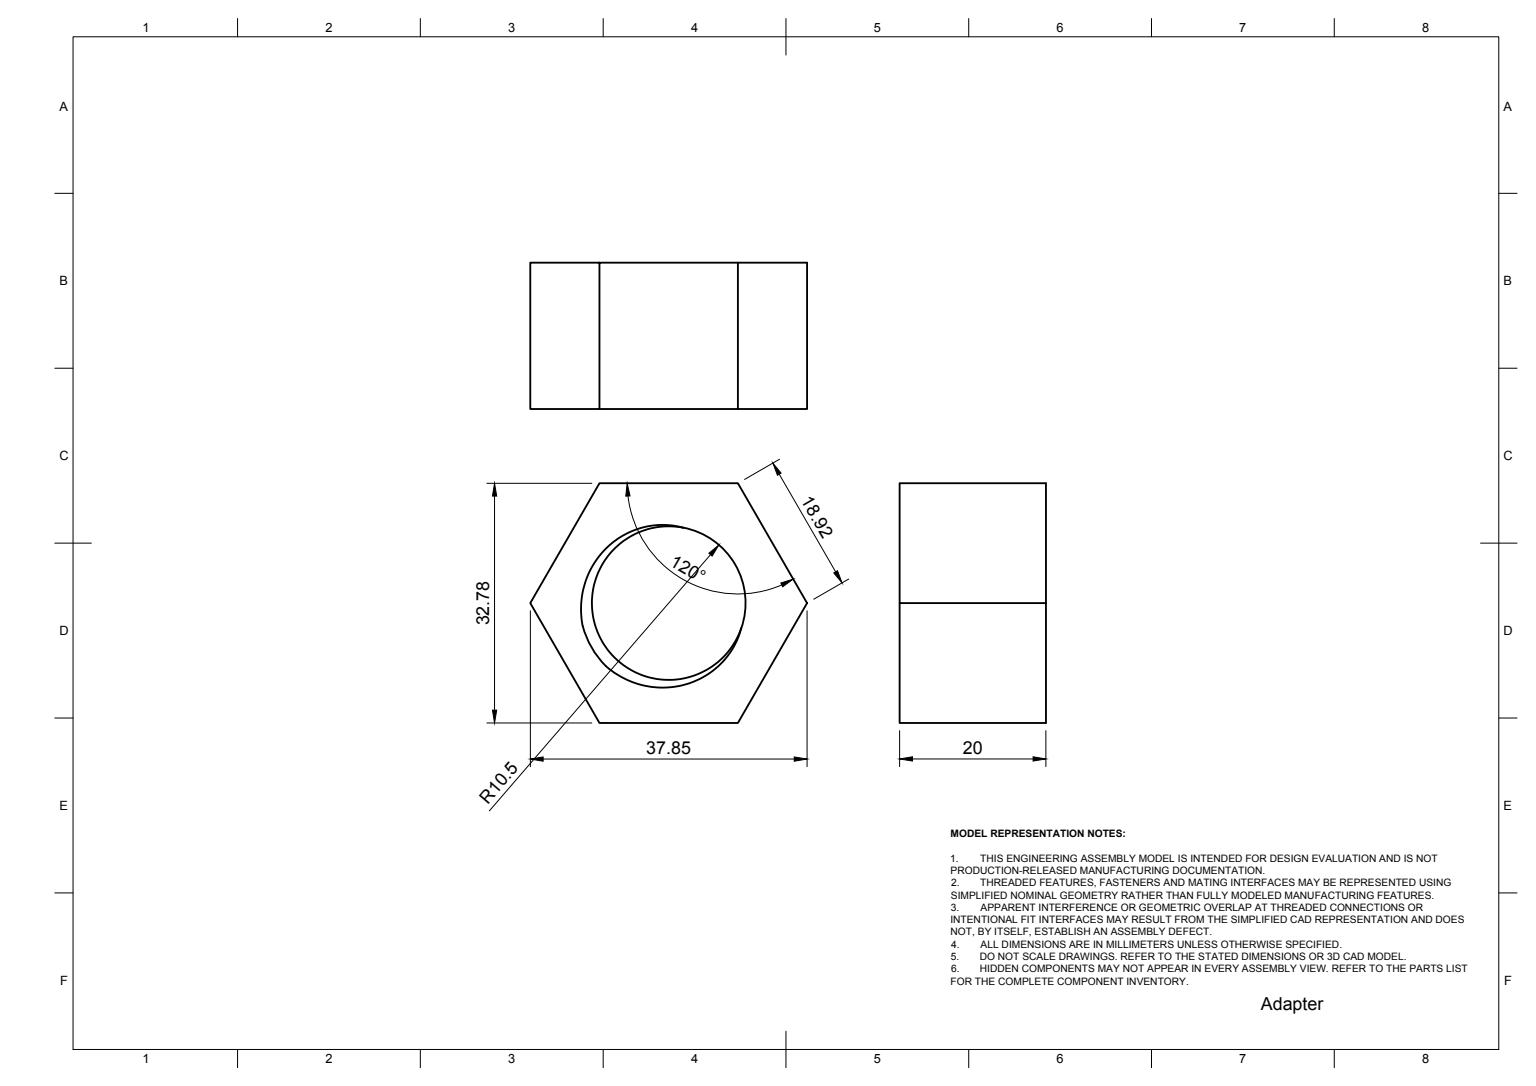
ISO-10303-21;
HEADER;
/* Generated by software containing ST-Developer
 * from STEP Tools, Inc. (www.steptools.com) 
 */

FILE_DESCRIPTION(
/* description */ (''),
/* implementation_level */ '2;1');

FILE_NAME(
/* name */ 'Adapter.step',
/* time_stamp */ '2026-10-06T12:47:13-07:00',
/* author */ (''),
/* organization */ (''),
/* preprocessor_version */ 'ST-DEVELOPER v20.2',
/* originating_system */ 'Autodesk Translation Framework v15.15.0.0',
/* authorisation */ '');

FILE_SCHEMA (('AUTOMOTIVE_DESIGN { 1 0 10303 214 3 1 1 }'));
ENDSEC;

DATA;
#10=MECHANICAL_DESIGN_GEOMETRIC_PRESENTATION_REPRESENTATION('',(#70),#42667);
#52=SHAPE_REPRESENTATION_RELATIONSHIP('SRR','None',#42705,#61);
#61=ADVANCED_BREP_SHAPE_REPRESENTATION('',(#79),#42661);
#70=STYLED_ITEM('',(#42756),#79);
#79=MANIFOLD_SOLID_BREP('Body1',#4035);
#86=B_SPLINE_SURFACE_WITH_KNOTS('',3,3,((#10429,#10430,#10431,#10432,#10433,
#10434,#10435,#10436,#10437,#10438,#10439,#10440,#10441,#10442,#10443,#10444,
#10445,#10446,#10447,#10448,#10449,#10450,#10451,#10452,#10453,#10454,#10455,
#10456,#10457,#10458,#10459,#10460,#10461,#10462,#10463,#10464,#10465,#10466,
#10467,#10468,#10469,#10470,#10471,#10472,#10473,#10474,#10475,#10476,#10477,
#10478,#10479,#10480,#10481,#10482,#10483,#10484,#10485,#10486,#10487,#10488,
#10489,#10490,#10491,#10492,#10493,#10494,#10495,#10496,#10497,#10498,#10499,
#10500,#10501,#10502,#10503,#10504,#10505,#10506,#10507,#10508,#10509,#10510,
#10511,#10512,#10513,#10514,#10515,#10516,#10517,#10518,#10519),(#10520,
#10521,#10522,#10523,#10524,#10525,#10526,#10527,#10528,#10529,#10530,#10531,
#10532,#10533,#10534,#10535,#10536,#10537,#10538,#10539,#10540,#10541,#10542,
#10543,#10544,#10545,#10546,#10547,#10548,#10549,#10550,#10551,#10552,#10553,
#10554,#10555,#10556,#10557,#10558,#10559,#10560,#10561,#10562,#10563,#10564,
#10565,#10566,#10567,#10568,#10569,#10570,#10571,#10572,#10573,#10574,#10575,
#10576,#10577,#10578,#10579,#10580,#10581,#10582,#10583,#10584,#10585,#10586,
#10587,#10588,#10589,#10590,#10591,#10592,#10593,#10594,#10595,#10596,#10597,
#10598,#10599,#10600,#10601,#10602,#10603,#10604,#10605,#10606,#10607,#10608,
#10609,#10610),(#10611,#10612,#10613,#10614,#10615,#10616,#10617,#10618,
#10619,#10620,#10621,#10622,#10623,#10624,#10625,#10626,#10627,#10628,#10629,
#10630,#10631,#10632,#10633,#10634,#10635,#10636,#10637,#10638,#10639,#10640,
#10641,#10642,#10643,#10644,#10645,#10646,#10647,#10648,#10649,#10650,#10651,
#10652,#10653,#10654,#10655,#10656,#10657,#10658,#10659,#10660,#10661,#10662,
#10663,#10664,#10665,#10666,#10667,#10668,#10669,#10670,#10671,#10672,#10673,
#10674,#10675,#10676,#10677,#10678,#10679,#10680,#10681,#10682,#10683,#10684,
#10685,#10686,#10687,#10688,#10689,#10690,#10691,#10692,#10693,#10694,#10695,
#10696,#10697,#10698,#10699,#10700,#10701),(#10702,#10703,#10704,#10705,
#10706,#10707,#10708,#10709,#10710,#10711,#10712,#10713,#10714,#10715,#10716,
#10717,#10718,#10719,#10720,#10721,#10722,#10723,#10724,#10725,#10726,#10727,
#10728,#10729,#10730,#10731,#10732,#10733,#10734,#10735,#10736,#10737,#10738,
#10739,#10740,#10741,#10742,#10743,#10744,#10745,#10746,#10747,#10748,#10749,
#10750,#10751,#10752,#10753,#10754,#10755,#10756,#10757,#10758,#10759,#10760,
#10761,#10762,#10763,#10764,#10765,#10766,#10767,#10768,#10769,#10770,#10771,
#10772,#10773,#10774,#10775,#10776,#10777,#10778,#10779,#10780,#10781,#10782,
#10783,#10784,#10785,#10786,#10787,#10788,#10789,#10790,#10791,#10792)),
 .UNSPECIFIED.,.F.,.F.,.F.,(4,4),(4,1,1,1,1,1,1,1,1,1,1,1,1,1,1,1,1,1,1,
1,1,1,1,1,1,1,1,1,1,1,1,1,1,1,1,1,1,1,1,1,1,1,1,1,1,1,1,1,1,1,1,1,1,1,1,
1,1,1,1,1,1,1,1,1,1,1,1,1,1,1,1,1,1,1,1,1,1,1,1,1,1,1,1,1,1,1,1,1,4),(-0.000129081019394602,
0.193330292353948),(11.8519068837255,12.3510302549558,12.8500245451668,
13.3490188353777,13.8480131255886,14.3470074157995,14.8460017060104,15.3449959962214,
15.8439902864323,16.3429845766432,16.8419788668541,17.3409731570651,17.839967447276,
18.3389617374869,18.8379560276978,19.3369503179088,19.8359446081197,20.3349388983306,
20.8339331885415,21.3329274787524,21.8319217689634,22.3309160591743,22.8299103493852,
23.3289046395961,23.8278989298071,24.326893220018,24.8258875102289,25.3248818004398,
25.8238760906508,26.3228703808617,26.8218646710726,27.3208589612835,27.8198532514944,
28.3188475417054,28.8178418319163,29.3168361221272,29.8158304123381,30.3148247025491,
30.81381899276,31.3128132829709,31.8118075731818,32.3108018633928,32.8097961536037,
33.3087904438146,33.8077847340255,34.3067790242364,34.8057733144474,35.3047676046583,
35.8037618948692,36.3027561850801,36.8017504752911,37.300744765502,37.7997390557129,
38.2987333459238,38.7977276361348,39.2967219263457,39.7957162165566,40.2947105067675,
40.7937047969784,41.2926990871894,41.7916933774003,42.2906876676112,42.7896819578221,
43.2886762480331,43.787670538244,44.2866648284549,44.7856591186658,45.2846534088767,
45.7836476990877,46.2826419892986,46.7816362795095,47.2806305697204,47.7796248599314,
48.2786191501423,48.7776134403532,49.2766077305641,49.7756020207751,50.274596310986,
50.7735906011969,51.2725848914078,51.7715791816187,52.2705734718297,52.7695677620406,
53.2685620522515,53.7675563424624,54.2665506326734,54.7655449228843,55.2645392130952,
55.7635335033061),.UNSPECIFIED.);
#87=B_SPLINE_SURFACE_WITH_KNOTS('',3,3,((#11034,#11035,#11036,#11037,#11038,
#11039,#11040,#11041,#11042,#11043,#11044,#11045,#11046,#11047,#11048,#11049,
#11050,#11051,#11052,#11053,#11054,#11055,#11056,#11057,#11058,#11059,#11060,
#11061,#11062,#11063,#11064,#11065,#11066,#11067,#11068,#11069,#11070,#11071,
#11072,#11073,#11074,#11075,#11076,#11077,#11078,#11079,#11080,#11081,#11082,
#11083,#11084,#11085,#11086,#11087,#11088,#11089,#11090,#11091,#11092,#11093,
#11094,#11095,#11096,#11097,#11098,#11099,#11100,#11101,#11102,#11103,#11104,
#11105,#11106,#11107,#11108,#11109,#11110,#11111,#11112,#11113,#11114,#11115,
#11116,#11117,#11118,#11119,#11120,#11121,#11122,#11123,#11124),(#11125,
#11126,#11127,#11128,#11129,#11130,#11131,#11132,#11133,#11134,#11135,#11136,
#11137,#11138,#11139,#11140,#11141,#11142,#11143,#11144,#11145,#11146,#11147,
#11148,#11149,#11150,#11151,#11152,#11153,#11154,#11155,#11156,#11157,#11158,
#11159,#11160,#11161,#11162,#11163,#11164,#11165,#11166,#11167,#11168,#11169,
#11170,#11171,#11172,#11173,#11174,#11175,#11176,#11177,#11178,#11179,#11180,
#11181,#11182,#11183,#11184,#11185,#11186,#11187,#11188,#11189,#11190,#11191,
#11192,#11193,#11194,#11195,#11196,#11197,#11198,#11199,#11200,#11201,#11202,
#11203,#11204,#11205,#11206,#11207,#11208,#11209,#11210,#11211,#11212,#11213,
#11214,#11215),(#11216,#11217,#11218,#11219,#11220,#11221,#11222,#11223,
#11224,#11225,#11226,#11227,#11228,#11229,#11230,#11231,#11232,#11233,#11234,
#11235,#11236,#11237,#11238,#11239,#11240,#11241,#11242,#11243,#11244,#11245,
#11246,#11247,#11248,#11249,#11250,#11251,#11252,#11253,#11254,#11255,#11256,
#11257,#11258,#11259,#11260,#11261,#11262,#11263,#11264,#11265,#11266,#11267,
#11268,#11269,#11270,#11271,#11272,#11273,#11274,#11275,#11276,#11277,#11278,
#11279,#11280,#11281,#11282,#11283,#11284,#11285,#11286,#11287,#11288,#11289,
#11290,#11291,#11292,#11293,#11294,#11295,#11296,#11297,#11298,#11299,#11300,
#11301,#11302,#11303,#11304,#11305,#11306),(#11307,#11308,#11309,#11310,
#11311,#11312,#11313,#11314,#11315,#11316,#11317,#11318,#11319,#11320,#11321,
#11322,#11323,#11324,#11325,#11326,#11327,#11328,#11329,#11330,#11331,#11332,
#11333,#11334,#11335,#11336,#11337,#11338,#11339,#11340,#11341,#11342,#11343,
#11344,#11345,#11346,#11347,#11348,#11349,#11350,#11351,#11352,#11353,#11354,
#11355,#11356,#11357,#11358,#11359,#11360,#11361,#11362,#11363,#11364,#11365,
#11366,#11367,#11368,#11369,#11370,#11371,#11372,#11373,#11374,#11375,#11376,
#11377,#11378,#11379,#11380,#11381,#11382,#11383,#11384,#11385,#11386,#11387,
#11388,#11389,#11390,#11391,#11392,#11393,#11394,#11395,#11396,#11397)),
 .UNSPECIFIED.,.F.,.F.,.F.,(4,4),(4,1,1,1,1,1,1,1,1,1,1,1,1,1,1,1,1,1,1,
1,1,1,1,1,1,1,1,1,1,1,1,1,1,1,1,1,1,1,1,1,1,1,1,1,1,1,1,1,1,1,1,1,1,1,1,
1,1,1,1,1,1,1,1,1,1,1,1,1,1,1,1,1,1,1,1,1,1,1,1,1,1,1,1,1,1,1,1,1,4),(-9.09719654654513E-5,
0.1933682374602),(14.3987024268659,14.8976967170768,15.3966910072877,15.8956852974986,
16.3946795877096,16.8936738779205,17.3926681681314,17.8916624583423,18.3906567485533,
18.8896510387642,19.3886453289751,19.887639619186,20.386633909397,20.8856281996079,
21.3846224898188,21.8836167800297,22.3826110702406,22.8816053604516,23.3805996506625,
23.8795939408734,24.3785882310843,24.8775825212953,25.3765768115062,25.8755711017171,
26.374565391928,26.8735596821389,27.3725539723499,27.8715482625608,28.3705425527717,
28.8695368429826,29.3685311331936,29.8675254234045,30.3665197136154,30.8655140038263,
31.3645082940373,31.8635025842482,32.3624968744591,32.86149116467,33.3604854548809,
33.8594797450919,34.3584740353028,34.8574683255137,35.3564626157246,35.8554569059356,
36.3544511961465,36.8534454863574,37.3524397765683,37.8514340667792,38.3504283569902,
38.8494226472011,39.348416937412,39.8474112276229,40.3464055178339,40.8453998080448,
41.3443940982557,41.8433883884666,42.3423826786776,42.8413769688885,43.3403712590994,
43.8393655493103,44.3383598395212,44.8373541297322,45.3363484199431,45.835342710154,
46.3343370003649,46.8333312905759,47.3323255807868,47.8313198709977,48.3303141612086,
48.8293084514195,49.3283027416305,49.8272970318414,50.3262913220523,50.8252856122632,
51.3242799024742,51.8232741926851,52.322268482896,52.8212627731069,53.3202570633179,
53.8192513535288,54.3182456437397,54.8172399339506,55.3162342241615,55.8152285143725,
56.3142228045834,56.8132170947943,57.3122113850052,57.8112056752162,58.3103290677895),
 .UNSPECIFIED.);
#100=B_SPLINE_CURVE_WITH_KNOTS('',3,(#5957,#5958,#5959,#5960,#5961,#5962,
#5963),.UNSPECIFIED.,.F.,.F.,(4,3,4),(13.8756314554422,13.9455249758043,
14.0061469241355),.UNSPECIFIED.);
#101=B_SPLINE_CURVE_WITH_KNOTS('',3,(#5970,#5971,#5972,#5973,#5974,#5975,
#5976,#5977,#5978,#5979,#5980,#5981,#5982,#5983,#5984,#5985,#5986,#5987,
#5988,#5989,#5990,#5991,#5992,#5993,#5994,#5995,#5996,#5997,#5998,#5999,
#6000,#6001,#6002,#6003,#6004,#6005,#6006,#6007,#6008,#6009,#6010,#6011,
#6012,#6013,#6014,#6015,#6016,#6017,#6018,#6019,#6020,#6021,#6022,#6023,
#6024,#6025,#6026,#6027,#6028,#6029,#6030,#6031,#6032,#6033,#6034,#6035,
#6036,#6037,#6038,#6039,#6040,#6041,#6042,#6043,#6044,#6045,#6046,#6047,
#6048,#6049,#6050,#6051,#6052,#6053,#6054,#6055,#6056,#6057,#6058,#6059,
#6060,#6061,#6062,#6063,#6064,#6065,#6066,#6067,#6068,#6069,#6070,#6071,
#6072,#6073,#6074,#6075,#6076,#6077,#6078,#6079,#6080,#6081,#6082,#6083,
#6084,#6085,#6086,#6087,#6088,#6089,#6090,#6091,#6092,#6093,#6094,#6095,
#6096,#6097,#6098,#6099,#6100,#6101,#6102,#6103,#6104,#6105,#6106,#6107,
#6108,#6109,#6110,#6111,#6112,#6113,#6114,#6115,#6116,#6117,#6118,#6119,
#6120,#6121,#6122,#6123,#6124,#6125,#6126,#6127,#6128,#6129,#6130,#6131,
#6132,#6133,#6134,#6135,#6136,#6137,#6138,#6139,#6140,#6141,#6142,#6143,
#6144,#6145,#6146,#6147,#6148,#6149,#6150,#6151,#6152,#6153,#6154,#6155,
#6156,#6157,#6158,#6159,#6160,#6161,#6162,#6163,#6164,#6165),
 .UNSPECIFIED.,.F.,.F.,(4,3,3,3,3,3,3,3,3,3,3,3,3,3,3,3,3,3,3,3,3,3,3,3,
3,3,3,3,3,3,3,3,3,3,3,3,3,3,3,3,3,3,3,3,3,3,3,3,3,3,3,3,3,3,3,3,3,3,3,3,
3,3,3,3,3,4),(15.7079632680278,15.781258546969,15.8439902864323,15.9140293859905,
15.9840565719878,16.0540759705774,16.1263031220939,16.1963262492752,16.2696554129592,
16.3429845766432,16.4130258394328,16.4830552130784,16.5530768178735,16.6253023301186,
16.6953276818739,16.768653274364,16.8419788668541,16.9120192399517,16.9820477145933,
17.0520684134795,17.1242945993759,17.1943190394544,17.2676460982597,17.3409731570651,
17.4110137716016,17.4810424897669,17.5510634336108,17.6232894370271,17.6933141225493,
17.7666407849127,17.839967447276,17.9100080714022,17.9800367996442,18.0500577540238,
18.1222837498896,18.192308446954,18.2656350922205,18.3389617374869,18.4090022932936,
18.4790309522726,18.5490518366316,18.6212778843981,18.6913025104407,18.7646292690693,
18.8379560276978,18.9079966408986,18.9780253579764,19.048046300983,19.1202723052145,
19.1902969905308,19.2636236542198,19.3369503179088,19.406990897852,19.47701958129,
19.5470404903645,19.6192665198033,19.6892911708882,19.762617889504,19.8359446081197,
19.9059847976786,19.9760129588395,20.0460332138481,20.1160559860082,20.1860772609487,
20.2561091917616,20.289300242169),.UNSPECIFIED.);
#102=B_SPLINE_CURVE_WITH_KNOTS('',3,(#6166,#6167,#6168,#6169,#6170,#6171,
#6172,#6173,#6174,#6175,#6176,#6177,#6178,#6179,#6180,#6181,#6182,#6183,
#6184,#6185,#6186,#6187,#6188,#6189,#6190,#6191,#6192,#6193,#6194,#6195,
#6196,#6197,#6198,#6199,#6200,#6201,#6202,#6203,#6204,#6205,#6206,#6207,
#6208,#6209,#6210,#6211,#6212,#6213,#6214,#6215,#6216,#6217,#6218,#6219,
#6220,#6221,#6222,#6223,#6224,#6225,#6226,#6227,#6228,#6229,#6230,#6231,
#6232,#6233,#6234,#6235,#6236,#6237,#6238,#6239,#6240,#6241),
 .UNSPECIFIED.,.F.,.F.,(4,3,3,3,3,3,3,3,3,3,3,3,3,3,3,3,3,3,3,3,3,3,3,3,
3,4),(14.0061469241355,14.076021357976,14.1459007978716,14.2157791918409,
14.2856739697488,14.3470074157995,14.4170482343003,14.4870771759581,14.5570983621866,
14.6293241981425,14.6993491698427,14.7726754379265,14.8460017060104,14.9160393182244,
14.9860649926552,15.0560828595175,15.1283111436935,15.198332708346,15.2716643522837,
15.3449959962214,15.4148686130277,15.488142276758,15.5579967616873,15.6278466788921,
15.697700868083,15.7079632679489),.UNSPECIFIED.);
#103=B_SPLINE_CURVE_WITH_KNOTS('',3,(#6245,#6246,#6247,#6248,#6249,#6250),
 .UNSPECIFIED.,.F.,.F.,(4,1,1,4),(14.3987024268659,14.8976967170768,15.3966910072877,
15.7079632679489),.UNSPECIFIED.);
#104=B_SPLINE_CURVE_WITH_KNOTS('',3,(#6251,#6252,#6253,#6254,#6255,#6256,
#6257,#6258,#6259,#6260,#6261,#6262,#6263),.UNSPECIFIED.,.F.,.F.,(4,1,1,
1,1,1,1,1,1,1,4),(15.7079632679489,15.8956852974986,16.3946795877096,16.8936738779205,
17.3926681681314,17.8916624583423,18.3906567485533,18.8896510387642,19.3886453289751,
19.887639619186,20.2892872762916),.UNSPECIFIED.);
#105=B_SPLINE_CURVE_WITH_KNOTS('',3,(#6269,#6270,#6271,#6272,#6273,#6274,
#6275,#6276,#6277,#6278,#6279,#6280,#6281,#6282,#6283,#6284,#6285,#6286,
#6287,#6288,#6289,#6290,#6291,#6292,#6293,#6294,#6295,#6296,#6297,#6298,
#6299,#6300,#6301,#6302,#6303,#6304,#6305,#6306,#6307,#6308,#6309,#6310,
#6311,#6312,#6313,#6314,#6315,#6316,#6317,#6318,#6319,#6320,#6321,#6322,
#6323,#6324,#6325,#6326,#6327,#6328,#6329,#6330,#6331,#6332,#6333,#6334,
#6335,#6336,#6337,#6338,#6339,#6340,#6341,#6342,#6343,#6344,#6345,#6346,
#6347,#6348,#6349,#6350,#6351,#6352,#6353,#6354,#6355,#6356,#6357,#6358,
#6359,#6360,#6361,#6362,#6363,#6364,#6365,#6366,#6367,#6368,#6369,#6370,
#6371,#6372,#6373,#6374,#6375,#6376,#6377,#6378,#6379,#6380,#6381,#6382,
#6383,#6384,#6385,#6386,#6387,#6388,#6389,#6390,#6391,#6392,#6393,#6394,
#6395,#6396,#6397,#6398,#6399,#6400,#6401,#6402,#6403,#6404,#6405,#6406,
#6407,#6408,#6409,#6410,#6411,#6412,#6413,#6414,#6415,#6416,#6417,#6418,
#6419,#6420,#6421,#6422,#6423,#6424,#6425,#6426,#6427,#6428,#6429,#6430,
#6431,#6432,#6433,#6434,#6435,#6436,#6437,#6438,#6439,#6440,#6441,#6442,
#6443,#6444,#6445,#6446,#6447,#6448,#6449,#6450,#6451,#6452,#6453,#6454,
#6455,#6456,#6457,#6458,#6459,#6460,#6461,#6462,#6463,#6464),
 .UNSPECIFIED.,.F.,.F.,(4,3,3,3,3,3,3,3,3,3,3,3,3,3,3,3,3,3,3,3,3,3,3,3,
3,3,3,3,3,3,3,3,3,3,3,3,3,3,3,3,3,3,3,3,3,3,3,3,3,3,3,3,3,3,3,3,3,3,3,3,
3,3,3,3,3,4),(21.9911485751285,22.0611187640108,22.1310953555668,22.2010715824223,
22.2710644969389,22.3309160591743,22.4009566501728,22.4709853447878,22.541006265131,
22.6132322861946,22.683256948635,22.7565836490101,22.8299103493852,22.8999509401425,
22.9699796345137,23.0400005546109,23.1122265758572,23.18225123805,23.2555779388231,
23.3289046395961,23.3989452304404,23.4689739248995,23.5389948450855,23.6112208662659,
23.6812455285474,23.7545722291773,23.8278989298071,23.8979395206352,23.9679682150779,
24.037989135248,24.1102151564405,24.1802398187058,24.2535665193619,24.326893220018,
24.3969338108387,24.4669625052738,24.5369834254368,24.6092094466348,24.6792341088923,
24.7525608095606,24.8258875102289,24.8959281010602,24.9659567955063,25.0359777156793,
25.1082037368695,25.1782283991379,25.2515550997889,25.3248818004398,25.3949223912636,
25.4649510857019,25.5349720058675,25.6071980270633,25.6772226893242,25.7505493899875,
25.8238760906508,25.8939166814786,25.9639453759211,26.0339662960901,26.106192317283,
26.1762169795476,26.2495436802046,26.3228703808617,26.392910974502,26.4629389186468,
26.5329614212261,26.5724975465912),.UNSPECIFIED.);
#106=B_SPLINE_CURVE_WITH_KNOTS('',3,(#6465,#6466,#6467,#6468,#6469,#6470,
#6471,#6472,#6473,#6474,#6475,#6476,#6477,#6478,#6479,#6480,#6481,#6482,
#6483,#6484,#6485,#6486,#6487,#6488,#6489,#6490,#6491,#6492,#6493,#6494,
#6495,#6496,#6497,#6498,#6499,#6500,#6501,#6502,#6503,#6504,#6505,#6506,
#6507,#6508,#6509,#6510,#6511,#6512,#6513,#6514,#6515,#6516,#6517,#6518,
#6519,#6520,#6521,#6522,#6523,#6524,#6525,#6526,#6527,#6528,#6529,#6530,
#6531,#6532,#6533,#6534,#6535,#6536,#6537,#6538,#6539,#6540),
 .UNSPECIFIED.,.F.,.F.,(4,3,3,3,3,3,3,3,3,3,3,3,3,3,3,3,3,3,3,3,3,3,3,3,
3,4),(20.289300242169,20.3349388983306,20.4049794883864,20.4750081820518,
20.5450291014412,20.6172551232163,20.6872797847037,20.7606064866226,20.8339331885415,
20.9039737790573,20.9740024731822,21.0440233930295,21.1162494144602,21.1862740763956,
21.259600777574,21.3329274787524,21.4029680700421,21.4729967649525,21.5430176855947,
21.6152437064369,21.6852683691804,21.7585950690719,21.8319217689634,21.9045986695098,
21.9772545252523,21.9911485750577),.UNSPECIFIED.);
#107=B_SPLINE_CURVE_WITH_KNOTS('',3,(#6542,#6543,#6544,#6545,#6546,#6547,
#6548,#6549),.UNSPECIFIED.,.F.,.F.,(4,1,1,1,1,4),(20.2892872762916,20.386633909397,
20.8856281996079,21.3846224898188,21.8836167800297,21.9911485751285),
 .UNSPECIFIED.);
#108=B_SPLINE_CURVE_WITH_KNOTS('',3,(#6550,#6551,#6552,#6553,#6554,#6555,
#6556,#6557,#6558,#6559,#6560,#6561,#6562,#6563,#6564,#6565,#6566,#6567,
#6568,#6569,#6570,#6571,#6572,#6573,#6574,#6575,#6576,#6577,#6578,#6579,
#6580,#6581,#6582,#6583,#6584,#6585,#6586,#6587,#6588,#6589,#6590,#6591,
#6592,#6593,#6594,#6595,#6596,#6597,#6598,#6599,#6600,#6601,#6602,#6603,
#6604,#6605,#6606,#6607,#6608,#6609,#6610,#6611,#6612,#6613,#6614,#6615,
#6616,#6617,#6618,#6619,#6620,#6621,#6622,#6623,#6624,#6625,#6626,#6627,
#6628,#6629,#6630,#6631,#6632,#6633,#6634,#6635,#6636,#6637,#6638,#6639,
#6640,#6641,#6642,#6643,#6644,#6645,#6646,#6647,#6648,#6649,#6650,#6651,
#6652,#6653,#6654,#6655,#6656,#6657,#6658,#6659,#6660,#6661,#6662,#6663,
#6664,#6665,#6666,#6667,#6668,#6669,#6670,#6671,#6672,#6673,#6674,#6675,
#6676,#6677,#6678,#6679,#6680,#6681,#6682,#6683,#6684,#6685,#6686,#6687,
#6688,#6689,#6690,#6691,#6692,#6693,#6694,#6695,#6696,#6697,#6698,#6699,
#6700,#6701,#6702,#6703,#6704,#6705,#6706,#6707,#6708,#6709,#6710,#6711,
#6712,#6713,#6714,#6715,#6716,#6717,#6718,#6719,#6720,#6721,#6722,#6723,
#6724,#6725,#6726,#6727,#6728,#6729,#6730,#6731,#6732,#6733,#6734,#6735,
#6736,#6737,#6738,#6739,#6740,#6741,#6742,#6743,#6744,#6745),
 .UNSPECIFIED.,.F.,.F.,(4,3,3,3,3,3,3,3,3,3,3,3,3,3,3,3,3,3,3,3,3,3,3,3,
3,3,3,3,3,3,3,3,3,3,3,3,3,3,3,3,3,3,3,3,3,3,3,3,3,3,3,3,3,3,3,3,3,3,3,3,
3,3,3,3,3,4),(21.9911485751285,22.0609174698852,22.1306788205048,22.2004452722809,
22.2702117236623,22.339993679049,22.3826110702406,22.4526516650052,22.522680363424,
22.5927012875987,22.6649273058119,22.7349519721031,22.8082786662773,22.8816053604516,
22.9516459505158,23.0216746441895,23.0916955635876,23.1639215853563,23.2339462468523,
23.3072729487574,23.3805996506625,23.4506402411789,23.5206689353043,23.5906898551522,
23.6629158765825,23.7329405385188,23.8062672396961,23.8795939408734,23.9496345321602,
24.0196632270677,24.0896841477066,24.1619101685511,24.2319348312914,24.3052615311878,
24.3785882310843,24.4486288215852,24.5186575156965,24.5886784355325,24.6609044569732,
24.7309291189009,24.8042558200981,24.8775825212953,24.9476231122925,25.0176518069063,
25.0876727272481,25.1598987483126,25.2299234107518,25.303250111129,25.3765768115062,
25.4466174022641,25.5166460966359,25.5866670167347,25.6588930379803,25.7289177001737,
25.8022444009454,25.8755711017171,25.9456116925611,26.0156403870198,26.0856613072057,
26.1578873283863,26.2279119906681,26.301238691298,26.374565391928,26.4446053180435,
26.5146354344288,26.5725063250621),.UNSPECIFIED.);
#109=B_SPLINE_CURVE_WITH_KNOTS('',3,(#6751,#6752,#6753,#6754,#6755,#6756,
#6757,#6758,#6759,#6760,#6761,#6762,#6763,#6764,#6765,#6766,#6767,#6768,
#6769,#6770,#6771,#6772,#6773,#6774,#6775,#6776,#6777,#6778,#6779,#6780,
#6781,#6782,#6783,#6784,#6785,#6786,#6787,#6788,#6789,#6790,#6791,#6792,
#6793,#6794,#6795,#6796,#6797,#6798,#6799,#6800,#6801,#6802,#6803,#6804,
#6805,#6806,#6807,#6808,#6809,#6810,#6811,#6812,#6813,#6814,#6815,#6816,
#6817,#6818,#6819,#6820,#6821,#6822,#6823,#6824,#6825,#6826,#6827,#6828,
#6829,#6830,#6831,#6832,#6833,#6834,#6835,#6836,#6837,#6838,#6839,#6840,
#6841,#6842,#6843,#6844,#6845,#6846,#6847,#6848,#6849,#6850,#6851,#6852,
#6853,#6854,#6855,#6856,#6857,#6858,#6859,#6860,#6861,#6862,#6863,#6864,
#6865,#6866,#6867,#6868,#6869,#6870,#6871,#6872,#6873,#6874,#6875,#6876,
#6877,#6878,#6879,#6880,#6881,#6882,#6883,#6884,#6885,#6886,#6887,#6888,
#6889,#6890,#6891,#6892,#6893,#6894,#6895,#6896,#6897,#6898,#6899,#6900,
#6901,#6902,#6903,#6904,#6905,#6906,#6907,#6908,#6909,#6910,#6911,#6912,
#6913,#6914,#6915,#6916,#6917,#6918,#6919,#6920,#6921,#6922,#6923,#6924,
#6925,#6926,#6927,#6928,#6929,#6930,#6931,#6932,#6933,#6934,#6935,#6936,
#6937,#6938,#6939,#6940,#6941,#6942,#6943,#6944,#6945,#6946),
 .UNSPECIFIED.,.F.,.F.,(4,3,3,3,3,3,3,3,3,3,3,3,3,3,3,3,3,3,3,3,3,3,3,3,
3,3,3,3,3,3,3,3,3,3,3,3,3,3,3,3,3,3,3,3,3,3,3,3,3,3,3,3,3,3,3,3,3,3,3,3,
3,3,3,3,3,4),(28.2743338823081,28.3188475417054,28.3888881325318,28.4589168269729,
28.5289377471412,28.601163768335,28.6711884305987,28.7445151312575,28.8178418319163,
28.8878824227428,28.9579111171838,29.0279320373515,29.1001580585454,29.170182720809,
29.2435094214681,29.3168361221272,29.3868767129537,29.4569054073949,29.526926327563,
29.5991523487568,29.6691770110205,29.7425037116793,29.8158304123381,29.8858710031646,
29.9558996976058,30.025920617774,30.0981466389678,30.1681713012315,30.2414980018903,
30.3148247025491,30.3848652933756,30.4548939878167,30.5249149079848,30.5971409291786,
30.6671655914423,30.7404922921012,30.81381899276,30.8838595835864,30.9538882780275,
31.0239091981955,31.0961352193893,31.166159881653,31.2394865823119,31.3128132829709,
31.3828538737974,31.4528825682385,31.5229034884066,31.5951295096004,31.6651541718641,
31.7384808725229,31.8118075731818,31.8818481640083,31.9518768584493,32.0218977786175,
32.0941237998113,32.164148462075,32.2374751627339,32.3108018633928,32.3808424542193,
32.4508711486604,32.5208920688285,32.5931180900223,32.6631427522859,32.7364694529448,
32.8097961536037,32.8556949433396),.UNSPECIFIED.);
#110=B_SPLINE_CURVE_WITH_KNOTS('',3,(#6947,#6948,#6949,#6950,#6951,#6952,
#6953,#6954,#6955,#6956,#6957,#6958,#6959,#6960,#6961,#6962,#6963,#6964,
#6965,#6966,#6967,#6968,#6969,#6970,#6971,#6972,#6973,#6974,#6975,#6976,
#6977,#6978,#6979,#6980,#6981,#6982,#6983,#6984,#6985,#6986,#6987,#6988,
#6989,#6990,#6991,#6992,#6993,#6994,#6995,#6996,#6997,#6998,#6999,#7000,
#7001,#7002,#7003,#7004,#7005,#7006,#7007,#7008,#7009,#7010,#7011,#7012,
#7013,#7014,#7015,#7016,#7017,#7018,#7019,#7020,#7021,#7022),
 .UNSPECIFIED.,.F.,.F.,(4,3,3,3,3,3,3,3,3,3,3,3,3,3,3,3,3,3,3,3,3,3,3,3,
3,4),(26.5724975465912,26.6425224627946,26.7125479358874,26.7825880206627,
26.8218646710726,26.8919052618991,26.9619339563403,27.0319548765084,27.1041808977022,
27.1742055599662,27.2475322606249,27.3208589612835,27.3908995521103,27.4609282465518,
27.5309491667197,27.6031751879134,27.6731998501771,27.7465265508357,27.8198532514944,
27.8896727070108,27.9594796023928,28.0292786272708,28.0990816217299,28.1688842155913,
28.238700456284,28.2743338822293),.UNSPECIFIED.);
#111=B_SPLINE_CURVE_WITH_KNOTS('',3,(#7024,#7025,#7026,#7027,#7028,#7029,
#7030,#7031,#7032,#7033,#7034,#7035,#7036,#7037,#7038,#7039,#7040,#7041,
#7042,#7043,#7044,#7045,#7046,#7047,#7048,#7049,#7050,#7051,#7052,#7053,
#7054,#7055,#7056,#7057,#7058,#7059,#7060,#7061,#7062,#7063,#7064,#7065,
#7066,#7067,#7068,#7069,#7070,#7071,#7072,#7073,#7074,#7075,#7076,#7077,
#7078,#7079,#7080,#7081,#7082,#7083,#7084,#7085,#7086,#7087,#7088,#7089,
#7090,#7091,#7092,#7093,#7094,#7095,#7096,#7097,#7098,#7099),
 .UNSPECIFIED.,.F.,.F.,(4,3,3,3,3,3,3,3,3,3,3,3,3,3,3,3,3,3,3,3,3,3,3,3,
3,4),(26.5725063250621,26.6425239289077,26.7125485918865,26.7825748927809,
26.8526147955675,26.8735596821389,26.9436002729595,27.0136289673943,27.0836498875562,
27.1558759087546,27.2259005710118,27.2992272716809,27.3725539723499,27.4425945631809,
27.5126232576271,27.5826441778001,27.6548701989903,27.7248948612584,27.7982215619096,
27.8715482625608,27.9413131725913,28.0110652143382,28.0808150034561,28.1505602216933,
28.2203156472821,28.2743338822406),.UNSPECIFIED.);
#112=B_SPLINE_CURVE_WITH_KNOTS('',3,(#7100,#7101,#7102,#7103,#7104,#7105,
#7106,#7107,#7108,#7109,#7110,#7111,#7112,#7113,#7114,#7115,#7116,#7117,
#7118,#7119,#7120,#7121,#7122,#7123,#7124,#7125,#7126,#7127,#7128,#7129,
#7130,#7131,#7132,#7133,#7134,#7135,#7136,#7137,#7138,#7139,#7140,#7141,
#7142,#7143,#7144,#7145,#7146,#7147,#7148,#7149,#7150,#7151,#7152,#7153,
#7154,#7155,#7156,#7157,#7158,#7159,#7160,#7161,#7162,#7163,#7164,#7165,
#7166,#7167,#7168,#7169,#7170,#7171,#7172,#7173,#7174,#7175,#7176,#7177,
#7178,#7179,#7180,#7181,#7182,#7183,#7184,#7185,#7186,#7187,#7188,#7189,
#7190,#7191,#7192,#7193,#7194,#7195,#7196,#7197,#7198,#7199,#7200,#7201,
#7202,#7203,#7204,#7205,#7206,#7207,#7208,#7209,#7210,#7211,#7212,#7213,
#7214,#7215,#7216,#7217,#7218,#7219,#7220,#7221,#7222,#7223,#7224,#7225,
#7226,#7227,#7228,#7229,#7230,#7231,#7232,#7233,#7234,#7235,#7236,#7237,
#7238,#7239,#7240,#7241,#7242,#7243,#7244,#7245,#7246,#7247,#7248,#7249,
#7250,#7251,#7252,#7253,#7254,#7255,#7256,#7257,#7258,#7259,#7260,#7261,
#7262,#7263,#7264,#7265,#7266,#7267,#7268,#7269,#7270,#7271,#7272,#7273,
#7274,#7275,#7276,#7277,#7278,#7279,#7280,#7281,#7282,#7283,#7284,#7285,
#7286,#7287,#7288,#7289,#7290,#7291,#7292,#7293,#7294,#7295),
 .UNSPECIFIED.,.F.,.F.,(4,3,3,3,3,3,3,3,3,3,3,3,3,3,3,3,3,3,3,3,3,3,3,3,
3,3,3,3,3,3,3,3,3,3,3,3,3,3,3,3,3,3,3,3,3,3,3,3,3,3,3,3,3,3,3,3,3,3,3,3,
3,3,3,3,3,4),(28.2743338823081,28.3488858316158,28.3705425527717,28.4405831435994,
28.5106118380417,28.5806327582111,28.652858779404,28.7228834416689,28.7962101423258,
28.8695368429826,28.9395774338088,29.0096061282494,29.0796270484171,29.1518530696112,
29.2218777318745,29.295204432534,29.3685311331936,29.4385717240202,29.5086004184613,
29.5786213386295,29.6508473598232,29.7208720220869,29.7941987227457,29.8675254234045,
29.937566014231,30.0075947086721,30.0776156288402,30.149841650034,30.2198663122976,
30.2931930129565,30.3665197136154,30.4365603044418,30.5065889988829,30.576609919051,
30.6488359402448,30.7188606025084,30.7921873031673,30.8655140038263,30.9355545946528,
31.005583289094,31.0756042092621,31.1478302304559,31.2178548927196,31.2911815933785,
31.3645082940373,31.4345488848638,31.5045775793049,31.574598499473,31.6468245206668,
31.7168491829305,31.7901758835893,31.8635025842482,31.9335431750747,32.0035718695158,
32.0735927896838,32.1458188108776,32.2158434731413,32.2891701738002,32.3624968744591,
32.4325374038997,32.5025660201463,32.5725868453283,32.643360355704,32.7133845410207,
32.7845327139258,32.8556808868309),.UNSPECIFIED.);
#113=B_SPLINE_CURVE_WITH_KNOTS('',3,(#7301,#7302,#7303,#7304,#7305,#7306,
#7307,#7308,#7309,#7310,#7311,#7312,#7313),.UNSPECIFIED.,.F.,.F.,(4,1,1,
1,1,1,1,1,1,1,4),(34.5575191894877,34.8057733144474,35.3047676046583,35.8037618948692,
36.3027561850801,36.8017504752911,37.300744765502,37.7997390557129,38.2987333459238,
38.7977276361348,39.138844988577),.UNSPECIFIED.);
#114=B_SPLINE_CURVE_WITH_KNOTS('',3,(#7314,#7315,#7316,#7317,#7318,#7319,
#7320,#7321,#7322,#7323,#7324,#7325,#7326,#7327,#7328,#7329,#7330,#7331,
#7332,#7333,#7334,#7335,#7336,#7337,#7338,#7339,#7340,#7341,#7342,#7343,
#7344,#7345,#7346,#7347,#7348,#7349,#7350,#7351,#7352,#7353,#7354,#7355,
#7356,#7357,#7358,#7359,#7360,#7361,#7362,#7363,#7364,#7365,#7366,#7367,
#7368,#7369,#7370,#7371,#7372,#7373,#7374,#7375,#7376,#7377,#7378,#7379,
#7380,#7381,#7382,#7383,#7384,#7385,#7386,#7387,#7388,#7389),
 .UNSPECIFIED.,.F.,.F.,(4,3,3,3,3,3,3,3,3,3,3,3,3,3,3,3,3,3,3,3,3,3,3,3,
3,4),(32.8556949433396,32.9257272727589,32.9957504074315,33.0657684672156,
33.1357932637452,33.205818991343,33.2758589616207,33.3087904438146,33.378831034641,
33.4488597290822,33.5188806492501,33.591106670444,33.6611313327076,33.7344580333666,
33.8077847340255,33.877825324852,33.9478540192931,34.0178749394612,34.090100960655,
34.1601256229187,34.2334523235775,34.3067790242364,34.3776775785114,34.4485623759747,
34.5194352520091,34.5575191894138),.UNSPECIFIED.);
#115=B_SPLINE_CURVE_WITH_KNOTS('',3,(#7391,#7392,#7393,#7394,#7395,#7396,
#7397,#7398,#7399,#7400,#7401,#7402,#7403,#7404,#7405,#7406,#7407,#7408,
#7409,#7410,#7411,#7412,#7413,#7414,#7415,#7416,#7417,#7418,#7419,#7420,
#7421,#7422,#7423,#7424,#7425,#7426,#7427,#7428,#7429,#7430,#7431,#7432,
#7433,#7434,#7435,#7436,#7437,#7438,#7439,#7440,#7441,#7442,#7443,#7444,
#7445,#7446,#7447,#7448,#7449,#7450,#7451,#7452,#7453,#7454,#7455,#7456,
#7457,#7458,#7459,#7460,#7461,#7462,#7463,#7464,#7465,#7466),
 .UNSPECIFIED.,.F.,.F.,(4,3,3,3,3,3,3,3,3,3,3,3,3,3,3,3,3,3,3,3,3,3,3,3,
3,4),(32.8556808868309,32.86149116467,32.9315317554965,33.0015604499375,
33.0715813701057,33.1438073912995,33.2138320535632,33.2871587542221,33.3604854548809,
33.4305260457074,33.5005547401485,33.5705756603166,33.6428016815104,33.712826343774,
33.786153044433,33.8594797450919,33.9295203359184,33.9995490303595,34.0695699505274,
34.1417959717213,34.211820633985,34.2851473346439,34.3584740353028,34.4302564390369,
34.5020210945599,34.557519189415),.UNSPECIFIED.);
#116=B_SPLINE_CURVE_WITH_KNOTS('',3,(#7467,#7468,#7469,#7470,#7471,#7472,
#7473,#7474,#7475,#7476,#7477,#7478,#7479,#7480,#7481,#7482,#7483,#7484,
#7485,#7486,#7487,#7488,#7489,#7490,#7491,#7492,#7493,#7494,#7495,#7496,
#7497,#7498,#7499,#7500,#7501,#7502,#7503,#7504,#7505,#7506,#7507,#7508,
#7509,#7510,#7511,#7512,#7513,#7514,#7515,#7516,#7517,#7518,#7519,#7520,
#7521,#7522,#7523,#7524,#7525,#7526,#7527,#7528,#7529,#7530,#7531,#7532,
#7533,#7534,#7535,#7536,#7537,#7538,#7539,#7540,#7541,#7542,#7543,#7544,
#7545,#7546,#7547,#7548,#7549,#7550,#7551,#7552,#7553,#7554,#7555,#7556,
#7557,#7558,#7559,#7560,#7561,#7562,#7563,#7564,#7565,#7566,#7567,#7568,
#7569,#7570,#7571,#7572,#7573,#7574,#7575,#7576,#7577,#7578,#7579,#7580,
#7581,#7582,#7583,#7584,#7585,#7586,#7587,#7588,#7589,#7590,#7591,#7592,
#7593,#7594,#7595,#7596,#7597,#7598,#7599,#7600,#7601,#7602,#7603,#7604,
#7605,#7606,#7607,#7608,#7609,#7610,#7611,#7612,#7613,#7614,#7615,#7616,
#7617,#7618,#7619,#7620,#7621,#7622,#7623,#7624,#7625,#7626,#7627,#7628,
#7629,#7630,#7631,#7632,#7633,#7634,#7635,#7636,#7637,#7638,#7639,#7640,
#7641,#7642,#7643,#7644,#7645,#7646,#7647,#7648,#7649,#7650,#7651,#7652,
#7653,#7654,#7655,#7656,#7657,#7658,#7659,#7660,#7661,#7662),
 .UNSPECIFIED.,.F.,.F.,(4,3,3,3,3,3,3,3,3,3,3,3,3,3,3,3,3,3,3,3,3,3,3,3,
3,3,3,3,3,3,3,3,3,3,3,3,3,3,3,3,3,3,3,3,3,3,3,3,3,3,3,3,3,3,3,3,3,3,3,3,
3,3,3,3,3,4),(34.5575191894877,34.6277996055737,34.6980904637057,34.7683845128919,
34.8386929125139,34.8574683255137,34.9275089163402,34.9975376107813,35.0675585309494,
35.1397845521432,35.2098092144068,35.2831359150657,35.3564626157246,35.4265032065511,
35.4965319009923,35.5665528211606,35.6387788423543,35.7088035046181,35.7821302052769,
35.8554569059356,35.9254974967621,35.9955261912033,36.0655471113711,36.137773132565,
36.2077977948286,36.2811244954875,36.3544511961465,36.424491786973,36.4945204814141,
36.5645414015817,36.6367674227756,36.7067920850394,36.7801187856984,36.8534454863574,
36.9234860771838,36.9935147716249,37.0635356917926,37.1357617129865,37.2057863752504,
37.2791130759094,37.3524397765683,37.4224803673948,37.4925090618357,37.5625299820039,
37.6347560031977,37.7047806654614,37.7781073661203,37.8514340667792,37.9214746576057,
37.9915033520468,38.0615242722151,38.1337502934089,38.2037749556726,38.2771016563314,
38.3504283569902,38.4204689478168,38.4904976422578,38.5605185624258,38.6327445836196,
38.702769245883,38.776095946542,38.8494226472011,38.9217823054225,38.9918107826881,
39.0653360313874,39.1388612800867),.UNSPECIFIED.);
#117=B_SPLINE_CURVE_WITH_KNOTS('',3,(#7668,#7669,#7670,#7671,#7672,#7673,
#7674,#7675,#7676,#7677,#7678,#7679,#7680,#7681,#7682,#7683,#7684,#7685,
#7686,#7687,#7688,#7689,#7690,#7691,#7692,#7693,#7694,#7695,#7696,#7697,
#7698,#7699,#7700,#7701,#7702,#7703,#7704,#7705,#7706,#7707,#7708,#7709,
#7710,#7711,#7712,#7713,#7714,#7715,#7716,#7717,#7718,#7719,#7720,#7721,
#7722,#7723,#7724,#7725,#7726,#7727,#7728,#7729,#7730,#7731,#7732,#7733,
#7734,#7735,#7736,#7737,#7738,#7739,#7740,#7741,#7742,#7743,#7744,#7745,
#7746,#7747,#7748,#7749,#7750,#7751,#7752,#7753,#7754,#7755,#7756,#7757,
#7758,#7759,#7760,#7761,#7762,#7763,#7764,#7765,#7766,#7767,#7768,#7769,
#7770,#7771,#7772,#7773,#7774,#7775,#7776,#7777,#7778,#7779,#7780,#7781,
#7782,#7783,#7784,#7785,#7786,#7787,#7788,#7789,#7790,#7791,#7792,#7793,
#7794,#7795,#7796,#7797,#7798,#7799,#7800,#7801,#7802,#7803,#7804,#7805,
#7806,#7807,#7808,#7809,#7810,#7811,#7812,#7813,#7814,#7815,#7816,#7817,
#7818,#7819,#7820,#7821,#7822,#7823,#7824,#7825,#7826,#7827,#7828,#7829,
#7830,#7831,#7832,#7833,#7834,#7835,#7836,#7837,#7838,#7839,#7840,#7841,
#7842,#7843,#7844,#7845,#7846,#7847,#7848,#7849,#7850,#7851,#7852,#7853,
#7854,#7855,#7856,#7857,#7858,#7859,#7860,#7861,#7862,#7863),
 .UNSPECIFIED.,.F.,.F.,(4,3,3,3,3,3,3,3,3,3,3,3,3,3,3,3,3,3,3,3,3,3,3,3,
3,3,3,3,3,3,3,3,3,3,3,3,3,3,3,3,3,3,3,3,3,3,3,3,3,3,3,3,3,3,3,3,3,3,3,3,
3,3,3,3,3,4),(40.8407044966673,40.910513107026,40.9803103162599,41.050100831576,
41.1198969722149,41.1896937756429,41.2595054868552,41.2926990871894,41.3627396780171,
41.4327683724595,41.5027892926283,41.5750153138213,41.645039976086,41.7183666767432,
41.7916933774003,41.861733968224,41.9317626626622,42.0017835828273,42.0740096040233,
42.1440342662842,42.2173609669477,42.2906876676112,42.3607282584425,42.4307569528887,
42.5007778730621,42.5730038942521,42.6430285565208,42.7163552571714,42.7896819578221,
42.8597225486426,42.9297512430777,42.9997721632399,43.0719981844382,43.1420228466959,
43.2153495473645,43.2886762480331,43.3587168388615,43.4287455333043,43.4987664534742,
43.5709924746666,43.641017136932,43.714343837588,43.787670538244,43.8577111290883,
43.9277398235473,43.9977607437335,44.0699867649139,44.1400114271953,44.2133381278251,
44.2866648284549,44.356705419211,44.426734113581,44.4967550336782,44.5689810549251,
44.6390057171185,44.7123324178922,44.7856591186658,44.8556997096685,44.9257284042865,
44.9957493246311,45.0679753456925,45.1380000081308,45.2113267085037,45.2846534088767,
45.3546946558375,45.4220693616144),.UNSPECIFIED.);
#118=B_SPLINE_CURVE_WITH_KNOTS('',3,(#7864,#7865,#7866,#7867,#7868,#7869,
#7870,#7871),.UNSPECIFIED.,.F.,.F.,(4,1,1,1,1,4),(39.138844988577,39.2967219263457,
39.7957162165566,40.2947105067675,40.7937047969784,40.8407044966673),
 .UNSPECIFIED.);
#119=B_SPLINE_CURVE_WITH_KNOTS('',3,(#7873,#7874,#7875,#7876,#7877,#7878,
#7879,#7880,#7881,#7882,#7883,#7884,#7885,#7886,#7887,#7888,#7889,#7890,
#7891,#7892,#7893,#7894,#7895,#7896,#7897,#7898,#7899,#7900,#7901,#7902,
#7903,#7904,#7905,#7906,#7907,#7908,#7909,#7910,#7911,#7912,#7913,#7914,
#7915,#7916,#7917,#7918,#7919,#7920,#7921,#7922,#7923,#7924,#7925,#7926,
#7927,#7928,#7929,#7930,#7931,#7932,#7933,#7934,#7935,#7936,#7937,#7938,
#7939,#7940,#7941,#7942,#7943,#7944,#7945),.UNSPECIFIED.,.F.,.F.,(4,3,3,
3,3,3,3,3,3,3,3,3,3,3,3,3,3,3,3,3,3,3,3,3,4),(39.1388612800867,39.2088860064159,
39.2789273844965,39.348416937412,39.4184575282385,39.4884862226791,39.5585071428482,
39.6307331640419,39.7007578263056,39.7740845269643,39.8474112276229,39.9174518184494,
39.9874805128906,40.0575014330589,40.1297274542526,40.1997521165164,40.2730788171751,
40.3464055178339,40.4164150422325,40.4864125754172,40.5564023218123,40.6274778655123,
40.6974714282655,40.7690879624389,40.8407044966123),.UNSPECIFIED.);
#120=B_SPLINE_CURVE_WITH_KNOTS('',3,(#7946,#7947,#7948,#7949,#7950,#7951,
#7952,#7953,#7954,#7955,#7956,#7957,#7958,#7959,#7960,#7961,#7962,#7963,
#7964,#7965,#7966,#7967,#7968,#7969,#7970,#7971,#7972,#7973,#7974,#7975,
#7976,#7977,#7978,#7979,#7980,#7981,#7982,#7983,#7984,#7985,#7986,#7987,
#7988,#7989,#7990,#7991,#7992,#7993,#7994,#7995,#7996,#7997,#7998,#7999,
#8000,#8001,#8002,#8003,#8004,#8005,#8006,#8007,#8008,#8009,#8010,#8011,
#8012,#8013,#8014,#8015,#8016,#8017,#8018,#8019,#8020,#8021,#8022,#8023,
#8024,#8025,#8026,#8027,#8028,#8029,#8030,#8031,#8032,#8033,#8034,#8035,
#8036,#8037,#8038,#8039,#8040,#8041,#8042,#8043,#8044,#8045,#8046,#8047,
#8048,#8049,#8050,#8051,#8052,#8053,#8054,#8055,#8056,#8057,#8058,#8059,
#8060,#8061,#8062,#8063,#8064,#8065,#8066,#8067,#8068,#8069,#8070,#8071,
#8072,#8073,#8074,#8075,#8076,#8077,#8078,#8079,#8080,#8081,#8082,#8083,
#8084,#8085,#8086,#8087,#8088,#8089,#8090,#8091,#8092,#8093,#8094,#8095,
#8096,#8097,#8098,#8099,#8100,#8101,#8102,#8103,#8104,#8105,#8106,#8107,
#8108,#8109,#8110,#8111,#8112,#8113,#8114,#8115,#8116,#8117,#8118,#8119,
#8120,#8121,#8122,#8123,#8124,#8125,#8126,#8127,#8128,#8129,#8130,#8131,
#8132,#8133,#8134,#8135,#8136,#8137,#8138,#8139,#8140,#8141,#8142,#8143,
#8144),.UNSPECIFIED.,.F.,.F.,(4,3,3,3,3,3,3,3,3,3,3,3,3,3,3,3,3,3,3,3,3,
3,3,3,3,3,3,3,3,3,3,3,3,3,3,3,3,3,3,3,3,3,3,3,3,3,3,3,3,3,3,3,3,3,3,3,3,
3,3,3,3,3,3,3,3,3,4),(40.8407044966673,40.8453998080448,40.9154403988712,
40.9854690933122,41.0554900134805,41.1277160346743,41.1977406969378,41.2710673975968,
41.3443940982557,41.4144346890823,41.4844633835235,41.5544843036917,41.6267103248854,
41.6967349871492,41.7700616878079,41.8433883884666,41.913428979293,41.9834576737341,
42.0534785939022,42.1257046150961,42.1957292773597,42.2690559780186,42.3423826786776,
42.4124232695042,42.4824519639455,42.5524728841137,42.6246989053074,42.6947235675711,
42.7680502682298,42.8413769688885,42.911417559715,42.9814462541562,43.0514671743242,
43.123693195518,43.1937178577816,43.2670445584405,43.3403712590994,43.4104118499255,
43.4804405443662,43.550461464534,43.6226874857281,43.6927121479913,43.7660388486508,
43.8393655493103,43.909406140138,43.9794348345803,44.0494557547496,44.1216817759425,
44.1917064382073,44.2650331388643,44.3383598395212,44.408400430345,44.4784291247834,
44.5484500449487,44.6206760661446,44.6907007284056,44.7640274290689,44.8373541297322,
44.9073947205635,44.9774234150094,45.0474443351823,45.1196703563725,45.189695018641,
45.263021719292,45.3363484199431,45.4063883545637,45.4220700257397),
 .UNSPECIFIED.);
#121=B_SPLINE_CURVE_WITH_KNOTS('',3,(#8150,#8151,#8152,#8153,#8154,#8155,
#8156,#8157,#8158,#8159,#8160,#8161,#8162,#8163,#8164,#8165,#8166,#8167,
#8168,#8169,#8170,#8171,#8172,#8173,#8174,#8175,#8176,#8177,#8178,#8179,
#8180,#8181,#8182,#8183,#8184,#8185,#8186,#8187,#8188,#8189,#8190,#8191,
#8192,#8193,#8194,#8195,#8196,#8197,#8198,#8199,#8200,#8201,#8202,#8203,
#8204,#8205,#8206,#8207,#8208,#8209,#8210,#8211,#8212,#8213,#8214,#8215,
#8216,#8217,#8218,#8219,#8220,#8221,#8222,#8223,#8224,#8225,#8226,#8227,
#8228,#8229,#8230,#8231,#8232,#8233,#8234,#8235,#8236,#8237,#8238,#8239,
#8240,#8241,#8242,#8243,#8244,#8245,#8246,#8247,#8248,#8249,#8250,#8251,
#8252,#8253,#8254,#8255,#8256,#8257,#8258,#8259,#8260,#8261,#8262,#8263,
#8264,#8265,#8266,#8267,#8268,#8269,#8270,#8271,#8272,#8273,#8274,#8275,
#8276,#8277,#8278,#8279,#8280,#8281,#8282,#8283,#8284,#8285,#8286,#8287,
#8288,#8289,#8290,#8291,#8292,#8293,#8294,#8295,#8296,#8297,#8298,#8299,
#8300,#8301,#8302,#8303,#8304,#8305,#8306,#8307,#8308,#8309,#8310,#8311,
#8312,#8313,#8314,#8315,#8316,#8317,#8318,#8319,#8320,#8321,#8322,#8323,
#8324,#8325,#8326,#8327,#8328,#8329,#8330,#8331,#8332,#8333,#8334,#8335,
#8336,#8337,#8338,#8339,#8340,#8341,#8342,#8343,#8344,#8345,#8346,#8347,
#8348),.UNSPECIFIED.,.F.,.F.,(4,3,3,3,3,3,3,3,3,3,3,3,3,3,3,3,3,3,3,3,3,
3,3,3,3,3,3,3,3,3,3,3,3,3,3,3,3,3,3,3,3,3,3,3,3,3,3,3,3,3,3,3,3,3,3,3,3,
3,3,3,3,3,3,3,3,3,4),(47.1238898039153,47.1966069931218,47.269346291875,
47.2806305697204,47.3506711645816,47.4206998630754,47.4907207873035,47.5629468054605,
47.6329714717519,47.7062981658417,47.7796248599314,47.8496654396268,47.919694122898,
47.9897150318869,48.0619410614508,48.1319657126511,48.2052924313967,48.2786191501423,
48.3486597639494,48.4186884814349,48.4887094246505,48.5609354285762,48.6309601136108,
48.704286776982,48.7776134403532,48.8476539950211,48.9176826532346,48.987703537201,
49.0599295855418,49.1299542121136,49.2032809713389,49.2766077305641,49.3466483562613,
49.4166770855596,49.486698040481,49.5589240355545,49.6289487318888,49.702275376332,
49.7756020207751,49.8456426343618,49.9156713518887,49.9856922954051,50.0579182993003,
50.1279429852639,50.201269648125,50.274596310986,50.3446366811021,50.4146651537395,
50.4846858515977,50.5569120389975,50.6269364804616,50.7002635408293,50.7735906011969,
50.8436318783237,50.9136612616073,50.9836828713458,51.0559083763613,51.1259337214531,
51.1992593064304,51.2725848914078,51.3426234218437,51.4126498588465,51.4857933163341,
51.5558129797052,51.6258314628023,51.695858176314,51.705223688797),
 .UNSPECIFIED.);
#122=B_SPLINE_CURVE_WITH_KNOTS('',3,(#8349,#8350,#8351,#8352,#8353,#8354,
#8355,#8356,#8357,#8358,#8359,#8360,#8361,#8362,#8363,#8364,#8365,#8366,
#8367,#8368,#8369,#8370,#8371,#8372,#8373,#8374,#8375,#8376,#8377,#8378,
#8379,#8380,#8381,#8382,#8383,#8384,#8385,#8386,#8387,#8388,#8389,#8390,
#8391,#8392,#8393,#8394,#8395,#8396,#8397,#8398,#8399,#8400,#8401,#8402,
#8403,#8404,#8405,#8406,#8407,#8408,#8409,#8410,#8411,#8412,#8413,#8414,
#8415,#8416,#8417,#8418,#8419,#8420,#8421,#8422,#8423,#8424),
 .UNSPECIFIED.,.F.,.F.,(4,3,3,3,3,3,3,3,3,3,3,3,3,3,3,3,3,3,3,3,3,3,3,3,
3,4),(45.4220693616144,45.4920905009292,45.5649798004688,45.6350044521349,
45.7050314710928,45.7750715078873,45.7836476990877,45.8536882903937,45.9237169853146,
45.9937379059628,46.0659639267968,46.1359885895327,46.2093152894156,46.2826419892986,
46.3526825797948,46.4227112739064,46.4927321937468,46.5649582151875,46.6349828771319,
46.7083095783207,46.7816362795095,46.8516132827516,46.9215804164053,46.9915381364908,
47.0614983061719,47.1238898038469),.UNSPECIFIED.);
#123=B_SPLINE_CURVE_WITH_KNOTS('',3,(#8426,#8427,#8428,#8429,#8430,#8431,
#8432,#8433,#8434,#8435,#8436,#8437,#8438,#8439,#8440,#8441,#8442,#8443,
#8444,#8445,#8446,#8447,#8448,#8449,#8450,#8451,#8452,#8453,#8454,#8455,
#8456,#8457,#8458,#8459,#8460,#8461,#8462,#8463,#8464,#8465,#8466,#8467,
#8468,#8469,#8470,#8471,#8472,#8473,#8474,#8475,#8476,#8477,#8478,#8479,
#8480,#8481,#8482,#8483,#8484,#8485,#8486,#8487,#8488,#8489,#8490,#8491,
#8492,#8493,#8494,#8495,#8496,#8497,#8498),.UNSPECIFIED.,.F.,.F.,(4,3,3,
3,3,3,3,3,3,3,3,3,3,3,3,3,3,3,3,3,3,3,3,3,4),(45.4220700257397,45.492096621416,
45.562116365311,45.6321420349469,45.7021668544972,45.7722078578491,45.835342710154,
45.9053833009824,45.9754119954253,46.045432915595,46.1176589367875,46.1876835990528,
46.2610102997088,46.3343370003649,46.4043775912091,46.4744062856679,46.544427205854,
46.6166532270345,46.6866778893158,46.7600045899459,46.8333312905759,46.9059709188937,
46.9763616597276,47.0501257317873,47.1238898038469),.UNSPECIFIED.);
#124=B_SPLINE_CURVE_WITH_KNOTS('',3,(#8499,#8500,#8501,#8502,#8503,#8504,
#8505,#8506,#8507,#8508,#8509,#8510,#8511,#8512,#8513,#8514,#8515,#8516,
#8517,#8518,#8519,#8520,#8521,#8522,#8523,#8524,#8525,#8526,#8527,#8528,
#8529,#8530,#8531,#8532,#8533,#8534,#8535,#8536,#8537,#8538,#8539,#8540,
#8541,#8542,#8543,#8544,#8545,#8546,#8547,#8548,#8549,#8550,#8551,#8552,
#8553,#8554,#8555,#8556,#8557,#8558,#8559,#8560,#8561,#8562,#8563,#8564,
#8565,#8566,#8567,#8568,#8569,#8570,#8571,#8572,#8573,#8574,#8575,#8576,
#8577,#8578,#8579,#8580,#8581,#8582,#8583,#8584,#8585,#8586,#8587,#8588,
#8589,#8590,#8591,#8592,#8593,#8594,#8595,#8596,#8597,#8598,#8599,#8600,
#8601,#8602,#8603,#8604,#8605,#8606,#8607,#8608,#8609,#8610,#8611,#8612,
#8613,#8614,#8615,#8616,#8617,#8618,#8619,#8620,#8621,#8622,#8623,#8624,
#8625,#8626,#8627,#8628,#8629,#8630,#8631,#8632,#8633,#8634,#8635,#8636,
#8637,#8638,#8639,#8640,#8641,#8642,#8643,#8644,#8645,#8646,#8647,#8648,
#8649,#8650,#8651,#8652,#8653,#8654,#8655,#8656,#8657,#8658,#8659,#8660,
#8661,#8662,#8663,#8664,#8665,#8666,#8667,#8668,#8669,#8670,#8671,#8672,
#8673,#8674,#8675,#8676,#8677,#8678,#8679,#8680,#8681,#8682,#8683,#8684,
#8685,#8686,#8687,#8688,#8689,#8690,#8691,#8692,#8693,#8694),
 .UNSPECIFIED.,.F.,.F.,(4,3,3,3,3,3,3,3,3,3,3,3,3,3,3,3,3,3,3,3,3,3,3,3,
3,3,3,3,3,3,3,3,3,3,3,3,3,3,3,3,3,3,3,3,3,3,3,3,3,3,3,3,3,3,3,3,3,3,3,3,
3,3,3,3,3,4),(47.1238898039108,47.1954657532806,47.2670653523193,47.3323255807868,
47.4023661717881,47.4723948664045,47.5424157867478,47.6146418078103,47.6846664702475,
47.7579931706226,47.8313198709977,47.9013604614893,47.9713891555945,48.0414100754268,
48.1136360968722,48.1836607588042,48.2569874600064,48.3303141612086,48.4003547525115,
48.4703834474297,48.5404043680745,48.6126303889108,48.6826550516439,48.7559817515317,
48.8293084514195,48.8993490419166,48.9693777360291,49.0393986558705,49.1116246773105,
49.1816493392556,49.2549760404431,49.3283027416305,49.3983433316981,49.4683720253742,
49.5383929447734,49.6106189665404,49.6806436280347,49.753970329938,49.8272970318414,
49.8973376266718,49.9673663251347,50.0373872493318,50.1096132675119,50.1796379337725,
50.2529646279124,50.3262913220523,50.3963319018199,50.4663605851638,50.5363814942255,
50.6086075237349,50.678632175007,50.7519588936351,50.8252856122632,50.8953262259418,
50.9653549432983,51.0353758863851,51.1076018904074,51.1776265753145,51.2509532388944,
51.3242799024742,51.3943197709416,51.4643474012373,51.5343709622389,51.6043893378668,
51.6744125951888,51.7052219494017),.UNSPECIFIED.);
#125=B_SPLINE_CURVE_WITH_KNOTS('',3,(#8700,#8701,#8702,#8703),
 .UNSPECIFIED.,.F.,.F.,(4,4),(7.59244615558812,7.94961020078307),
 .UNSPECIFIED.);
#126=B_SPLINE_CURVE_WITH_KNOTS('',3,(#8705,#8706,#8707,#8708,#8709,#8710,
#8711,#8712,#8713,#8714,#8715,#8716,#8717,#8718,#8719,#8720,#8721,#8722,
#8723,#8724,#8725,#8726,#8727,#8728,#8729,#8730,#8731,#8732,#8733,#8734,
#8735,#8736,#8737,#8738,#8739,#8740,#8741,#8742,#8743,#8744,#8745,#8746,
#8747,#8748,#8749,#8750,#8751,#8752,#8753,#8754,#8755,#8756,#8757,#8758,
#8759,#8760,#8761,#8762,#8763,#8764,#8765,#8766,#8767,#8768,#8769,#8770,
#8771,#8772,#8773,#8774,#8775,#8776,#8777,#8778,#8779,#8780,#8781,#8782,
#8783,#8784,#8785,#8786,#8787,#8788,#8789,#8790,#8791,#8792,#8793,#8794,
#8795,#8796,#8797,#8798,#8799,#8800,#8801,#8802,#8803,#8804,#8805,#8806,
#8807,#8808,#8809,#8810,#8811,#8812,#8813,#8814,#8815,#8816,#8817,#8818,
#8819,#8820,#8821,#8822,#8823,#8824,#8825,#8826,#8827,#8828,#8829,#8830,
#8831,#8832,#8833,#8834,#8835,#8836,#8837,#8838,#8839,#8840,#8841,#8842,
#8843,#8844,#8845,#8846,#8847,#8848,#8849,#8850,#8851,#8852,#8853,#8854,
#8855,#8856,#8857,#8858,#8859,#8860,#8861,#8862,#8863,#8864,#8865,#8866,
#8867,#8868,#8869,#8870,#8871,#8872,#8873,#8874,#8875,#8876,#8877,#8878,
#8879,#8880,#8881,#8882,#8883,#8884,#8885,#8886,#8887,#8888,#8889,#8890,
#8891,#8892,#8893,#8894,#8895,#8896,#8897,#8898,#8899,#8900,#8901,#8902,
#8903,#8904,#8905,#8906,#8907,#8908,#8909,#8910,#8911,#8912,#8913,#8914,
#8915,#8916,#8917,#8918,#8919,#8920,#8921,#8922,#8923,#8924,#8925,#8926,
#8927,#8928,#8929,#8930,#8931,#8932,#8933,#8934,#8935,#8936,#8937,#8938,
#8939,#8940,#8941,#8942),.UNSPECIFIED.,.F.,.F.,(4,3,3,3,3,3,3,3,3,3,3,3,
3,3,3,3,3,3,3,3,3,3,3,3,3,3,3,3,3,3,3,3,3,3,3,3,3,3,3,3,3,3,3,3,3,3,3,3,
3,3,3,3,3,3,3,3,3,3,3,3,3,3,3,3,3,3,3,3,3,3,3,3,3,3,3,3,3,3,3,4),(2.02359556728784,
2.09612063785746,2.16863302303831,2.24113775293914,2.31364811582229,2.38615861296181,
2.45868474905377,2.49497145105461,2.56765002727523,2.64031589890252,2.71297367059207,
2.78563719645063,2.85829941345175,2.93097867400525,2.99396574126554,3.06664098081929,
3.13930345029594,3.21195776421116,3.28461777093719,3.35727644001194,3.42995213051997,
3.49296003147646,3.56564099670242,3.63830926977429,3.71096944845288,3.78363537238572,
3.85629997895852,3.92898159803042,3.99195432168738,4.06463110674485,4.13729514772769,
4.20995105460737,4.28261267608536,4.35527296959601,4.42795028890615,4.49094861189831,
4.56362763260635,4.63629393530697,4.70895212345169,4.78161603998939,4.85427863280186,
4.92695824199939,4.98994290210923,5.06262100423254,5.1352863784211,5.20794363080207,
5.28060660711106,5.35326825861507,5.42594693144099,5.48893719232016,5.56161554328838,
5.63428116853687,5.70693867347046,5.77960190281452,5.85226380724567,5.92494273101668,
5.98793148253108,6.06060984370026,6.13327547967456,6.20593299582697,6.27859623707525,
6.35125815377287,6.42393709031945,6.486925772742,6.55960406326347,6.63226962758147,
6.70492707127597,6.77759023934746,6.85025208257815,6.92293094570417,6.98592006295293,
7.05859841273454,7.13126403706467,7.20392154135016,7.27658477047137,7.3492466749157,
7.42192559908852,7.48491435316385,7.56187309461106,7.59244614826265),
 .UNSPECIFIED.);
#127=B_SPLINE_CURVE_WITH_KNOTS('',3,(#8945,#8946,#8947,#8948,#8949,#8950,
#8951,#8952,#8953,#8954,#8955,#8956,#8957,#8958,#8959,#8960,#8961,#8962,
#8963,#8964,#8965,#8966,#8967,#8968,#8969,#8970,#8971,#8972,#8973,#8974,
#8975,#8976,#8977,#8978,#8979,#8980,#8981,#8982,#8983,#8984,#8985,#8986,
#8987,#8988,#8989,#8990,#8991,#8992,#8993,#8994,#8995,#8996,#8997,#8998,
#8999,#9000,#9001,#9002,#9003,#9004,#9005,#9006,#9007,#9008,#9009,#9010,
#9011,#9012,#9013,#9014),.UNSPECIFIED.,.F.,.F.,(4,2,2,2,2,2,2,2,2,2,2,2,
2,2,2,2,2,2,2,2,2,2,2,2,2,2,2,2,2,2,2,2,2,2,4),(0.000135688236192026,0.182534690442223,
0.329186859064794,0.430874046907693,0.509112081933848,0.621923710755093,
0.759294802457872,0.927030288955933,1.02288050568415,1.13549080719406,1.27678418460036,
1.46799932847935,1.55466406176925,1.66507905500832,1.80304759971923,1.99678085625352,
2.0809754199086,2.18736690979933,2.32733794325047,2.51744206634343,2.60414998945933,
2.71106797400003,2.85081076527383,3.0461407368146,3.13059907723473,3.24204658312837,
3.38004050519128,3.55146567007771,3.64685346840213,3.75941222161808,3.89978325985654,
4.0956229489707,4.18023039862239,4.29380952169095,4.43103355894701),
 .UNSPECIFIED.);
#128=B_SPLINE_CURVE_WITH_KNOTS('',3,(#9020,#9021,#9022,#9023,#9024,#9025,
#9026,#9027,#9028,#9029),.UNSPECIFIED.,.F.,.F.,(4,2,2,2,4),(12.8422919822627,
12.887154762158,13.0258167989269,13.1186138717486,13.2178341603313),
 .UNSPECIFIED.);
#129=B_SPLINE_CURVE_WITH_KNOTS('',3,(#9030,#9031,#9032,#9033,#9034,#9035,
#9036,#9037,#9038,#9039,#9040,#9041,#9042,#9043,#9044,#9045),
 .UNSPECIFIED.,.F.,.F.,(4,1,1,1,1,1,1,1,1,1,1,1,1,4),(7.94961020078307,
7.98390864337477,8.48290293358569,8.98189722379661,9.48089151400754,9.97988580421846,
10.4788800944294,10.9778743846403,11.4768686748512,11.9758629650621,12.4748572552731,
12.973851545484,13.4728458356949,13.8756314554422),.UNSPECIFIED.);
#130=B_SPLINE_CURVE_WITH_KNOTS('',3,(#9046,#9047,#9048,#9049,#9050,#9051,
#9052,#9053,#9054,#9055,#9056,#9057,#9058,#9059,#9060,#9061,#9062,#9063,
#9064,#9065,#9066,#9067,#9068,#9069,#9070,#9071,#9072,#9073,#9074,#9075,
#9076,#9077,#9078,#9079,#9080,#9081,#9082,#9083,#9084,#9085,#9086,#9087,
#9088,#9089,#9090,#9091,#9092,#9093,#9094,#9095,#9096,#9097,#9098,#9099,
#9100,#9101,#9102,#9103,#9104,#9105,#9106,#9107,#9108,#9109,#9110,#9111,
#9112,#9113,#9114,#9115,#9116,#9117,#9118,#9119,#9120,#9121,#9122,#9123,
#9124,#9125,#9126,#9127,#9128,#9129,#9130,#9131,#9132,#9133,#9134,#9135,
#9136,#9137,#9138,#9139,#9140,#9141,#9142,#9143,#9144,#9145),
 .UNSPECIFIED.,.F.,.F.,(4,2,2,2,2,2,2,2,2,2,2,2,2,2,2,2,2,2,2,2,2,2,2,2,
2,2,2,2,2,2,2,2,2,2,2,2,2,2,2,2,2,2,2,2,2,2,2,2,2,4),(4.43103355894701,
4.43112108136264,4.5974129920961,4.6949760496939,4.80225796218608,4.94513629188488,
5.14304951890869,5.22888262205294,5.33530324797899,5.47522895906651,5.67102573081961,
5.75521840543593,5.85791461303463,5.99864276279524,6.19466351084876,6.27953142305181,
6.39127651196381,6.52922847922396,6.70026604013396,6.79590080792733,6.97576906914361,
7.1369089391772,7.32967716260638,7.44353181543372,7.58080169596608,7.74761716210148,
7.84478550698122,7.95299010726183,8.09543431525411,8.29292072871432,8.37862309065676,
8.48559834856376,8.6253332273617,8.80539149015593,8.8980055317184,9.07507730815184,
9.23653588492767,9.42891091322493,9.53717879929051,9.67641954779035,9.85634273166462,
9.94846876501138,10.124371807052,10.2862506150661,10.4786886768751,10.585108936019,
10.7250936259518,10.9209686902655,11.0051861291791,11.0413371089366),
 .UNSPECIFIED.);
#131=B_SPLINE_CURVE_WITH_KNOTS('',3,(#9150,#9151,#9152,#9153,#9154,#9155,
#9156,#9157,#9158,#9159,#9160,#9161,#9162,#9163,#9164,#9165,#9166,#9167,
#9168,#9169,#9170,#9171,#9172,#9173,#9174,#9175,#9176,#9177,#9178,#9179,
#9180,#9181,#9182,#9183,#9184,#9185,#9186,#9187,#9188,#9189,#9190,#9191,
#9192,#9193,#9194,#9195,#9196,#9197,#9198,#9199,#9200,#9201,#9202,#9203,
#9204,#9205,#9206,#9207,#9208,#9209,#9210,#9211,#9212,#9213,#9214,#9215,
#9216,#9217,#9218,#9219,#9220,#9221,#9222,#9223,#9224,#9225,#9226,#9227,
#9228,#9229,#9230,#9231,#9232,#9233,#9234,#9235,#9236,#9237,#9238,#9239,
#9240,#9241,#9242,#9243,#9244,#9245,#9246,#9247,#9248,#9249,#9250,#9251),
 .UNSPECIFIED.,.F.,.F.,(4,2,2,2,2,2,2,2,2,2,2,2,2,2,2,2,2,2,2,2,2,2,2,2,
2,2,2,2,2,2,2,2,2,2,2,2,2,2,2,2,2,2,2,2,2,2,2,2,2,2,4),(6.23335612761586,
6.2680726661503,6.44942264436023,6.60915211923207,6.76136559666284,6.84923300983916,
6.95045580235986,7.11269571489834,7.25090846445631,7.36192407750934,7.44688581082496,
7.64297223261621,7.78383654572914,7.88624389570455,7.97052662126554,8.16631202122395,
8.30633596179256,8.41253308698677,8.4983811778714,8.69627543731715,8.83915310298785,
8.94644447739489,9.04402311820006,9.21031149618558,9.34765752913951,9.46120630502673,
9.54583931617467,9.74166539339258,9.8820615547246,9.9945325293888,10.0897943123272,
10.2615588379134,10.399560401475,10.5111028004756,10.5959745858038,10.7919542465067,
10.9326770564329,11.0353378666286,11.2280111432196,11.3887279582758,11.5692870436916,
11.6648159305064,11.8359091402827,11.9738179216995,12.0855833718003,12.1704159141617,
12.3663497119896,12.5070126022303,12.6105784668576,12.695645656318,12.8422919822627),
 .UNSPECIFIED.);
#132=B_SPLINE_CURVE_WITH_KNOTS('',3,(#9252,#9253,#9254,#9255,#9256,#9257,
#9258,#9259,#9260,#9261,#9262,#9263,#9264,#9265,#9266,#9267,#9268,#9269,
#9270,#9271,#9272,#9273,#9274,#9275,#9276,#9277,#9278,#9279,#9280,#9281,
#9282,#9283,#9284,#9285,#9286,#9287,#9288,#9289,#9290,#9291,#9292,#9293,
#9294,#9295,#9296,#9297,#9298,#9299,#9300,#9301,#9302,#9303,#9304,#9305,
#9306,#9307,#9308,#9309,#9310,#9311,#9312,#9313,#9314,#9315,#9316,#9317,
#9318,#9319,#9320,#9321,#9322,#9323,#9324,#9325,#9326,#9327,#9328,#9329,
#9330,#9331,#9332,#9333,#9334,#9335,#9336,#9337,#9338,#9339,#9340,#9341,
#9342,#9343,#9344,#9345,#9346,#9347),.UNSPECIFIED.,.F.,.F.,(4,2,2,2,2,2,
2,2,2,2,2,2,2,2,2,2,2,2,2,2,2,2,2,2,2,2,2,2,2,2,2,2,2,2,2,2,2,2,2,2,2,2,
2,2,2,2,2,4),(11.0413371089366,11.1079687724179,11.2487172487334,11.4447819529984,
11.5296659966344,11.6414732350562,11.7794588126016,11.9506203229406,12.0462296440394,
12.226700548978,12.3876027102809,12.5801555071267,12.6942822091242,12.8315199327858,
12.9987910833866,13.0956430068284,13.2046843234955,13.3467852356924,13.5439569316993,
13.6295371093675,13.7372405177515,13.8767441274198,14.0567961574491,14.1491616376219,
14.3256279190537,14.4873651427831,14.6798877932856,14.787419457666,14.9270028333426,
15.1070873787722,15.1995282230915,15.3761715394229,15.5378626266959,15.7303489097924,
15.8379211901484,15.9775009910812,16.1575942573031,16.2500284409572,16.4266528536513,
16.5883656734284,16.7808760392524,16.8884584809964,17.0280466873063,17.2081519258478,
17.3005913133539,17.4772251458276,17.6389498989778,17.6543409950681),
 .UNSPECIFIED.);
#133=B_SPLINE_CURVE_WITH_KNOTS('',3,(#9353,#9354,#9355,#9356,#9357,#9358),
 .UNSPECIFIED.,.F.,.F.,(4,2,4),(12.8423781512227,12.9895144519815,13.2181607322366),
 .UNSPECIFIED.);
#134=B_SPLINE_CURVE_WITH_KNOTS('',3,(#9359,#9360,#9361,#9362,#9363,#9364,
#9365,#9366,#9367,#9368,#9369,#9370,#9371,#9372,#9373,#9374,#9375,#9376,
#9377,#9378,#9379,#9380,#9381,#9382,#9383,#9384,#9385,#9386,#9387,#9388,
#9389,#9390,#9391,#9392,#9393,#9394,#9395,#9396,#9397,#9398,#9399,#9400,
#9401,#9402,#9403,#9404,#9405,#9406,#9407,#9408,#9409,#9410,#9411,#9412,
#9413,#9414,#9415,#9416,#9417,#9418,#9419,#9420,#9421,#9422,#9423,#9424,
#9425,#9426,#9427,#9428,#9429,#9430,#9431,#9432,#9433,#9434,#9435,#9436,
#9437,#9438,#9439,#9440,#9441,#9442,#9443,#9444,#9445,#9446,#9447,#9448),
 .UNSPECIFIED.,.F.,.F.,(4,2,2,2,2,2,2,2,2,2,2,2,2,2,2,2,2,2,2,2,2,2,2,2,
2,2,2,2,2,2,2,2,2,2,2,2,2,2,2,2,2,2,2,2,4),(0.000192812523341109,0.227830918649042,
0.402695824517761,0.495345820468585,0.605011255121174,0.745682846989847,
0.941635256368896,1.02647350321401,1.13818028830822,1.27609592000783,1.44708043233579,
1.54269318764458,1.72249229572632,1.88359776728222,2.07669827020567,2.17942746011534,
2.32010735870701,2.51607560838843,2.60091849941476,2.71266275449528,2.8505826010169,
3.02164223123286,3.11721781087632,3.29748494778651,3.45836804138001,3.65087443006171,
3.76478362635717,3.90200434301853,4.06891694069374,4.16595768138673,4.27438799083112,
4.416686309398,4.61401881184024,4.69966105666755,4.80681895602313,4.94644760489433,
5.12645933890658,5.21897313800511,5.39581519676004,5.55731223059382,5.74983419995918,
5.85878400080293,5.99773397831681,6.17448435879023,6.23335612761586),
 .UNSPECIFIED.);
#135=B_SPLINE_CURVE_WITH_KNOTS('',3,(#9449,#9450,#9451,#9452,#9453,#9454,
#9455,#9456,#9457,#9458,#9459,#9460,#9461,#9462,#9463,#9464,#9465,#9466,
#9467,#9468,#9469,#9470,#9471,#9472,#9473,#9474,#9475,#9476,#9477,#9478,
#9479,#9480,#9481,#9482,#9483,#9484,#9485,#9486,#9487,#9488,#9489,#9490,
#9491,#9492,#9493,#9494,#9495,#9496,#9497,#9498,#9499,#9500,#9501,#9502,
#9503,#9504,#9505,#9506,#9507,#9508,#9509,#9510,#9511,#9512,#9513,#9514,
#9515,#9516,#9517,#9518,#9519,#9520,#9521,#9522,#9523,#9524,#9525,#9526,
#9527,#9528,#9529,#9530,#9531,#9532,#9533,#9534,#9535,#9536,#9537,#9538,
#9539,#9540,#9541,#9542,#9543,#9544),.UNSPECIFIED.,.F.,.F.,(4,2,2,2,2,2,
2,2,2,2,2,2,2,2,2,2,2,2,2,2,2,2,2,2,2,2,2,2,2,2,2,2,2,2,2,2,2,2,2,2,2,2,
2,2,2,2,2,4),(17.6543409950681,17.831448232565,17.9388970388975,18.078550307813,
18.2580275286684,18.3509018576439,18.5285655816919,18.6899522360199,18.883317496408,
18.9859410358361,19.1268498083911,19.3230657959226,19.4080515417586,19.5194700182778,
19.6576752470134,19.8301085240745,19.925273452302,20.0382668814786,20.1785995356747,
20.3745754313835,20.4591193113276,20.560959448406,20.7022315358752,20.8987111478103,
20.9839122498395,21.0939464152428,21.2326549062009,21.4123366353141,21.5039831339058,
21.6859652182246,21.8449450631771,22.0389207324904,22.1618875308622,22.352077762761,
22.492416404637,22.6054578212541,22.7006149626931,22.8731170251549,23.0113543915084,
23.1227549816257,23.2077525682346,23.4039738361564,23.5449009423806,23.6475443397645,
23.8402633557091,24.0010308597138,24.1820036907275,24.2697619665442),
 .UNSPECIFIED.);
#136=B_SPLINE_CURVE_WITH_KNOTS('',3,(#9549,#9550,#9551,#9552,#9553,#9554,
#9555,#9556,#9557,#9558,#9559,#9560,#9561,#9562,#9563,#9564,#9565,#9566,
#9567,#9568,#9569,#9570,#9571,#9572,#9573,#9574,#9575,#9576,#9577,#9578,
#9579,#9580,#9581,#9582,#9583,#9584,#9585,#9586,#9587,#9588,#9589,#9590,
#9591,#9592,#9593,#9594,#9595,#9596,#9597,#9598,#9599,#9600,#9601,#9602,
#9603,#9604,#9605,#9606,#9607,#9608,#9609,#9610,#9611,#9612,#9613,#9614,
#9615,#9616,#9617,#9618,#9619,#9620,#9621,#9622,#9623,#9624,#9625,#9626,
#9627,#9628,#9629,#9630,#9631,#9632,#9633,#9634,#9635,#9636,#9637,#9638,
#9639,#9640,#9641,#9642,#9643,#9644,#9645,#9646,#9647,#9648,#9649,#9650),
 .UNSPECIFIED.,.F.,.F.,(4,2,2,2,2,2,2,2,2,2,2,2,2,2,2,2,2,2,2,2,2,2,2,2,
2,2,2,2,2,2,2,2,2,2,2,2,2,2,2,2,2,2,2,2,2,2,2,2,2,2,4),(6.23337760445098,
6.26077836375648,6.36024771798476,6.46448343304622,6.60906386766685,6.78456179187364,
6.93662045763576,7.1323810286063,7.30321529556475,7.45656361674879,7.53958466179243,
7.73647663198394,7.87584064015966,7.98371163899557,8.06920767247095,8.2661630472445,
8.40808467559384,8.51733631274462,8.61403729468532,8.78135200164673,8.91851068914279,
9.03266254477226,9.11723416458245,9.3130398364756,9.45336262315145,9.56600363361281,
9.66119059252339,9.83316651194362,9.97120439935581,10.0826538815603,10.1675408239304,
10.3635373773577,10.5042835130592,10.6069015054932,10.7997225471817,10.9605892203953,
11.1408781760215,11.2364444175853,11.4074977978003,11.545416911005,11.6571650160255,
11.742002359112,11.9379433516568,12.0786137180603,12.1827271699913,12.2684323702091,
12.4659165898637,12.6083986443827,12.7163747934482,12.813552790721,12.8423781512227),
 .UNSPECIFIED.);
#137=B_SPLINE_CURVE_WITH_KNOTS('',3,(#9651,#9652,#9653,#9654,#9655,#9656,
#9657,#9658,#9659,#9660,#9661,#9662,#9663,#9664,#9665,#9666,#9667,#9668,
#9669,#9670,#9671,#9672,#9673,#9674,#9675,#9676,#9677,#9678,#9679,#9680,
#9681,#9682,#9683,#9684,#9685,#9686,#9687,#9688,#9689,#9690,#9691,#9692,
#9693,#9694,#9695,#9696,#9697,#9698,#9699,#9700,#9701,#9702,#9703,#9704,
#9705,#9706,#9707,#9708,#9709,#9710,#9711,#9712,#9713,#9714,#9715,#9716,
#9717,#9718,#9719,#9720,#9721,#9722,#9723,#9724,#9725,#9726,#9727,#9728,
#9729,#9730,#9731,#9732,#9733,#9734,#9735,#9736,#9737,#9738,#9739,#9740,
#9741,#9742,#9743,#9744,#9745,#9746,#9747,#9748,#9749,#9750),
 .UNSPECIFIED.,.F.,.F.,(4,2,2,2,2,2,2,2,2,2,2,2,2,2,2,2,2,2,2,2,2,2,2,2,
2,2,2,2,2,2,2,2,2,2,2,2,2,2,2,2,2,2,2,2,2,2,2,2,2,4),(24.2697619665442,
24.2775981868636,24.4489178802201,24.5869659818761,24.6988703740305,24.7837903210938,
24.9799298746111,25.1207383490778,25.2327027835779,25.3283426169409,25.4995888239524,
25.6376391981639,25.7495081133103,25.8344271986969,26.0305591071743,26.1713654429127,
26.2755865933713,26.3613764208643,26.5590561568995,26.7016799031348,26.8097776151025,
26.907082060738,27.0739033264763,27.2112791614196,27.325154142349,27.5182505086529,
27.6797073494656,27.8571147537519,27.9498752178987,28.1297026103414,28.269443400461,
28.376645608559,28.4623502090655,28.6598040912766,28.8022060851135,28.9107074268383,
29.0078121207644,29.1748316803279,29.3121502107654,29.4261396767462,29.6186715357246,
29.7795702717774,29.9601421331204,30.0557572846878,30.2269559593022,30.3649693430795,
30.4768074783437,30.5617037610844,30.7577828820173,30.8837752445267),
 .UNSPECIFIED.);
#138=B_SPLINE_CURVE_WITH_KNOTS('',3,(#9756,#9757,#9758,#9759,#9760,#9761,
#9762,#9763,#9764,#9765,#9766,#9767,#9768,#9769,#9770,#9771),
 .UNSPECIFIED.,.F.,.F.,(4,3,3,3,3,4),(39.0083726877398,39.080749342486,
39.1531225734978,39.2254897186212,39.2978686649688,39.3655358516619),
 .UNSPECIFIED.);
#139=B_SPLINE_CURVE_WITH_KNOTS('',3,(#9772,#9773,#9774,#9775,#9776,#9777,
#9778,#9779,#9780,#9781,#9782,#9783,#9784,#9785,#9786,#9787,#9788,#9789,
#9790,#9791,#9792,#9793,#9794,#9795,#9796,#9797,#9798,#9799,#9800,#9801,
#9802,#9803,#9804,#9805,#9806,#9807,#9808,#9809,#9810,#9811,#9812,#9813,
#9814,#9815,#9816,#9817,#9818,#9819,#9820,#9821,#9822,#9823,#9824,#9825,
#9826,#9827,#9828,#9829,#9830,#9831,#9832,#9833,#9834,#9835,#9836,#9837,
#9838,#9839,#9840,#9841,#9842,#9843,#9844,#9845,#9846,#9847,#9848,#9849,
#9850,#9851,#9852,#9853,#9854,#9855,#9856,#9857,#9858,#9859,#9860,#9861),
 .UNSPECIFIED.,.F.,.F.,(4,2,2,2,2,2,2,2,2,2,2,2,2,2,2,2,2,2,2,2,2,2,2,2,
2,2,2,2,2,2,2,2,2,2,2,2,2,2,2,2,2,2,2,2,4),(0.000167115010632562,0.089463628004945,
0.250033227595873,0.40679334364094,0.599455029928833,0.709557528655732,
0.847466881949497,1.01852676597952,1.11408252919257,1.29448763332879,1.45527420990791,
1.64770353594286,1.76183295060474,1.89896780692874,2.06626165489344,2.16295304662853,
2.27218807214103,2.41408405866917,2.61102554534045,2.69650541653858,2.80439100592715,
2.94371708965856,3.12363136335108,3.21585090273878,3.39199485037615,3.55371328896186,
3.74598316810651,3.85235900021351,3.9922991398571,4.18810604298212,4.27229888220503,
4.37502957916033,4.51573723764941,4.71173916253334,4.79659919197649,4.90832981096552,
5.04628129377324,5.21729951277161,5.31294329014396,5.49270605398742,5.65389454952269,
5.84654957518262,5.95881353677797,6.09659716585997,6.23337760445098),
 .UNSPECIFIED.);
#140=B_SPLINE_CURVE_WITH_KNOTS('',3,(#9862,#9863,#9864,#9865,#9866,#9867,
#9868,#9869,#9870,#9871,#9872,#9873,#9874,#9875,#9876,#9877,#9878,#9879,
#9880,#9881,#9882,#9883,#9884,#9885,#9886,#9887,#9888,#9889,#9890,#9891,
#9892,#9893,#9894,#9895,#9896,#9897,#9898,#9899,#9900,#9901,#9902,#9903,
#9904,#9905,#9906,#9907,#9908,#9909,#9910,#9911,#9912,#9913,#9914,#9915,
#9916,#9917,#9918,#9919,#9920,#9921,#9922,#9923,#9924,#9925,#9926,#9927,
#9928,#9929,#9930,#9931,#9932,#9933,#9934,#9935,#9936,#9937,#9938,#9939,
#9940,#9941,#9942,#9943,#9944,#9945,#9946,#9947,#9948,#9949,#9950,#9951,
#9952,#9953,#9954,#9955,#9956,#9957,#9958,#9959,#9960,#9961,#9962,#9963),
 .UNSPECIFIED.,.F.,.F.,(4,2,2,2,2,2,2,2,2,2,2,2,2,2,2,2,2,2,2,2,2,2,2,2,
2,2,2,2,2,2,2,2,2,2,2,2,2,2,2,2,2,2,2,2,2,2,2,2,2,2,4),(30.8837752445267,
30.8985513929829,31.0027440740847,31.0885107450702,31.286137105715,31.4287223138741,
31.5367910962938,31.6340692241231,31.8008456401066,31.9381844314296,32.0520287869352,
32.2444973830893,32.4053508658922,32.5859358628873,32.6815315693023,32.8527112874765,
32.9907030816835,33.102527544385,33.1874107771474,33.3834603362991,33.5242072801014,
33.6283862497612,33.7141403102153,33.9117376999498,34.0543021429303,34.1623538351394,
34.2596179149756,34.4263689485974,34.5636873656241,34.6775144495382,34.7621518063255,
34.9580361662437,35.0984506837668,35.2110292174805,35.3062933455278,35.4782022778076,
35.6162659000383,35.7278089514407,35.8127161027665,36.0087700324591,36.1495508876168,
36.2522288887509,36.3364601035755,36.5322938606012,36.6722842831347,36.7786588078875,
36.9711336332874,37.1330696108447,37.3087527931773,37.4007818445533,37.4953062588109),
 .UNSPECIFIED.);
#141=B_SPLINE_CURVE_WITH_KNOTS('',3,(#9966,#9967,#9968,#9969,#9970,#9971,
#9972,#9973,#9974,#9975,#9976,#9977,#9978,#9979,#9980,#9981,#9982,#9983,
#9984,#9985,#9986,#9987,#9988,#9989,#9990,#9991,#9992,#9993,#9994,#9995,
#9996,#9997,#9998,#9999,#10000,#10001,#10002,#10003,#10004,#10005,#10006,
#10007,#10008,#10009,#10010,#10011,#10012,#10013,#10014,#10015,#10016,#10017,
#10018,#10019,#10020,#10021,#10022,#10023,#10024,#10025,#10026,#10027,#10028,
#10029,#10030,#10031,#10032,#10033,#10034,#10035,#10036,#10037,#10038,#10039,
#10040,#10041,#10042,#10043,#10044,#10045,#10046,#10047,#10048,#10049,#10050,
#10051,#10052,#10053,#10054,#10055,#10056,#10057,#10058,#10059,#10060,#10061),
 .UNSPECIFIED.,.F.,.F.,(4,2,2,2,2,2,2,2,2,2,2,2,2,2,2,2,2,2,2,2,2,2,2,2,
2,2,2,2,2,2,2,2,2,2,2,2,2,2,2,2,2,2,2,2,2,2,2,4),(37.4953062588109,37.580624778732,
37.7197557646577,37.8282792076654,37.9136581049212,38.1103703089893,38.2520187572005,
38.3618986649034,38.4583721738345,38.6259798462175,38.7631013939321,38.877424770735,
39.0700022564623,39.230922664749,39.4111958169609,39.506781849307,39.6778619379215,
39.8158050480093,39.9275760812986,40.0124351730281,40.2084252844014,40.3491389033369,
40.4518678475122,40.5360457888487,40.7318229906229,40.8717348049317,40.9781885420517,
41.1704701195794,41.332243773217,41.5082714258425,41.6004220997857,41.7802696498608,
41.9194967324815,42.0276105701555,42.220272096058,42.3820437005206,42.5580485181999,
42.6503136546282,42.8302519341941,42.9696994200002,43.0771426351419,43.2692475698609,
43.4296997938774,43.6106309098647,43.7071358476977,43.7706118235221,43.9091487174759,
44.0778884690173),.UNSPECIFIED.);
#142=B_SPLINE_CURVE_WITH_KNOTS('',3,(#10064,#10065,#10066,#10067,#10068,
#10069,#10070,#10071,#10072,#10073,#10074,#10075,#10076,#10077,#10078,#10079,
#10080,#10081,#10082,#10083,#10084,#10085,#10086,#10087,#10088,#10089,#10090,
#10091,#10092,#10093,#10094,#10095,#10096,#10097,#10098,#10099,#10100,#10101,
#10102,#10103,#10104,#10105,#10106,#10107,#10108,#10109,#10110,#10111,#10112,
#10113,#10114,#10115,#10116,#10117,#10118,#10119,#10120,#10121,#10122,#10123,
#10124,#10125,#10126,#10127,#10128,#10129,#10130,#10131,#10132,#10133,#10134,
#10135,#10136,#10137,#10138,#10139,#10140,#10141,#10142,#10143,#10144,#10145,
#10146,#10147,#10148,#10149,#10150,#10151,#10152,#10153,#10154,#10155,#10156,
#10157,#10158,#10159,#10160,#10161,#10162,#10163,#10164,#10165,#10166,#10167,
#10168,#10169,#10170,#10171,#10172,#10173,#10174,#10175,#10176,#10177,#10178,
#10179,#10180,#10181,#10182,#10183,#10184,#10185,#10186,#10187,#10188,#10189,
#10190,#10191,#10192,#10193,#10194,#10195,#10196,#10197,#10198,#10199,#10200,
#10201,#10202,#10203,#10204,#10205,#10206,#10207,#10208,#10209,#10210,#10211,
#10212,#10213,#10214,#10215,#10216,#10217,#10218,#10219,#10220,#10221,#10222,
#10223,#10224,#10225,#10226,#10227,#10228,#10229,#10230,#10231,#10232,#10233,
#10234,#10235,#10236,#10237,#10238,#10239,#10240,#10241,#10242,#10243,#10244,
#10245,#10246,#10247,#10248,#10249,#10250,#10251,#10252,#10253,#10254,#10255,
#10256),.UNSPECIFIED.,.F.,.F.,(4,3,3,3,3,3,3,3,3,3,3,3,3,3,3,3,3,3,3,3,
3,3,3,3,3,3,3,3,3,3,3,3,3,3,3,3,3,3,3,3,3,3,3,3,3,3,3,3,3,3,3,3,3,3,3,3,
3,3,3,3,3,3,3,3,4),(39.3655358516619,39.4205489266629,39.4932256719064,
39.5658896866156,39.6385455807481,39.7112072104722,39.7838675238176,39.856544881781,
39.9195432168738,39.9922242628658,40.0648925892348,40.1375527937686,40.2102187009694,
40.2828832672999,40.3555648079552,40.4185375070847,40.4912126225807,40.5638750101892,
40.6365292843827,40.7091893168006,40.7818480476756,40.8545238586228,40.9175317972957,
40.9902104856699,41.062876431308,41.1355342389029,41.2081977415302,41.2808599026547,
41.353539054321,41.4165260875066,41.4892161017965,41.561893459126,41.6345627313084,
41.7072376971512,41.7799113036542,41.8526017895959,41.9155203777175,41.988155950647,
42.0607786263891,42.1333931314236,42.2060135911872,42.2786329155975,42.3512698720499,
42.4145146679284,42.48729869792,42.5600703328061,42.632833872698,42.7056024032701,
42.7783690429378,42.8511510266575,42.9135089581394,42.9859787125309,43.0584354826672,
43.1308844455598,43.2033410888313,43.275797773863,43.3482751674385,43.4125032483503,
43.4856192267066,43.5587218933442,43.6318145250677,43.7049066040599,43.7779931512484,
43.8510867420094,43.9114975385612),.UNSPECIFIED.);
#143=B_SPLINE_CURVE_WITH_KNOTS('',3,(#10259,#10260,#10261,#10262,#10263,
#10264,#10265,#10266,#10267,#10268,#10269,#10270,#10271,#10272,#10273,#10274,
#10275,#10276,#10277,#10278,#10279,#10280,#10281,#10282,#10283,#10284,#10285,
#10286,#10287,#10288,#10289,#10290,#10291,#10292,#10293,#10294,#10295,#10296,
#10297,#10298,#10299,#10300,#10301,#10302,#10303,#10304,#10305,#10306,#10307,
#10308,#10309,#10310,#10311,#10312,#10313,#10314,#10315,#10316,#10317,#10318,
#10319,#10320,#10321,#10322,#10323,#10324,#10325,#10326,#10327,#10328,#10329,
#10330,#10331,#10332,#10333,#10334),.UNSPECIFIED.,.F.,.F.,(4,3,3,3,3,3,
3,3,3,3,3,3,3,3,3,3,3,3,3,3,3,3,3,3,3,4),(51.7052219494017,51.7752622461825,
51.8232741926851,51.8933148183004,51.9633435475172,52.0333645023577,52.1055904974923,
52.1756151937478,52.2489418383219,52.322268482896,52.3923090961645,52.4623378133711,
52.5323587565658,52.6045847607011,52.674609446344,52.7479361097254,52.8212627731069,
52.8913031445529,52.961331618526,53.0313523177225,53.1035785041213,53.1736029469128,
53.2469300051154,53.3202570633179,53.3951479415614,53.4070751110265),
 .UNSPECIFIED.);
#144=B_SPLINE_CURVE_WITH_KNOTS('',3,(#10336,#10337,#10338,#10339,#10340,
#10341,#10342,#10343,#10344),.UNSPECIFIED.,.F.,.F.,(4,1,1,1,1,1,4),(53.4070751344278,
53.8192513535288,54.3182456437397,54.8172399339506,55.3162342241615,55.8152285143725,
56.2866044747298),.UNSPECIFIED.);
#145=B_SPLINE_CURVE_WITH_KNOTS('',3,(#10348,#10349,#10350,#10351,#10352,
#10353,#10354,#10355),.UNSPECIFIED.,.F.,.F.,(4,1,1,1,1,4),(53.4070751110265,
53.7675563424624,54.2665506326734,54.7655449228843,55.2645392130952,55.7635335033061),
 .UNSPECIFIED.);
#146=B_SPLINE_CURVE_WITH_KNOTS('',3,(#10356,#10357,#10358,#10359,#10360,
#10361,#10362,#10363,#10364,#10365,#10366,#10367,#10368,#10369,#10370,#10371,
#10372,#10373,#10374,#10375,#10376,#10377,#10378,#10379,#10380,#10381,#10382,
#10383,#10384,#10385,#10386,#10387,#10388,#10389,#10390,#10391,#10392,#10393,
#10394,#10395,#10396,#10397,#10398,#10399,#10400,#10401,#10402,#10403,#10404,
#10405,#10406,#10407,#10408,#10409,#10410,#10411,#10412,#10413,#10414,#10415,
#10416,#10417,#10418,#10419,#10420,#10421,#10422,#10423,#10424,#10425,#10426,
#10427,#10428),.UNSPECIFIED.,.F.,.F.,(4,3,3,3,3,3,3,3,3,3,3,3,3,3,3,3,3,
3,3,3,3,3,3,3,4),(51.705223688797,51.7715791816187,51.8416224003585,51.9116537285312,
51.9816772813509,52.0539013289706,52.1239285887193,52.1972510302745,52.2705734718297,
52.3406109642765,52.4106365581925,52.4806543837547,52.5528827283262,52.6229043486391,
52.6962360553399,52.7695677620406,52.8396086885631,52.9096377028379,52.9796589263131,
53.0518847077977,53.1219096292928,53.1952358407721,53.2685620522515,53.3417764954199,
53.4070751084796),.UNSPECIFIED.);
#147=B_SPLINE_CURVE_WITH_KNOTS('',3,(#10794,#10795,#10796,#10797,#10798,
#10799,#10800,#10801,#10802,#10803,#10804,#10805,#10806,#10807,#10808,#10809,
#10810,#10811,#10812,#10813,#10814,#10815,#10816,#10817,#10818,#10819,#10820,
#10821,#10822,#10823,#10824,#10825,#10826,#10827,#10828,#10829,#10830,#10831,
#10832,#10833,#10834,#10835,#10836,#10837,#10838,#10839,#10840,#10841,#10842,
#10843,#10844,#10845,#10846,#10847,#10848,#10849,#10850,#10851,#10852,#10853,
#10854,#10855,#10856,#10857,#10858,#10859,#10860,#10861,#10862,#10863,#10864,
#10865,#10866,#10867,#10868,#10869,#10870,#10871,#10872,#10873,#10874,#10875,
#10876,#10877,#10878,#10879,#10880,#10881,#10882,#10883,#10884,#10885,#10886,
#10887,#10888,#10889,#10890,#10891,#10892,#10893,#10894,#10895,#10896,#10897,
#10898,#10899,#10900,#10901,#10902,#10903,#10904,#10905,#10906,#10907,#10908,
#10909,#10910,#10911,#10912,#10913,#10914),.UNSPECIFIED.,.F.,.F.,(4,3,3,
3,3,3,3,3,3,3,3,3,3,3,3,3,3,3,3,3,3,3,3,3,3,3,3,3,3,3,3,3,3,3,3,3,3,3,3,
3,4),(0.,0.0847077516937711,0.170225033889545,0.255907500532044,0.341119279232027,
0.425059357774081,0.455383656591401,0.465770691009882,0.474513364932373,
0.558298342951859,0.600642802906426,0.684662560232661,0.768686524706548,
0.851862297329437,0.912900878915177,0.924214418880625,0.933065505594978,
1.0153136859126,1.09836343076414,1.18141317561567,1.26373325194697,1.34541324334634,
1.36175593088453,1.37449997082537,1.4548533829364,1.53535345080198,1.61538859658373,
1.69412331509383,1.74187144182578,1.78111905912933,1.79651186345433,1.80847555043388,
1.88768501687034,1.96689410707861,2.04543359504746,2.05585238025418,2.07005430121714,
2.14795915943215,2.2248426348574,2.28089532743822,2.31010750305873),
 .UNSPECIFIED.);
#148=B_SPLINE_CURVE_WITH_KNOTS('',3,(#10915,#10916,#10917,#10918),
 .UNSPECIFIED.,.F.,.F.,(4,4),(-0.00101472999876572,0.),.UNSPECIFIED.);
#149=B_SPLINE_CURVE_WITH_KNOTS('',3,(#10919,#10920,#10921,#10922,#10923,
#10924,#10925,#10926,#10927,#10928,#10929,#10930,#10931,#10932,#10933,#10934,
#10935,#10936,#10937,#10938,#10939,#10940,#10941,#10942,#10943,#10944,#10945,
#10946,#10947,#10948,#10949,#10950,#10951,#10952,#10953,#10954,#10955,#10956,
#10957,#10958,#10959,#10960,#10961,#10962,#10963,#10964,#10965,#10966,#10967,
#10968,#10969,#10970,#10971,#10972,#10973,#10974,#10975,#10976,#10977,#10978,
#10979,#10980,#10981,#10982,#10983,#10984,#10985,#10986,#10987,#10988,#10989,
#10990,#10991,#10992,#10993,#10994,#10995,#10996,#10997,#10998,#10999,#11000,
#11001,#11002,#11003,#11004,#11005,#11006,#11007,#11008,#11009,#11010,#11011,
#11012,#11013,#11014,#11015,#11016,#11017,#11018,#11019,#11020,#11021,#11022,
#11023,#11024,#11025,#11026,#11027,#11028,#11029,#11030,#11031,#11032,#11033),
 .UNSPECIFIED.,.F.,.F.,(4,3,3,3,3,3,3,3,3,3,3,3,3,3,3,3,3,3,3,3,3,3,3,3,
3,3,3,3,3,3,3,3,3,3,3,3,3,3,4),(0.,0.0756021000860911,0.152393199558973,
0.230392842176159,0.308644925471132,0.386546669685798,0.408880923643587,
0.422045036140801,0.501691131550158,0.537249170842264,0.616137946028816,
0.695699298379207,0.775607582769941,0.834608203354004,0.843321085046558,
0.924172696188028,1.0095507158666,1.09492873554517,1.18019567138666,1.26546260722815,
1.27900992162839,1.28771744272705,1.36946368552726,1.45259721935328,1.53602421303373,
1.61905253984022,1.6726411664557,1.7128618032572,1.72976589348117,1.74248623587577,
1.82597852344175,1.91057121436523,1.99440626086767,2.0125183165509,2.02643670802463,
2.1120758801977,2.19783429697825,2.26933164573093,2.30291422475425),
 .UNSPECIFIED.);
#150=B_SPLINE_CURVE_WITH_KNOTS('',3,(#11398,#11399,#11400,#11401,#11402,
#11403,#11404,#11405,#11406,#11407,#11408,#11409,#11410,#11411,#11412,#11413,
#11414,#11415,#11416,#11417,#11418,#11419,#11420,#11421,#11422,#11423,#11424,
#11425,#11426,#11427,#11428,#11429,#11430,#11431,#11432,#11433,#11434,#11435,
#11436,#11437,#11438,#11439,#11440,#11441,#11442,#11443,#11444,#11445,#11446,
#11447,#11448,#11449,#11450,#11451,#11452,#11453,#11454,#11455,#11456,#11457,
#11458,#11459,#11460,#11461,#11462,#11463,#11464,#11465,#11466,#11467,#11468,
#11469,#11470,#11471,#11472,#11473,#11474,#11475,#11476,#11477,#11478,#11479,
#11480,#11481,#11482,#11483,#11484,#11485,#11486,#11487,#11488,#11489,#11490,
#11491,#11492,#11493,#11494,#11495,#11496,#11497,#11498,#11499,#11500,#11501,
#11502,#11503,#11504,#11505,#11506,#11507,#11508,#11509,#11510,#11511,#11512),
 .UNSPECIFIED.,.F.,.F.,(4,3,3,3,3,3,3,3,3,3,3,3,3,3,3,3,3,3,3,3,3,3,3,3,
3,3,3,3,3,3,3,3,3,3,3,3,3,3,4),(0.,0.0756020442574116,0.152393096832318,
0.230392716296112,0.308644793984952,0.386546557639097,0.408880856230141,
0.420928744427606,0.500569899331183,0.537249170842273,0.616073663427341,
0.695678467211851,0.775598186338839,0.815514504989629,0.834608290416057,
0.84847123329491,0.929373466901696,1.01215110122343,1.09492873554516,1.17606648597094,
1.25762667195969,1.27900990554167,1.28771743639829,1.3694636568822,1.45259718089028,
1.53602417080081,1.61905249837216,1.6726411664557,1.73231431654345,1.74174492869213,
1.82529436366379,1.90959642814042,1.99435898918172,2.01251832412271,2.02375496071478,
2.10938057767906,2.19514471614932,2.26933164573094,2.30291844692703),
 .UNSPECIFIED.);
#151=B_SPLINE_CURVE_WITH_KNOTS('',3,(#11513,#11514,#11515,#11516,#11517,
#11518,#11519,#11520,#11521,#11522,#11523,#11524,#11525,#11526,#11527,#11528,
#11529,#11530,#11531,#11532,#11533,#11534,#11535,#11536,#11537,#11538,#11539,
#11540,#11541,#11542,#11543,#11544,#11545,#11546,#11547,#11548,#11549,#11550,
#11551,#11552,#11553,#11554,#11555,#11556,#11557,#11558,#11559,#11560,#11561,
#11562,#11563,#11564,#11565,#11566,#11567,#11568,#11569,#11570,#11571,#11572,
#11573,#11574,#11575,#11576,#11577,#11578,#11579,#11580,#11581,#11582,#11583,
#11584,#11585,#11586,#11587,#11588,#11589,#11590,#11591,#11592,#11593,#11594,
#11595,#11596,#11597,#11598,#11599,#11600,#11601,#11602,#11603,#11604,#11605,
#11606,#11607,#11608,#11609,#11610,#11611,#11612,#11613,#11614,#11615,#11616,
#11617,#11618,#11619,#11620,#11621,#11622,#11623,#11624,#11625,#11626,#11627,
#11628,#11629,#11630,#11631,#11632,#11633,#11634,#11635,#11636),
 .UNSPECIFIED.,.F.,.F.,(4,3,3,3,3,3,3,3,3,3,3,3,3,3,3,3,3,3,3,3,3,3,3,3,
3,3,3,3,3,3,3,3,3,3,3,3,3,3,3,3,3,4),(6.61845341725208E-15,0.0849506171234816,
0.170583039076072,0.256324783691451,0.342404288495193,0.406963917098,0.455383638550105,
0.468536166046617,0.479421865514442,0.56319740127756,0.600642802906421,
0.684641773439832,0.768646494244517,0.852075754152883,0.893242931835729,
0.912628999565668,0.923529204327917,0.932945920282414,0.963808297499684,
1.04604185844047,1.12763182145717,1.18141317561565,1.26548811560765,1.34956305559966,
1.36175593015859,1.37449997074551,1.45485337915238,1.53535344652152,1.61538859015649,
1.6941233006684,1.74187144182573,1.79625541798791,1.80632110746682,1.88551239813008,
1.96470047939158,2.04374919140323,2.05752087865608,2.0731251477082,2.15101429053224,
2.22787487765179,2.28089532743819,2.31010750305869),.UNSPECIFIED.);
#388=FACE_BOUND('',#912,.T.);
#389=FACE_BOUND('',#920,.T.);
#410=CYLINDRICAL_SURFACE('',#4236,12.1745);
#411=CYLINDRICAL_SURFACE('',#4238,12.1745);
#412=CYLINDRICAL_SURFACE('',#4240,12.1745);
#413=CYLINDRICAL_SURFACE('',#4241,12.1745);
#414=CYLINDRICAL_SURFACE('',#4242,12.1745);
#415=CYLINDRICAL_SURFACE('',#4243,12.1745);
#416=CYLINDRICAL_SURFACE('',#4244,12.1745);
#417=CYLINDRICAL_SURFACE('',#4245,10.501);
#418=CYLINDRICAL_SURFACE('',#4247,10.501);
#419=CYLINDRICAL_SURFACE('',#4248,10.501);
#420=CYLINDRICAL_SURFACE('',#4249,10.501);
#421=CYLINDRICAL_SURFACE('',#4250,10.501);
#422=CYLINDRICAL_SURFACE('',#4251,10.501);
#423=CYLINDRICAL_SURFACE('',#4252,10.501);
#424=CYLINDRICAL_SURFACE('',#4254,12.1745);
#561=CIRCLE('',#4237,12.1745);
#562=CIRCLE('',#4239,12.1745);
#563=CIRCLE('',#4246,10.501);
#564=CIRCLE('',#4253,10.501);
#565=CIRCLE('',#4255,12.1745);
#687=FACE_OUTER_BOUND('',#894,.T.);
#688=FACE_OUTER_BOUND('',#895,.T.);
#689=FACE_OUTER_BOUND('',#896,.T.);
#690=FACE_OUTER_BOUND('',#897,.T.);
#691=FACE_OUTER_BOUND('',#898,.T.);
#692=FACE_OUTER_BOUND('',#899,.T.);
#693=FACE_OUTER_BOUND('',#900,.T.);
#694=FACE_OUTER_BOUND('',#901,.T.);
#695=FACE_OUTER_BOUND('',#902,.T.);
#696=FACE_OUTER_BOUND('',#903,.T.);
#697=FACE_OUTER_BOUND('',#904,.T.);
#698=FACE_OUTER_BOUND('',#905,.T.);
#699=FACE_OUTER_BOUND('',#906,.T.);
#700=FACE_OUTER_BOUND('',#907,.T.);
#701=FACE_OUTER_BOUND('',#908,.T.);
#702=FACE_OUTER_BOUND('',#909,.T.);
#703=FACE_OUTER_BOUND('',#910,.T.);
#704=FACE_OUTER_BOUND('',#911,.T.);
#705=FACE_OUTER_BOUND('',#913,.T.);
#706=FACE_OUTER_BOUND('',#914,.T.);
#707=FACE_OUTER_BOUND('',#915,.T.);
#708=FACE_OUTER_BOUND('',#916,.T.);
#709=FACE_OUTER_BOUND('',#917,.T.);
#710=FACE_OUTER_BOUND('',#918,.T.);
#711=FACE_OUTER_BOUND('',#919,.T.);
#894=EDGE_LOOP('',(#2744,#2745,#2746));
#895=EDGE_LOOP('',(#2747,#2748,#2749,#2750,#2751,#2752,#2753));
#896=EDGE_LOOP('',(#2754,#2755,#2756,#2757,#2758,#2759));
#897=EDGE_LOOP('',(#2760,#2761,#2762,#2763,#2764,#2765));
#898=EDGE_LOOP('',(#2766,#2767,#2768,#2769,#2770,#2771));
#899=EDGE_LOOP('',(#2772,#2773,#2774,#2775,#2776,#2777));
#900=EDGE_LOOP('',(#2778,#2779,#2780,#2781,#2782,#2783));
#901=EDGE_LOOP('',(#2784,#2785,#2786,#2787,#2788));
#902=EDGE_LOOP('',(#2789,#2790,#2791,#2792,#2793));
#903=EDGE_LOOP('',(#2794,#2795,#2796,#2797));
#904=EDGE_LOOP('',(#2798,#2799,#2800,#2801,#2802));
#905=EDGE_LOOP('',(#2803,#2804,#2805,#2806));
#906=EDGE_LOOP('',(#2807,#2808,#2809,#2810,#2811));
#907=EDGE_LOOP('',(#2812,#2813,#2814,#2815));
#908=EDGE_LOOP('',(#2816,#2817,#2818,#2819,#2820,#2821));
#909=EDGE_LOOP('',(#2822,#2823,#2824,#2825,#2826,#2827,#2828,#2829,#2830,
#2831,#2832,#2833,#2834,#2835,#2836,#2837,#2838,#2839,#2840,#2841,#2842,
#2843,#2844,#2845,#2846));
#910=EDGE_LOOP('',(#2847,#2848,#2849,#2850,#2851,#2852,#2853,#2854,#2855,
#2856,#2857,#2858,#2859,#2860,#2861,#2862,#2863,#2864,#2865,#2866,#2867,
#2868,#2869,#2870,#2871,#2872,#2873));
#911=EDGE_LOOP('',(#2874,#2875,#2876,#2877,#2878,#2879));
#912=EDGE_LOOP('',(#2880,#2881,#2882,#2883,#2884));
#913=EDGE_LOOP('',(#2885,#2886,#2887,#2888));
#914=EDGE_LOOP('',(#2889,#2890,#2891,#2892));
#915=EDGE_LOOP('',(#2893,#2894,#2895,#2896));
#916=EDGE_LOOP('',(#2897,#2898,#2899,#2900));
#917=EDGE_LOOP('',(#2901,#2902,#2903,#2904));
#918=EDGE_LOOP('',(#2905,#2906,#2907,#2908));
#919=EDGE_LOOP('',(#2909,#2910,#2911,#2912,#2913,#2914));
#920=EDGE_LOOP('',(#2915,#2916,#2917,#2918,#2919));
#1107=LINE('',#5955,#1320);
#1108=LINE('',#5968,#1321);
#1109=LINE('',#6267,#1322);
#1110=LINE('',#6749,#1323);
#1111=LINE('',#7299,#1324);
#1112=LINE('',#7666,#1325);
#1113=LINE('',#8148,#1326);
#1114=LINE('',#8698,#1327);
#1115=LINE('',#9018,#1328);
#1116=LINE('',#9149,#1329);
#1117=LINE('',#9351,#1330);
#1118=LINE('',#9548,#1331);
#1119=LINE('',#9754,#1332);
#1120=LINE('',#11640,#1333);
#1121=LINE('',#11642,#1334);
#1122=LINE('',#11644,#1335);
#1123=LINE('',#11646,#1336);
#1124=LINE('',#11648,#1337);
#1125=LINE('',#11649,#1338);
#1126=LINE('',#11653,#1339);
#1127=LINE('',#11654,#1340);
#1128=LINE('',#11655,#1341);
#1129=LINE('',#11658,#1342);
#1130=LINE('',#11659,#1343);
#1131=LINE('',#11662,#1344);
#1132=LINE('',#11663,#1345);
#1133=LINE('',#11666,#1346);
#1134=LINE('',#11667,#1347);
#1135=LINE('',#11670,#1348);
#1136=LINE('',#11671,#1349);
#1137=LINE('',#11673,#1350);
#1320=VECTOR('',#4716,12.1745);
#1321=VECTOR('',#4721,12.1745);
#1322=VECTOR('',#4726,12.1745);
#1323=VECTOR('',#4729,12.1745);
#1324=VECTOR('',#4732,12.1745);
#1325=VECTOR('',#4735,12.1745);
#1326=VECTOR('',#4738,12.1745);
#1327=VECTOR('',#4741,10.501);
#1328=VECTOR('',#4746,10.501);
#1329=VECTOR('',#4749,10.501);
#1330=VECTOR('',#4752,10.501);
#1331=VECTOR('',#4755,10.501);
#1332=VECTOR('',#4758,10.501);
#1333=VECTOR('',#4769,10.);
#1334=VECTOR('',#4770,10.);
#1335=VECTOR('',#4771,10.);
#1336=VECTOR('',#4772,10.);
#1337=VECTOR('',#4773,10.);
#1338=VECTOR('',#4774,10.);
#1339=VECTOR('',#4777,10.);
#1340=VECTOR('',#4778,10.);
#1341=VECTOR('',#4779,10.);
#1342=VECTOR('',#4782,10.);
#1343=VECTOR('',#4783,10.);
#1344=VECTOR('',#4786,10.);
#1345=VECTOR('',#4787,10.);
#1346=VECTOR('',#4790,10.);
#1347=VECTOR('',#4791,10.);
#1348=VECTOR('',#4794,10.);
#1349=VECTOR('',#4795,10.);
#1350=VECTOR('',#4798,10.);
#1543=VERTEX_POINT('',#5953);
#1544=VERTEX_POINT('',#5954);
#1545=VERTEX_POINT('',#5956);
#1546=VERTEX_POINT('',#5966);
#1547=VERTEX_POINT('',#5967);
#1548=VERTEX_POINT('',#5969);
#1549=VERTEX_POINT('',#6242);
#1550=VERTEX_POINT('',#6244);
#1551=VERTEX_POINT('',#6265);
#1552=VERTEX_POINT('',#6266);
#1553=VERTEX_POINT('',#6268);
#1554=VERTEX_POINT('',#6541);
#1555=VERTEX_POINT('',#6747);
#1556=VERTEX_POINT('',#6748);
#1557=VERTEX_POINT('',#6750);
#1558=VERTEX_POINT('',#7023);
#1559=VERTEX_POINT('',#7297);
#1560=VERTEX_POINT('',#7298);
#1561=VERTEX_POINT('',#7300);
#1562=VERTEX_POINT('',#7390);
#1563=VERTEX_POINT('',#7664);
#1564=VERTEX_POINT('',#7665);
#1565=VERTEX_POINT('',#7667);
#1566=VERTEX_POINT('',#7872);
#1567=VERTEX_POINT('',#8146);
#1568=VERTEX_POINT('',#8147);
#1569=VERTEX_POINT('',#8149);
#1570=VERTEX_POINT('',#8425);
#1571=VERTEX_POINT('',#8696);
#1572=VERTEX_POINT('',#8697);
#1573=VERTEX_POINT('',#8699);
#1574=VERTEX_POINT('',#8704);
#1575=VERTEX_POINT('',#8943);
#1576=VERTEX_POINT('',#9016);
#1577=VERTEX_POINT('',#9017);
#1578=VERTEX_POINT('',#9019);
#1579=VERTEX_POINT('',#9147);
#1580=VERTEX_POINT('',#9148);
#1581=VERTEX_POINT('',#9349);
#1582=VERTEX_POINT('',#9350);
#1583=VERTEX_POINT('',#9352);
#1584=VERTEX_POINT('',#9546);
#1585=VERTEX_POINT('',#9547);
#1586=VERTEX_POINT('',#9752);
#1587=VERTEX_POINT('',#9753);
#1588=VERTEX_POINT('',#9755);
#1589=VERTEX_POINT('',#9965);
#1590=VERTEX_POINT('',#10062);
#1591=VERTEX_POINT('',#10258);
#1592=VERTEX_POINT('',#10335);
#1593=VERTEX_POINT('',#10345);
#1594=VERTEX_POINT('',#10347);
#1595=VERTEX_POINT('',#10793);
#1596=VERTEX_POINT('',#11638);
#1597=VERTEX_POINT('',#11639);
#1598=VERTEX_POINT('',#11641);
#1599=VERTEX_POINT('',#11643);
#1600=VERTEX_POINT('',#11645);
#1601=VERTEX_POINT('',#11647);
#1602=VERTEX_POINT('',#11651);
#1603=VERTEX_POINT('',#11652);
#1604=VERTEX_POINT('',#11657);
#1605=VERTEX_POINT('',#11661);
#1606=VERTEX_POINT('',#11665);
#1607=VERTEX_POINT('',#11669);
#2023=EDGE_CURVE('',#1543,#1544,#1107,.T.);
#2024=EDGE_CURVE('',#1545,#1543,#100,.T.);
#2025=EDGE_CURVE('',#1545,#1544,#561,.T.);
#2026=EDGE_CURVE('',#1546,#1547,#1108,.T.);
#2027=EDGE_CURVE('',#1548,#1546,#101,.T.);
#2028=EDGE_CURVE('',#1543,#1548,#102,.T.);
#2029=EDGE_CURVE('',#1544,#1549,#562,.T.);
#2030=EDGE_CURVE('',#1549,#1550,#103,.T.);
#2031=EDGE_CURVE('',#1550,#1547,#104,.T.);
#2032=EDGE_CURVE('',#1551,#1552,#1109,.T.);
#2033=EDGE_CURVE('',#1553,#1551,#105,.T.);
#2034=EDGE_CURVE('',#1546,#1553,#106,.T.);
#2035=EDGE_CURVE('',#1547,#1554,#107,.T.);
#2036=EDGE_CURVE('',#1554,#1552,#108,.T.);
#2037=EDGE_CURVE('',#1555,#1556,#1110,.T.);
#2038=EDGE_CURVE('',#1557,#1555,#109,.T.);
#2039=EDGE_CURVE('',#1551,#1557,#110,.T.);
#2040=EDGE_CURVE('',#1552,#1558,#111,.T.);
#2041=EDGE_CURVE('',#1558,#1556,#112,.T.);
#2042=EDGE_CURVE('',#1559,#1560,#1111,.T.);
#2043=EDGE_CURVE('',#1561,#1559,#113,.T.);
#2044=EDGE_CURVE('',#1555,#1561,#114,.T.);
#2045=EDGE_CURVE('',#1556,#1562,#115,.T.);
#2046=EDGE_CURVE('',#1562,#1560,#116,.T.);
#2047=EDGE_CURVE('',#1563,#1564,#1112,.T.);
#2048=EDGE_CURVE('',#1565,#1563,#117,.T.);
#2049=EDGE_CURVE('',#1559,#1565,#118,.T.);
#2050=EDGE_CURVE('',#1560,#1566,#119,.T.);
#2051=EDGE_CURVE('',#1566,#1564,#120,.T.);
#2052=EDGE_CURVE('',#1567,#1568,#1113,.T.);
#2053=EDGE_CURVE('',#1569,#1567,#121,.T.);
#2054=EDGE_CURVE('',#1563,#1569,#122,.T.);
#2055=EDGE_CURVE('',#1564,#1570,#123,.T.);
#2056=EDGE_CURVE('',#1570,#1568,#124,.T.);
#2057=EDGE_CURVE('',#1571,#1572,#1114,.T.);
#2058=EDGE_CURVE('',#1573,#1571,#125,.T.);
#2059=EDGE_CURVE('',#1574,#1573,#126,.T.);
#2060=EDGE_CURVE('',#1575,#1574,#563,.F.);
#2061=EDGE_CURVE('',#1572,#1575,#127,.F.);
#2062=EDGE_CURVE('',#1576,#1577,#1115,.T.);
#2063=EDGE_CURVE('',#1578,#1576,#128,.F.);
#2064=EDGE_CURVE('',#1571,#1578,#129,.T.);
#2065=EDGE_CURVE('',#1577,#1572,#130,.F.);
#2066=EDGE_CURVE('',#1579,#1580,#1116,.T.);
#2067=EDGE_CURVE('',#1576,#1579,#131,.F.);
#2068=EDGE_CURVE('',#1580,#1577,#132,.F.);
#2069=EDGE_CURVE('',#1581,#1582,#1117,.T.);
#2070=EDGE_CURVE('',#1583,#1581,#133,.F.);
#2071=EDGE_CURVE('',#1579,#1583,#134,.F.);
#2072=EDGE_CURVE('',#1582,#1580,#135,.F.);
#2073=EDGE_CURVE('',#1584,#1585,#1118,.T.);
#2074=EDGE_CURVE('',#1581,#1584,#136,.F.);
#2075=EDGE_CURVE('',#1585,#1582,#137,.F.);
#2076=EDGE_CURVE('',#1586,#1587,#1119,.T.);
#2077=EDGE_CURVE('',#1588,#1586,#138,.T.);
#2078=EDGE_CURVE('',#1584,#1588,#139,.F.);
#2079=EDGE_CURVE('',#1587,#1585,#140,.F.);
#2080=EDGE_CURVE('',#1589,#1587,#141,.F.);
#2081=EDGE_CURVE('',#1589,#1590,#564,.F.);
#2082=EDGE_CURVE('',#1586,#1590,#142,.T.);
#2083=EDGE_CURVE('',#1568,#1591,#143,.T.);
#2084=EDGE_CURVE('',#1591,#1592,#144,.T.);
#2085=EDGE_CURVE('',#1592,#1593,#565,.T.);
#2086=EDGE_CURVE('',#1594,#1593,#145,.T.);
#2087=EDGE_CURVE('',#1567,#1594,#146,.T.);
#2088=EDGE_CURVE('',#1593,#1595,#147,.T.);
#2089=EDGE_CURVE('',#1595,#1589,#148,.T.);
#2090=EDGE_CURVE('',#1575,#1545,#149,.T.);
#2091=EDGE_CURVE('',#1590,#1592,#150,.T.);
#2092=EDGE_CURVE('',#1549,#1574,#151,.T.);
#2093=EDGE_CURVE('',#1596,#1597,#1120,.T.);
#2094=EDGE_CURVE('',#1598,#1596,#1121,.T.);
#2095=EDGE_CURVE('',#1599,#1598,#1122,.T.);
#2096=EDGE_CURVE('',#1600,#1599,#1123,.T.);
#2097=EDGE_CURVE('',#1601,#1600,#1124,.T.);
#2098=EDGE_CURVE('',#1597,#1601,#1125,.T.);
#2099=EDGE_CURVE('',#1602,#1603,#1126,.T.);
#2100=EDGE_CURVE('',#1602,#1598,#1127,.T.);
#2101=EDGE_CURVE('',#1603,#1596,#1128,.T.);
#2102=EDGE_CURVE('',#1604,#1602,#1129,.T.);
#2103=EDGE_CURVE('',#1604,#1599,#1130,.T.);
#2104=EDGE_CURVE('',#1605,#1604,#1131,.T.);
#2105=EDGE_CURVE('',#1605,#1600,#1132,.T.);
#2106=EDGE_CURVE('',#1606,#1605,#1133,.T.);
#2107=EDGE_CURVE('',#1606,#1601,#1134,.T.);
#2108=EDGE_CURVE('',#1607,#1606,#1135,.T.);
#2109=EDGE_CURVE('',#1607,#1597,#1136,.T.);
#2110=EDGE_CURVE('',#1603,#1607,#1137,.T.);
#2744=ORIENTED_EDGE('',*,*,#2023,.F.);
#2745=ORIENTED_EDGE('',*,*,#2024,.F.);
#2746=ORIENTED_EDGE('',*,*,#2025,.T.);
#2747=ORIENTED_EDGE('',*,*,#2026,.F.);
#2748=ORIENTED_EDGE('',*,*,#2027,.F.);
#2749=ORIENTED_EDGE('',*,*,#2028,.F.);
#2750=ORIENTED_EDGE('',*,*,#2023,.T.);
#2751=ORIENTED_EDGE('',*,*,#2029,.T.);
#2752=ORIENTED_EDGE('',*,*,#2030,.T.);
#2753=ORIENTED_EDGE('',*,*,#2031,.T.);
#2754=ORIENTED_EDGE('',*,*,#2032,.F.);
#2755=ORIENTED_EDGE('',*,*,#2033,.F.);
#2756=ORIENTED_EDGE('',*,*,#2034,.F.);
#2757=ORIENTED_EDGE('',*,*,#2026,.T.);
#2758=ORIENTED_EDGE('',*,*,#2035,.T.);
#2759=ORIENTED_EDGE('',*,*,#2036,.T.);
#2760=ORIENTED_EDGE('',*,*,#2037,.F.);
#2761=ORIENTED_EDGE('',*,*,#2038,.F.);
#2762=ORIENTED_EDGE('',*,*,#2039,.F.);
#2763=ORIENTED_EDGE('',*,*,#2032,.T.);
#2764=ORIENTED_EDGE('',*,*,#2040,.T.);
#2765=ORIENTED_EDGE('',*,*,#2041,.T.);
#2766=ORIENTED_EDGE('',*,*,#2042,.F.);
#2767=ORIENTED_EDGE('',*,*,#2043,.F.);
#2768=ORIENTED_EDGE('',*,*,#2044,.F.);
#2769=ORIENTED_EDGE('',*,*,#2037,.T.);
#2770=ORIENTED_EDGE('',*,*,#2045,.T.);
#2771=ORIENTED_EDGE('',*,*,#2046,.T.);
#2772=ORIENTED_EDGE('',*,*,#2047,.F.);
#2773=ORIENTED_EDGE('',*,*,#2048,.F.);
#2774=ORIENTED_EDGE('',*,*,#2049,.F.);
#2775=ORIENTED_EDGE('',*,*,#2042,.T.);
#2776=ORIENTED_EDGE('',*,*,#2050,.T.);
#2777=ORIENTED_EDGE('',*,*,#2051,.T.);
#2778=ORIENTED_EDGE('',*,*,#2052,.F.);
#2779=ORIENTED_EDGE('',*,*,#2053,.F.);
#2780=ORIENTED_EDGE('',*,*,#2054,.F.);
#2781=ORIENTED_EDGE('',*,*,#2047,.T.);
#2782=ORIENTED_EDGE('',*,*,#2055,.T.);
#2783=ORIENTED_EDGE('',*,*,#2056,.T.);
#2784=ORIENTED_EDGE('',*,*,#2057,.F.);
#2785=ORIENTED_EDGE('',*,*,#2058,.F.);
#2786=ORIENTED_EDGE('',*,*,#2059,.F.);
#2787=ORIENTED_EDGE('',*,*,#2060,.F.);
#2788=ORIENTED_EDGE('',*,*,#2061,.F.);
#2789=ORIENTED_EDGE('',*,*,#2062,.F.);
#2790=ORIENTED_EDGE('',*,*,#2063,.F.);
#2791=ORIENTED_EDGE('',*,*,#2064,.F.);
#2792=ORIENTED_EDGE('',*,*,#2057,.T.);
#2793=ORIENTED_EDGE('',*,*,#2065,.F.);
#2794=ORIENTED_EDGE('',*,*,#2066,.F.);
#2795=ORIENTED_EDGE('',*,*,#2067,.F.);
#2796=ORIENTED_EDGE('',*,*,#2062,.T.);
#2797=ORIENTED_EDGE('',*,*,#2068,.F.);
#2798=ORIENTED_EDGE('',*,*,#2069,.F.);
#2799=ORIENTED_EDGE('',*,*,#2070,.F.);
#2800=ORIENTED_EDGE('',*,*,#2071,.F.);
#2801=ORIENTED_EDGE('',*,*,#2066,.T.);
#2802=ORIENTED_EDGE('',*,*,#2072,.F.);
#2803=ORIENTED_EDGE('',*,*,#2073,.F.);
#2804=ORIENTED_EDGE('',*,*,#2074,.F.);
#2805=ORIENTED_EDGE('',*,*,#2069,.T.);
#2806=ORIENTED_EDGE('',*,*,#2075,.F.);
#2807=ORIENTED_EDGE('',*,*,#2076,.F.);
#2808=ORIENTED_EDGE('',*,*,#2077,.F.);
#2809=ORIENTED_EDGE('',*,*,#2078,.F.);
#2810=ORIENTED_EDGE('',*,*,#2073,.T.);
#2811=ORIENTED_EDGE('',*,*,#2079,.F.);
#2812=ORIENTED_EDGE('',*,*,#2076,.T.);
#2813=ORIENTED_EDGE('',*,*,#2080,.F.);
#2814=ORIENTED_EDGE('',*,*,#2081,.T.);
#2815=ORIENTED_EDGE('',*,*,#2082,.F.);
#2816=ORIENTED_EDGE('',*,*,#2052,.T.);
#2817=ORIENTED_EDGE('',*,*,#2083,.T.);
#2818=ORIENTED_EDGE('',*,*,#2084,.T.);
#2819=ORIENTED_EDGE('',*,*,#2085,.T.);
#2820=ORIENTED_EDGE('',*,*,#2086,.F.);
#2821=ORIENTED_EDGE('',*,*,#2087,.F.);
#2822=ORIENTED_EDGE('',*,*,#2088,.T.);
#2823=ORIENTED_EDGE('',*,*,#2089,.T.);
#2824=ORIENTED_EDGE('',*,*,#2080,.T.);
#2825=ORIENTED_EDGE('',*,*,#2079,.T.);
#2826=ORIENTED_EDGE('',*,*,#2075,.T.);
#2827=ORIENTED_EDGE('',*,*,#2072,.T.);
#2828=ORIENTED_EDGE('',*,*,#2068,.T.);
#2829=ORIENTED_EDGE('',*,*,#2065,.T.);
#2830=ORIENTED_EDGE('',*,*,#2061,.T.);
#2831=ORIENTED_EDGE('',*,*,#2090,.T.);
#2832=ORIENTED_EDGE('',*,*,#2024,.T.);
#2833=ORIENTED_EDGE('',*,*,#2028,.T.);
#2834=ORIENTED_EDGE('',*,*,#2027,.T.);
#2835=ORIENTED_EDGE('',*,*,#2034,.T.);
#2836=ORIENTED_EDGE('',*,*,#2033,.T.);
#2837=ORIENTED_EDGE('',*,*,#2039,.T.);
#2838=ORIENTED_EDGE('',*,*,#2038,.T.);
#2839=ORIENTED_EDGE('',*,*,#2044,.T.);
#2840=ORIENTED_EDGE('',*,*,#2043,.T.);
#2841=ORIENTED_EDGE('',*,*,#2049,.T.);
#2842=ORIENTED_EDGE('',*,*,#2048,.T.);
#2843=ORIENTED_EDGE('',*,*,#2054,.T.);
#2844=ORIENTED_EDGE('',*,*,#2053,.T.);
#2845=ORIENTED_EDGE('',*,*,#2087,.T.);
#2846=ORIENTED_EDGE('',*,*,#2086,.T.);
#2847=ORIENTED_EDGE('',*,*,#2091,.T.);
#2848=ORIENTED_EDGE('',*,*,#2084,.F.);
#2849=ORIENTED_EDGE('',*,*,#2083,.F.);
#2850=ORIENTED_EDGE('',*,*,#2056,.F.);
#2851=ORIENTED_EDGE('',*,*,#2055,.F.);
#2852=ORIENTED_EDGE('',*,*,#2051,.F.);
#2853=ORIENTED_EDGE('',*,*,#2050,.F.);
#2854=ORIENTED_EDGE('',*,*,#2046,.F.);
#2855=ORIENTED_EDGE('',*,*,#2045,.F.);
#2856=ORIENTED_EDGE('',*,*,#2041,.F.);
#2857=ORIENTED_EDGE('',*,*,#2040,.F.);
#2858=ORIENTED_EDGE('',*,*,#2036,.F.);
#2859=ORIENTED_EDGE('',*,*,#2035,.F.);
#2860=ORIENTED_EDGE('',*,*,#2031,.F.);
#2861=ORIENTED_EDGE('',*,*,#2030,.F.);
#2862=ORIENTED_EDGE('',*,*,#2092,.T.);
#2863=ORIENTED_EDGE('',*,*,#2059,.T.);
#2864=ORIENTED_EDGE('',*,*,#2058,.T.);
#2865=ORIENTED_EDGE('',*,*,#2064,.T.);
#2866=ORIENTED_EDGE('',*,*,#2063,.T.);
#2867=ORIENTED_EDGE('',*,*,#2067,.T.);
#2868=ORIENTED_EDGE('',*,*,#2071,.T.);
#2869=ORIENTED_EDGE('',*,*,#2070,.T.);
#2870=ORIENTED_EDGE('',*,*,#2074,.T.);
#2871=ORIENTED_EDGE('',*,*,#2078,.T.);
#2872=ORIENTED_EDGE('',*,*,#2077,.T.);
#2873=ORIENTED_EDGE('',*,*,#2082,.T.);
#2874=ORIENTED_EDGE('',*,*,#2093,.F.);
#2875=ORIENTED_EDGE('',*,*,#2094,.F.);
#2876=ORIENTED_EDGE('',*,*,#2095,.F.);
#2877=ORIENTED_EDGE('',*,*,#2096,.F.);
#2878=ORIENTED_EDGE('',*,*,#2097,.F.);
#2879=ORIENTED_EDGE('',*,*,#2098,.F.);
#2880=ORIENTED_EDGE('',*,*,#2091,.F.);
#2881=ORIENTED_EDGE('',*,*,#2081,.F.);
#2882=ORIENTED_EDGE('',*,*,#2089,.F.);
#2883=ORIENTED_EDGE('',*,*,#2088,.F.);
#2884=ORIENTED_EDGE('',*,*,#2085,.F.);
#2885=ORIENTED_EDGE('',*,*,#2099,.F.);
#2886=ORIENTED_EDGE('',*,*,#2100,.T.);
#2887=ORIENTED_EDGE('',*,*,#2094,.T.);
#2888=ORIENTED_EDGE('',*,*,#2101,.F.);
#2889=ORIENTED_EDGE('',*,*,#2102,.F.);
#2890=ORIENTED_EDGE('',*,*,#2103,.T.);
#2891=ORIENTED_EDGE('',*,*,#2095,.T.);
#2892=ORIENTED_EDGE('',*,*,#2100,.F.);
#2893=ORIENTED_EDGE('',*,*,#2104,.F.);
#2894=ORIENTED_EDGE('',*,*,#2105,.T.);
#2895=ORIENTED_EDGE('',*,*,#2096,.T.);
#2896=ORIENTED_EDGE('',*,*,#2103,.F.);
#2897=ORIENTED_EDGE('',*,*,#2106,.F.);
#2898=ORIENTED_EDGE('',*,*,#2107,.T.);
#2899=ORIENTED_EDGE('',*,*,#2097,.T.);
#2900=ORIENTED_EDGE('',*,*,#2105,.F.);
#2901=ORIENTED_EDGE('',*,*,#2108,.F.);
#2902=ORIENTED_EDGE('',*,*,#2109,.T.);
#2903=ORIENTED_EDGE('',*,*,#2098,.T.);
#2904=ORIENTED_EDGE('',*,*,#2107,.F.);
#2905=ORIENTED_EDGE('',*,*,#2110,.F.);
#2906=ORIENTED_EDGE('',*,*,#2101,.T.);
#2907=ORIENTED_EDGE('',*,*,#2093,.T.);
#2908=ORIENTED_EDGE('',*,*,#2109,.F.);
#2909=ORIENTED_EDGE('',*,*,#2110,.T.);
#2910=ORIENTED_EDGE('',*,*,#2108,.T.);
#2911=ORIENTED_EDGE('',*,*,#2106,.T.);
#2912=ORIENTED_EDGE('',*,*,#2104,.T.);
#2913=ORIENTED_EDGE('',*,*,#2102,.T.);
#2914=ORIENTED_EDGE('',*,*,#2099,.T.);
#2915=ORIENTED_EDGE('',*,*,#2092,.F.);
#2916=ORIENTED_EDGE('',*,*,#2029,.F.);
#2917=ORIENTED_EDGE('',*,*,#2025,.F.);
#2918=ORIENTED_EDGE('',*,*,#2090,.F.);
#2919=ORIENTED_EDGE('',*,*,#2060,.T.);
#3798=PLANE('',#4256);
#3799=PLANE('',#4257);
#3800=PLANE('',#4258);
#3801=PLANE('',#4259);
#3802=PLANE('',#4260);
#3803=PLANE('',#4261);
#3804=PLANE('',#4262);
#3805=PLANE('',#4263);
#3883=ADVANCED_FACE('',(#687),#410,.F.);
#3884=ADVANCED_FACE('',(#688),#411,.F.);
#3885=ADVANCED_FACE('',(#689),#412,.F.);
#3886=ADVANCED_FACE('',(#690),#413,.F.);
#3887=ADVANCED_FACE('',(#691),#414,.F.);
#3888=ADVANCED_FACE('',(#692),#415,.F.);
#3889=ADVANCED_FACE('',(#693),#416,.F.);
#3890=ADVANCED_FACE('',(#694),#417,.F.);
#3891=ADVANCED_FACE('',(#695),#418,.F.);
#3892=ADVANCED_FACE('',(#696),#419,.F.);
#3893=ADVANCED_FACE('',(#697),#420,.F.);
#3894=ADVANCED_FACE('',(#698),#421,.F.);
#3895=ADVANCED_FACE('',(#699),#422,.F.);
#3896=ADVANCED_FACE('',(#700),#423,.F.);
#3897=ADVANCED_FACE('',(#701),#424,.F.);
#3898=ADVANCED_FACE('',(#702),#86,.T.);
#3899=ADVANCED_FACE('',(#703),#87,.T.);
#3900=ADVANCED_FACE('',(#704,#388),#3798,.F.);
#3901=ADVANCED_FACE('',(#705),#3799,.F.);
#3902=ADVANCED_FACE('',(#706),#3800,.F.);
#3903=ADVANCED_FACE('',(#707),#3801,.F.);
#3904=ADVANCED_FACE('',(#708),#3802,.F.);
#3905=ADVANCED_FACE('',(#709),#3803,.F.);
#3906=ADVANCED_FACE('',(#710),#3804,.F.);
#3907=ADVANCED_FACE('',(#711,#389),#3805,.T.);
#4035=CLOSED_SHELL('',(#3883,#3884,#3885,#3886,#3887,#3888,#3889,#3890,
#3891,#3892,#3893,#3894,#3895,#3896,#3897,#3898,#3899,#3900,#3901,#3902,
#3903,#3904,#3905,#3906,#3907));
#4235=AXIS2_PLACEMENT_3D('',#5951,#4712,#4713);
#4236=AXIS2_PLACEMENT_3D('',#5952,#4714,#4715);
#4237=AXIS2_PLACEMENT_3D('',#5964,#4717,#4718);
#4238=AXIS2_PLACEMENT_3D('',#5965,#4719,#4720);
#4239=AXIS2_PLACEMENT_3D('',#6243,#4722,#4723);
#4240=AXIS2_PLACEMENT_3D('',#6264,#4724,#4725);
#4241=AXIS2_PLACEMENT_3D('',#6746,#4727,#4728);
#4242=AXIS2_PLACEMENT_3D('',#7296,#4730,#4731);
#4243=AXIS2_PLACEMENT_3D('',#7663,#4733,#4734);
#4244=AXIS2_PLACEMENT_3D('',#8145,#4736,#4737);
#4245=AXIS2_PLACEMENT_3D('',#8695,#4739,#4740);
#4246=AXIS2_PLACEMENT_3D('',#8944,#4742,#4743);
#4247=AXIS2_PLACEMENT_3D('',#9015,#4744,#4745);
#4248=AXIS2_PLACEMENT_3D('',#9146,#4747,#4748);
#4249=AXIS2_PLACEMENT_3D('',#9348,#4750,#4751);
#4250=AXIS2_PLACEMENT_3D('',#9545,#4753,#4754);
#4251=AXIS2_PLACEMENT_3D('',#9751,#4756,#4757);
#4252=AXIS2_PLACEMENT_3D('',#9964,#4759,#4760);
#4253=AXIS2_PLACEMENT_3D('',#10063,#4761,#4762);
#4254=AXIS2_PLACEMENT_3D('',#10257,#4763,#4764);
#4255=AXIS2_PLACEMENT_3D('',#10346,#4765,#4766);
#4256=AXIS2_PLACEMENT_3D('',#11637,#4767,#4768);
#4257=AXIS2_PLACEMENT_3D('',#11650,#4775,#4776);
#4258=AXIS2_PLACEMENT_3D('',#11656,#4780,#4781);
#4259=AXIS2_PLACEMENT_3D('',#11660,#4784,#4785);
#4260=AXIS2_PLACEMENT_3D('',#11664,#4788,#4789);
#4261=AXIS2_PLACEMENT_3D('',#11668,#4792,#4793);
#4262=AXIS2_PLACEMENT_3D('',#11672,#4796,#4797);
#4263=AXIS2_PLACEMENT_3D('',#11674,#4799,#4800);
#4712=DIRECTION('axis',(0.,0.,1.));
#4713=DIRECTION('refdir',(1.,0.,0.));
#4714=DIRECTION('center_axis',(0.,-1.,0.));
#4715=DIRECTION('ref_axis',(-0.130665282675078,0.,-0.991426539842182));
#4716=DIRECTION('',(0.,-1.,0.));
#4717=DIRECTION('center_axis',(0.,-1.,0.));
#4718=DIRECTION('ref_axis',(1.,0.,1.81309624337467E-14));
#4719=DIRECTION('center_axis',(0.,-1.,0.));
#4720=DIRECTION('ref_axis',(-0.130665282675078,0.,-0.991426539842182));
#4721=DIRECTION('',(0.,-1.,0.));
#4722=DIRECTION('center_axis',(0.,-1.,0.));
#4723=DIRECTION('ref_axis',(1.,0.,1.81309624337467E-14));
#4724=DIRECTION('center_axis',(0.,-1.,0.));
#4725=DIRECTION('ref_axis',(-0.130665282675078,0.,-0.991426539842182));
#4726=DIRECTION('',(0.,-1.,0.));
#4727=DIRECTION('center_axis',(0.,-1.,0.));
#4728=DIRECTION('ref_axis',(-0.130665282675078,0.,-0.991426539842182));
#4729=DIRECTION('',(0.,-1.,0.));
#4730=DIRECTION('center_axis',(0.,-1.,0.));
#4731=DIRECTION('ref_axis',(-0.130665282675078,0.,-0.991426539842182));
#4732=DIRECTION('',(0.,-1.,0.));
#4733=DIRECTION('center_axis',(0.,-1.,0.));
#4734=DIRECTION('ref_axis',(-0.130665282675078,0.,-0.991426539842182));
#4735=DIRECTION('',(0.,-1.,0.));
#4736=DIRECTION('center_axis',(0.,-1.,0.));
#4737=DIRECTION('ref_axis',(-0.130665282675078,0.,-0.991426539842182));
#4738=DIRECTION('',(0.,-1.,0.));
#4739=DIRECTION('center_axis',(0.,-1.,0.));
#4740=DIRECTION('ref_axis',(0.936888000853192,0.,0.349629623826857));
#4741=DIRECTION('',(0.,-1.,0.));
#4742=DIRECTION('center_axis',(0.,-1.,0.));
#4743=DIRECTION('ref_axis',(1.,0.,0.));
#4744=DIRECTION('center_axis',(0.,-1.,0.));
#4745=DIRECTION('ref_axis',(0.936888000853192,0.,0.349629623826857));
#4746=DIRECTION('',(0.,-1.,0.));
#4747=DIRECTION('center_axis',(0.,-1.,0.));
#4748=DIRECTION('ref_axis',(0.936888000853192,0.,0.349629623826857));
#4749=DIRECTION('',(0.,-1.,0.));
#4750=DIRECTION('center_axis',(0.,-1.,0.));
#4751=DIRECTION('ref_axis',(0.936888000853192,0.,0.349629623826857));
#4752=DIRECTION('',(0.,-1.,0.));
#4753=DIRECTION('center_axis',(0.,-1.,0.));
#4754=DIRECTION('ref_axis',(0.936888000853192,0.,0.349629623826857));
#4755=DIRECTION('',(0.,-1.,0.));
#4756=DIRECTION('center_axis',(0.,-1.,0.));
#4757=DIRECTION('ref_axis',(0.936888000853192,0.,0.349629623826857));
#4758=DIRECTION('',(0.,-1.,0.));
#4759=DIRECTION('center_axis',(0.,-1.,0.));
#4760=DIRECTION('ref_axis',(0.936888000853192,0.,0.349629623826857));
#4761=DIRECTION('center_axis',(0.,-1.,0.));
#4762=DIRECTION('ref_axis',(1.,0.,0.));
#4763=DIRECTION('center_axis',(0.,-1.,0.));
#4764=DIRECTION('ref_axis',(-0.130665282675078,0.,-0.991426539842182));
#4765=DIRECTION('center_axis',(0.,1.,0.));
#4766=DIRECTION('ref_axis',(1.,0.,1.81309624337467E-14));
#4767=DIRECTION('center_axis',(0.,-1.,0.));
#4768=DIRECTION('ref_axis',(1.,0.,0.));
#4769=DIRECTION('',(-1.,0.,4.69353744302978E-16));
#4770=DIRECTION('',(-0.499999999999999,0.,0.866025403784439));
#4771=DIRECTION('',(0.500000000000001,0.,0.866025403784438));
#4772=DIRECTION('',(1.,0.,-4.69353744302978E-16));
#4773=DIRECTION('',(0.5,0.,-0.866025403784439));
#4774=DIRECTION('',(-0.5,0.,-0.866025403784439));
#4775=DIRECTION('center_axis',(-0.866025403784439,0.,-0.499999999999999));
#4776=DIRECTION('ref_axis',(-0.499999999999999,0.,0.866025403784439));
#4777=DIRECTION('',(-0.499999999999999,0.,0.866025403784439));
#4778=DIRECTION('',(0.,1.,0.));
#4779=DIRECTION('',(0.,1.,0.));
#4780=DIRECTION('center_axis',(-0.866025403784438,0.,0.500000000000001));
#4781=DIRECTION('ref_axis',(0.500000000000001,0.,0.866025403784438));
#4782=DIRECTION('',(0.500000000000001,0.,0.866025403784438));
#4783=DIRECTION('',(0.,1.,0.));
#4784=DIRECTION('center_axis',(4.69353744302978E-16,0.,1.));
#4785=DIRECTION('ref_axis',(1.,0.,-4.69353744302978E-16));
#4786=DIRECTION('',(1.,0.,-4.69353744302978E-16));
#4787=DIRECTION('',(0.,1.,0.));
#4788=DIRECTION('center_axis',(0.866025403784439,0.,0.5));
#4789=DIRECTION('ref_axis',(0.5,0.,-0.866025403784439));
#4790=DIRECTION('',(0.5,0.,-0.866025403784439));
#4791=DIRECTION('',(0.,1.,0.));
#4792=DIRECTION('center_axis',(0.866025403784439,0.,-0.5));
#4793=DIRECTION('ref_axis',(-0.5,0.,-0.866025403784439));
#4794=DIRECTION('',(-0.5,0.,-0.866025403784439));
#4795=DIRECTION('',(0.,1.,0.));
#4796=DIRECTION('center_axis',(-4.69353744302978E-16,0.,-1.));
#4797=DIRECTION('ref_axis',(-1.,0.,4.69353744302978E-16));
#4798=DIRECTION('',(-1.,0.,4.69353744302978E-16));
#4799=DIRECTION('center_axis',(0.,-1.,0.));
#4800=DIRECTION('ref_axis',(1.,0.,0.));
#5951=CARTESIAN_POINT('',(0.,0.,0.));
#5952=CARTESIAN_POINT('Origin',(0.,13.3748739960349,0.));
#5953=CARTESIAN_POINT('',(1.59078448392775,20.0623165459775,12.0701224093086));
#5954=CARTESIAN_POINT('',(1.59078448392774,20.,12.0701224093086));
#5955=CARTESIAN_POINT('',(1.59078448392774,13.3748739960349,12.0701224093086));
#5956=CARTESIAN_POINT('',(3.14799128255578,20.,11.7604677260283));
#5957=CARTESIAN_POINT('Ctrl Pts',(3.14799128255578,20.,11.7604677260283));
#5958=CARTESIAN_POINT('Ctrl Pts',(2.8740867128099,20.0111238992557,11.8337853200134));
#5959=CARTESIAN_POINT('Ctrl Pts',(2.59757666171726,20.0222477985115,11.8975412512316));
#5960=CARTESIAN_POINT('Ctrl Pts',(2.31914702161461,20.0333716977672,11.9515692418249));
#5961=CARTESIAN_POINT('Ctrl Pts',(2.07765185627277,20.043019980504,11.9984302675283));
#5962=CARTESIAN_POINT('Ctrl Pts',(1.83471293240725,20.0526682632408,12.0379738048562));
#5963=CARTESIAN_POINT('Ctrl Pts',(1.59078448392775,20.0623165459775,12.0701224093086));
#5964=CARTESIAN_POINT('Origin',(0.,20.,0.));
#5965=CARTESIAN_POINT('Origin',(0.,13.3748739960349,0.));
#5966=CARTESIAN_POINT('',(1.59078448392772,23.0623012722853,12.0701224093087));
#5967=CARTESIAN_POINT('',(1.5908148051505,22.812547089465,12.070351758578));
#5968=CARTESIAN_POINT('',(1.59078448392774,13.3748739960349,12.0701224093086));
#5969=CARTESIAN_POINT('',(-12.1744999960254,20.8748739960726,-0.000311090449405607));
#5970=CARTESIAN_POINT('Ctrl Pts',(-12.1744999960254,20.8748739960726,-0.000311090449404772));
#5971=CARTESIAN_POINT('Ctrl Pts',(-12.1744923950652,20.8865393020214,-0.297774062673808));
#5972=CARTESIAN_POINT('Ctrl Pts',(-12.1635784601364,20.8982046079702,-0.595182841827181));
#5973=CARTESIAN_POINT('Ctrl Pts',(-12.1417960711354,20.909869913919,-0.891761412577232));
#5974=CARTESIAN_POINT('Ctrl Pts',(-12.1231530265705,20.9198539803433,-1.14559617382575));
#5975=CARTESIAN_POINT('Ctrl Pts',(-12.0965494250141,20.9298380467676,-1.39882274221339));
#5976=CARTESIAN_POINT('Ctrl Pts',(-12.0620392196327,20.939822113192,-1.65095733259334));
#5977=CARTESIAN_POINT('Ctrl Pts',(-12.0235090635879,20.9509691820964,-1.9324620354562));
#5978=CARTESIAN_POINT('Ctrl Pts',(-11.9751141751885,20.9621162510008,-2.2126594358091));
#5979=CARTESIAN_POINT('Ctrl Pts',(-11.9169675814257,20.9732633199052,-2.49085003829017));
#5980=CARTESIAN_POINT('Ctrl Pts',(-11.8588308783237,20.9844084927074,-2.76899332090735));
#5981=CARTESIAN_POINT('Ctrl Pts',(-11.7909458361135,20.9955536655097,-3.04513022613635));
#5982=CARTESIAN_POINT('Ctrl Pts',(-11.7134766039781,21.006698838312,-3.31857139414821));
#5983=CARTESIAN_POINT('Ctrl Pts',(-11.6360159868468,21.0178427717099,-3.591982154));
#5984=CARTESIAN_POINT('Ctrl Pts',(-11.5489733807489,21.0289867051078,-3.86269751864585));
#5985=CARTESIAN_POINT('Ctrl Pts',(-11.4525631648402,21.0401306385056,-4.1300420343315));
#5986=CARTESIAN_POINT('Ctrl Pts',(-11.3531130779724,21.0516259466949,-4.40581608024554));
#5987=CARTESIAN_POINT('Ctrl Pts',(-11.2436951564039,21.0631212548842,-4.67800297633621));
#5988=CARTESIAN_POINT('Ctrl Pts',(-11.1245994311076,21.0746165630735,-4.94588088689978));
#5989=CARTESIAN_POINT('Ctrl Pts',(-11.0091379329855,21.0857610898951,-5.20558445552521));
#5990=CARTESIAN_POINT('Ctrl Pts',(-10.8845806273897,21.0969056167168,-5.46123786352323));
#5991=CARTESIAN_POINT('Ctrl Pts',(-10.7512401330826,21.1080501435385,-5.71220499026376));
#5992=CARTESIAN_POINT('Ctrl Pts',(-10.6116041681331,21.1197208424116,-5.97502115196405));
#5993=CARTESIAN_POINT('Ctrl Pts',(-10.4623358132792,21.1313915412847,-6.23269757967499));
#5994=CARTESIAN_POINT('Ctrl Pts',(-10.3038478790065,21.1430622401578,-6.48453307002857));
#5995=CARTESIAN_POINT('Ctrl Pts',(-10.1453599447337,21.1547329390309,-6.73636856038215));
#5996=CARTESIAN_POINT('Ctrl Pts',(-9.97765261724218,21.166403637904,-6.98236283400452));
#5997=CARTESIAN_POINT('Ctrl Pts',(-9.80119115426147,21.1780743367771,-7.22184894660825));
#5998=CARTESIAN_POINT('Ctrl Pts',(-9.63264179299859,21.1892217499704,-7.45059708588386));
#5999=CARTESIAN_POINT('Ctrl Pts',(-9.45605571647231,21.2003691631638,-7.67347617436341));
#6000=CARTESIAN_POINT('Ctrl Pts',(-9.27186695090699,21.2115165763572,-7.88992607662954));
#6001=CARTESIAN_POINT('Ctrl Pts',(-9.08770945043724,21.2226620973345,-8.10633923763807));
#6002=CARTESIAN_POINT('Ctrl Pts',(-8.89595201024563,21.2338076183118,-8.31632518819218));
#6003=CARTESIAN_POINT('Ctrl Pts',(-8.69706869375794,21.2449531392891,-8.51935715802874));
#6004=CARTESIAN_POINT('Ctrl Pts',(-8.49820744079386,21.2560974238155,-8.72236660410243));
#6005=CARTESIAN_POINT('Ctrl Pts',(-8.29222207669095,21.2672417083419,-8.91842341943104));
#6006=CARTESIAN_POINT('Ctrl Pts',(-8.07962411441024,21.2783859928682,-9.10703708237979));
#6007=CARTESIAN_POINT('Ctrl Pts',(-7.86033469976557,21.2898810401594,-9.30158729959874));
#6008=CARTESIAN_POINT('Ctrl Pts',(-7.63400990204134,21.3013760874505,-9.48821803027954));
#6009=CARTESIAN_POINT('Ctrl Pts',(-7.40124976128749,21.3128711347417,-9.66643430749115));
#6010=CARTESIAN_POINT('Ctrl Pts',(-7.17558004674712,21.3240160156153,-9.83922169400216));
#6011=CARTESIAN_POINT('Ctrl Pts',(-6.94386147980823,21.3351608964889,-10.0040995187547));
#6012=CARTESIAN_POINT('Ctrl Pts',(-6.70667300845964,21.3463057773625,-10.1606588077545));
#6013=CARTESIAN_POINT('Ctrl Pts',(-6.45830602768054,21.3579759078624,-10.3245966151054));
#6014=CARTESIAN_POINT('Ctrl Pts',(-6.20394142385836,21.3696460383624,-10.4794127629059));
#6015=CARTESIAN_POINT('Ctrl Pts',(-5.94427710028753,21.3813161688623,-10.6246891721592));
#6016=CARTESIAN_POINT('Ctrl Pts',(-5.68461277671671,21.3929862993622,-10.7699655814125));
#6017=CARTESIAN_POINT('Ctrl Pts',(-5.41964903042489,21.4046564298622,-10.9057020959921));
#6018=CARTESIAN_POINT('Ctrl Pts',(-5.15011341352574,21.4163265603621,-11.031535798692));
#6019=CARTESIAN_POINT('Ctrl Pts',(-4.89265384818702,21.4274738319566,-11.1517317519199));
#6020=CARTESIAN_POINT('Ctrl Pts',(-4.63094619394671,21.4386211035511,-11.262928642111));
#6021=CARTESIAN_POINT('Ctrl Pts',(-4.36563958289154,21.4497683751456,-11.3648423342469));
#6022=CARTESIAN_POINT('Ctrl Pts',(-4.10037804211338,21.460913753042,-11.4667387132886));
#6023=CARTESIAN_POINT('Ctrl Pts',(-3.83151901407759,21.4720591309384,-11.5593549471958));
#6024=CARTESIAN_POINT('Ctrl Pts',(-3.55973082007956,21.4832045088348,-11.6424553569501));
#6025=CARTESIAN_POINT('Ctrl Pts',(-3.28797280464175,21.4943486491813,-11.7255465394797));
#6026=CARTESIAN_POINT('Ctrl Pts',(-3.01328652773389,21.5054927895278,-11.7991239297607));
#6027=CARTESIAN_POINT('Ctrl Pts',(-2.73635584774457,21.5166369298742,-11.8630015984368));
#6028=CARTESIAN_POINT('Ctrl Pts',(-2.45070250392632,21.5281320843803,-11.9288912631476));
#6029=CARTESIAN_POINT('Ctrl Pts',(-2.16266136567062,21.5396272388864,-11.9844601901464));
#6030=CARTESIAN_POINT('Ctrl Pts',(-1.87299620102137,21.5511223933925,-12.0295609014195));
#6031=CARTESIAN_POINT('Ctrl Pts',(-1.59216120034856,21.5622671291682,-12.0732867608822));
#6032=CARTESIAN_POINT('Ctrl Pts',(-1.30979999634929,21.573411864944,-12.1071731361329));
#6033=CARTESIAN_POINT('Ctrl Pts',(-1.02661663648201,21.5845566007197,-12.1311379734837));
#6034=CARTESIAN_POINT('Ctrl Pts',(-0.730077273105364,21.596226964591,-12.156233083644));
#6035=CARTESIAN_POINT('Ctrl Pts',(-0.432636652240616,21.6078973284622,-12.1704482314372));
#6036=CARTESIAN_POINT('Ctrl Pts',(-0.135107706832327,21.6195676923335,-12.1737502914079));
#6037=CARTESIAN_POINT('Ctrl Pts',(0.162421238575963,21.6312380562048,-12.1770523513786));
#6038=CARTESIAN_POINT('Ctrl Pts',(0.460038172932362,21.642908420076,-12.1694413285824));
#6039=CARTESIAN_POINT('Ctrl Pts',(0.756930527455535,21.6545787839473,-12.1509467296423));
#6040=CARTESIAN_POINT('Ctrl Pts',(1.04051646831786,21.665726093968,-12.1332810398346));
#6041=CARTESIAN_POINT('Ctrl Pts',(1.3235260540737,21.6768734039887,-12.1056806331005));
#6042=CARTESIAN_POINT('Ctrl Pts',(1.60525332965216,21.6880207140093,-12.06820666038));
#6043=CARTESIAN_POINT('Ctrl Pts',(1.88693275396258,21.6991661306637,-12.0307390525992));
#6044=CARTESIAN_POINT('Ctrl Pts',(2.16733003861535,21.7103115473181,-11.983401262163));
#6045=CARTESIAN_POINT('Ctrl Pts',(2.44574556760614,21.7214569639726,-11.9263061703335));
#6046=CARTESIAN_POINT('Ctrl Pts',(2.72413018796549,21.7326011433053,-11.8692174169836));
#6047=CARTESIAN_POINT('Ctrl Pts',(3.00053323073995,21.743745322638,-11.8023735788287));
#6048=CARTESIAN_POINT('Ctrl Pts',(3.27426524481732,21.7548895019707,-11.7259386556719));
#6049=CARTESIAN_POINT('Ctrl Pts',(3.55661747114543,21.7663846274342,-11.6470966875694));
#6050=CARTESIAN_POINT('Ctrl Pts',(3.83612742536485,21.7778797528976,-11.5580498424948));
#6051=CARTESIAN_POINT('Ctrl Pts',(4.11205390419272,21.7893748783611,-11.4590341189392));
#6052=CARTESIAN_POINT('Ctrl Pts',(4.37957064322381,21.8005196532004,-11.3630362154727));
#6053=CARTESIAN_POINT('Ctrl Pts',(4.64371884535662,21.8116644280397,-11.2576681964017));
#6054=CARTESIAN_POINT('Ctrl Pts',(4.90384104113907,21.8228092028791,-11.1431949320309));
#6055=CARTESIAN_POINT('Ctrl Pts',(5.1762291608586,21.8344795036546,-11.0233237416994));
#6056=CARTESIAN_POINT('Ctrl Pts',(5.44420215910206,21.8461498044302,-10.8934680664645));
#6057=CARTESIAN_POINT('Ctrl Pts',(5.70703039091337,21.8578201052057,-10.7539878355516));
#6058=CARTESIAN_POINT('Ctrl Pts',(5.96985862272468,21.8694904059813,-10.6145076046387));
#6059=CARTESIAN_POINT('Ctrl Pts',(6.22754179586538,21.8811607067569,-10.465402983073));
#6060=CARTESIAN_POINT('Ctrl Pts',(6.47938055605088,21.8928310075324,-10.3070887189288));
#6061=CARTESIAN_POINT('Ctrl Pts',(6.71993349237776,21.9039783190793,-10.1558691009707));
#6062=CARTESIAN_POINT('Ctrl Pts',(6.95522616261537,21.9151256306262,-9.9962019716106));
#6063=CARTESIAN_POINT('Ctrl Pts',(7.18466795616308,21.9262729421732,-9.82847885533074));
#6064=CARTESIAN_POINT('Ctrl Pts',(7.41407078071216,21.9374183604313,-9.66078422558678));
#6065=CARTESIAN_POINT('Ctrl Pts',(7.6376244972866,21.9485637786895,-9.48503649799234));
#6066=CARTESIAN_POINT('Ctrl Pts',(7.85476881658421,21.9597091969477,-9.30166958604832));
#6067=CARTESIAN_POINT('Ctrl Pts',(8.07188903077369,21.9708533779572,-9.11832302959531));
#6068=CARTESIAN_POINT('Ctrl Pts',(8.28260106469835,21.9819975589667,-8.92735914978249));
#6069=CARTESIAN_POINT('Ctrl Pts',(8.48637801690925,21.9931417399762,-8.72925188112472));
#6070=CARTESIAN_POINT('Ctrl Pts',(8.69657214291512,22.004636864238,-8.52490598361697));
#6071=CARTESIAN_POINT('Ctrl Pts',(8.89938710238414,22.0161319884998,-8.31295969955983));
#6072=CARTESIAN_POINT('Ctrl Pts',(9.09428500702047,22.0276271127616,-8.09397494813783));
#6073=CARTESIAN_POINT('Ctrl Pts',(9.28324282708307,22.0387718894379,-7.88166439850486));
#6074=CARTESIAN_POINT('Ctrl Pts',(9.46475885166343,22.0499166661142,-7.66273827282285));
#6075=CARTESIAN_POINT('Ctrl Pts',(9.63838253212706,22.0610614427905,-7.43774377176224));
#6076=CARTESIAN_POINT('Ctrl Pts',(9.82019327263628,22.072731740845,-7.20213986831372));
#6077=CARTESIAN_POINT('Ctrl Pts',(9.99334925383761,22.0844020388995,-6.95988177403458));
#6078=CARTESIAN_POINT('Ctrl Pts',(10.1573820426963,22.096072336954,-6.71163469571394));
#6079=CARTESIAN_POINT('Ctrl Pts',(10.3214148315549,22.1077426350085,-6.4633876173933));
#6080=CARTESIAN_POINT('Ctrl Pts',(10.4763242504391,22.119412933063,-6.20915183978187));
#6081=CARTESIAN_POINT('Ctrl Pts',(10.6216946965625,22.1310832311175,-5.94962620868038));
#6082=CARTESIAN_POINT('Ctrl Pts',(10.7605504536662,22.142230531791,-5.70173106248379));
#6083=CARTESIAN_POINT('Ctrl Pts',(10.8907448834759,22.1533778324646,-5.44893572672565));
#6084=CARTESIAN_POINT('Ctrl Pts',(11.0119467530863,22.1645251331381,-5.19186661589001));
#6085=CARTESIAN_POINT('Ctrl Pts',(11.133128035799,22.1756705403727,-4.934841169855));
#6086=CARTESIAN_POINT('Ctrl Pts',(11.2453196941389,22.1868159476073,-4.67354363924085));
#6087=CARTESIAN_POINT('Ctrl Pts',(11.3482374041766,22.197961354842,-4.4086231488355));
#6088=CARTESIAN_POINT('Ctrl Pts',(11.4511436882337,22.2091055247073,-4.14373207004823));
#6089=CARTESIAN_POINT('Ctrl Pts',(11.5447779833639,22.2202496945727,-3.87521908322539));
#6090=CARTESIAN_POINT('Ctrl Pts',(11.6289044340636,22.2313938644381,-3.6037524767131));
#6091=CARTESIAN_POINT('Ctrl Pts',(11.7156802739048,22.2428889969602,-3.3237365890463));
#6092=CARTESIAN_POINT('Ctrl Pts',(11.7923396078497,22.2543841294822,-3.04057831121402));
#6093=CARTESIAN_POINT('Ctrl Pts',(11.8586790366335,22.2658792620042,-2.75502844923766));
#6094=CARTESIAN_POINT('Ctrl Pts',(11.9229964655406,22.2770240273771,-2.47818203551679));
#6095=CARTESIAN_POINT('Ctrl Pts',(11.9776137036275,22.2881687927499,-2.19908793968402));
#6096=CARTESIAN_POINT('Ctrl Pts',(12.0223969991252,22.2993135581228,-1.91844224448522));
#6097=CARTESIAN_POINT('Ctrl Pts',(12.0692921285266,22.3109838742194,-1.62456221520135));
#6098=CARTESIAN_POINT('Ctrl Pts',(12.1054034747324,22.322654190316,-1.32898104250092));
#6099=CARTESIAN_POINT('Ctrl Pts',(12.1306380526509,22.3343245064127,-1.03250699057074));
#6100=CARTESIAN_POINT('Ctrl Pts',(12.1558726305694,22.3459948225093,-0.736032938640579));
#6101=CARTESIAN_POINT('Ctrl Pts',(12.1702304204935,22.3576651386059,-0.43866634252017));
#6102=CARTESIAN_POINT('Ctrl Pts',(12.1736809240298,22.3693354547026,-0.14121972211462));
#6103=CARTESIAN_POINT('Ctrl Pts',(12.1769767929329,22.3804827645107,0.142896800657586));
#6104=CARTESIAN_POINT('Ctrl Pts',(12.1703224929076,22.3916300743188,0.427171187125004));
#6105=CARTESIAN_POINT('Ctrl Pts',(12.1537269468445,22.4027773841269,0.710894894865639));
#6106=CARTESIAN_POINT('Ctrl Pts',(12.1371342194696,22.4139228006082,0.99457041324932));
#6107=CARTESIAN_POINT('Ctrl Pts',(12.11060363268,22.4250682170895,1.2776951734493));
#6108=CARTESIAN_POINT('Ctrl Pts',(12.074196166311,22.4362136335708,1.55956313993394));
#6109=CARTESIAN_POINT('Ctrl Pts',(12.0377927416301,22.4473578127703,1.84139981551791));
#6110=CARTESIAN_POINT('Ctrl Pts',(11.9915146609846,22.4585019919697,2.12197971150438));
#6111=CARTESIAN_POINT('Ctrl Pts',(11.9354746331794,22.4696461711692,2.40060315977681));
#6112=CARTESIAN_POINT('Ctrl Pts',(11.8776698234813,22.4811412967624,2.68800086523175));
#6113=CARTESIAN_POINT('Ctrl Pts',(11.8094783169454,22.4926364223556,2.97331661069409));
#6114=CARTESIAN_POINT('Ctrl Pts',(11.7310808084977,22.5041315479488,3.25579380712257));
#6115=CARTESIAN_POINT('Ctrl Pts',(11.6550727153316,22.5152763227554,3.52966160583902));
#6116=CARTESIAN_POINT('Ctrl Pts',(11.5694716039288,22.5264210975619,3.80086105222759));
#6117=CARTESIAN_POINT('Ctrl Pts',(11.474493137458,22.5375658723685,4.06871693392769));
#6118=CARTESIAN_POINT('Ctrl Pts',(11.3750360097731,22.549236173355,4.34920342331078));
#6119=CARTESIAN_POINT('Ctrl Pts',(11.2652959853262,22.5609064743416,4.62602313302054));
#6120=CARTESIAN_POINT('Ctrl Pts',(11.1455782047075,22.5725767753281,4.89842186145174));
#6121=CARTESIAN_POINT('Ctrl Pts',(11.0258604240889,22.5842470763146,5.17082058988296));
#6122=CARTESIAN_POINT('Ctrl Pts',(10.8961650303231,22.5959173773012,5.43879803342295));
#6123=CARTESIAN_POINT('Ctrl Pts',(10.7568540674013,22.6075876782877,5.7016261559867));
#6124=CARTESIAN_POINT('Ctrl Pts',(10.6237862289835,22.6187349828027,5.95267581791911));
#6125=CARTESIAN_POINT('Ctrl Pts',(10.4819059659421,22.6298822873177,6.19910251958811));
#6126=CARTESIAN_POINT('Ctrl Pts',(10.331560180348,22.6410295918327,6.44028838561183));
#6127=CARTESIAN_POINT('Ctrl Pts',(10.1812399312278,22.65217500296,6.68143328582792));
#6128=CARTESIAN_POINT('Ctrl Pts',(10.0224571713425,22.6633204140874,6.91733890132951));
#6129=CARTESIAN_POINT('Ctrl Pts',(9.85560331246676,22.6744658252148,7.14741446939341));
#6130=CARTESIAN_POINT('Ctrl Pts',(9.68876797717991,22.6856099990138,7.37746449519373));
#6131=CARTESIAN_POINT('Ctrl Pts',(9.51386348869,22.6967541728128,7.60168555009451));
#6132=CARTESIAN_POINT('Ctrl Pts',(9.33132363306449,22.7078983466118,7.81951721687548));
#6133=CARTESIAN_POINT('Ctrl Pts',(9.14303517522486,22.7193934762168,8.04420890662334));
#6134=CARTESIAN_POINT('Ctrl Pts',(8.9466228297042,22.7308886058219,8.26210202013036));
#6135=CARTESIAN_POINT('Ctrl Pts',(8.74260731912758,22.742383735427,8.47261869279722));
#6136=CARTESIAN_POINT('Ctrl Pts',(8.54481000069478,22.7535285047855,8.67671902429267));
#6137=CARTESIAN_POINT('Ctrl Pts',(8.33986632224162,22.7646732741439,8.87388570935947));
#6138=CARTESIAN_POINT('Ctrl Pts',(8.12828876731127,22.7758180435024,9.0636290725736));
#6139=CARTESIAN_POINT('Ctrl Pts',(7.90673410626821,22.7874883532308,9.26231993340673));
#6140=CARTESIAN_POINT('Ctrl Pts',(7.67790509962432,22.7991586629592,9.45287030906345));
#6141=CARTESIAN_POINT('Ctrl Pts',(7.44243059986118,22.8108289726876,9.63476398342222));
#6142=CARTESIAN_POINT('Ctrl Pts',(7.20695610009804,22.822499282416,9.81665765778099));
#6143=CARTESIAN_POINT('Ctrl Pts',(6.96483637809425,22.8341695921444,9.98989443269214));
#6144=CARTESIAN_POINT('Ctrl Pts',(6.71673773003182,22.8458399018728,10.1540082980056));
#6145=CARTESIAN_POINT('Ctrl Pts',(6.47975894975053,22.8569871442562,10.3107665227399));
#6146=CARTESIAN_POINT('Ctrl Pts',(6.23725464023926,22.8681343866396,10.4592484615104));
#6147=CARTESIAN_POINT('Ctrl Pts',(5.98982507339607,22.879281629023,10.5990775938341));
#6148=CARTESIAN_POINT('Ctrl Pts',(5.74243799903203,22.8904269570274,10.7388827125099));
#6149=CARTESIAN_POINT('Ctrl Pts',(5.49012758823057,22.9015722850318,10.8700378604094));
#6150=CARTESIAN_POINT('Ctrl Pts',(5.2335202165415,22.9127176130361,10.9922116242843));
#6151=CARTESIAN_POINT('Ctrl Pts',(4.97694181572515,22.9238616827373,11.1143715947887));
#6152=CARTESIAN_POINT('Ctrl Pts',(4.71606766354038,22.9350057524385,11.2275520914857));
#6153=CARTESIAN_POINT('Ctrl Pts',(4.4515468169242,22.9461498221397,11.3314686244428));
#6154=CARTESIAN_POINT('Ctrl Pts',(4.18701646107352,22.957294292458,11.4353888930854));
#6155=CARTESIAN_POINT('Ctrl Pts',(3.91883939619725,22.9684387627762,11.5300444326363));
#6156=CARTESIAN_POINT('Ctrl Pts',(3.64768399310814,22.9795832330945,11.6151991690381));
#6157=CARTESIAN_POINT('Ctrl Pts',(3.3765343878357,22.9907274651229,11.7003520846701));
#6158=CARTESIAN_POINT('Ctrl Pts',(3.10240682663631,23.0018716971513,11.7760045248472));
#6159=CARTESIAN_POINT('Ctrl Pts',(2.82598510932383,23.0130159291796,11.8419702081993));
#6160=CARTESIAN_POINT('Ctrl Pts',(2.54952132601668,23.0241618571428,11.9079459302419));
#6161=CARTESIAN_POINT('Ctrl Pts',(2.27076294842339,23.0353077851059,11.9642318876258));
#6162=CARTESIAN_POINT('Ctrl Pts',(1.99040570099081,23.0464537130691,12.0106925443733));
#6163=CARTESIAN_POINT('Ctrl Pts',(1.85753271828706,23.0517362328078,12.0327121857307));
#6164=CARTESIAN_POINT('Ctrl Pts',(1.72430074052143,23.0570187525466,12.0525256043933));
#6165=CARTESIAN_POINT('Ctrl Pts',(1.59078448392772,23.0623012722853,12.0701224093086));
#6166=CARTESIAN_POINT('Ctrl Pts',(1.59078448392775,20.0623165459775,12.0701224093086));
#6167=CARTESIAN_POINT('Ctrl Pts',(1.30962621197678,20.073437407519,12.1071777266766));
#6168=CARTESIAN_POINT('Ctrl Pts',(1.02715337834117,20.0845582690605,12.134407435356));
#6169=CARTESIAN_POINT('Ctrl Pts',(0.744068298005909,20.0956791306019,12.1517411352408));
#6170=CARTESIAN_POINT('Ctrl Pts',(0.460962936440192,20.1068007888818,12.169076076974));
#6171=CARTESIAN_POINT('Ctrl Pts',(0.177245508869123,20.1179224471617,12.1765135734054));
#6172=CARTESIAN_POINT('Ctrl Pts',(-0.106378153026004,20.1290441054415,12.1740352364596));
#6173=CARTESIAN_POINT('Ctrl Pts',(-0.389997569760771,20.1401655972571,12.1715569366084));
#6174=CARTESIAN_POINT('Ctrl Pts',(-0.673522954588797,20.1512870890726,12.1591631043686));
#6175=CARTESIAN_POINT('Ctrl Pts',(-0.956249174934971,20.1624085808882,12.1368874826059));
#6176=CARTESIAN_POINT('Ctrl Pts',(-1.23904168428342,20.1735326802885,12.1146066380212));
#6177=CARTESIAN_POINT('Ctrl Pts',(-1.52103438623292,20.1846567796889,12.0824393934102));
#6178=CARTESIAN_POINT('Ctrl Pts',(-1.80152635112408,20.1957808790892,12.040471463203));
#6179=CARTESIAN_POINT('Ctrl Pts',(-2.0476611742289,20.205542400205,12.0036441370383));
#6180=CARTESIAN_POINT('Ctrl Pts',(-2.29264034845842,20.2153039213208,11.9592708188833));
#6181=CARTESIAN_POINT('Ctrl Pts',(-2.53599567615223,20.2250654424367,11.90744205027));
#6182=CARTESIAN_POINT('Ctrl Pts',(-2.81389961659165,20.2362127849193,11.8482552670495));
#6183=CARTESIAN_POINT('Ctrl Pts',(-3.08977208840519,20.2473601274019,11.7793265425913));
#6184=CARTESIAN_POINT('Ctrl Pts',(-3.36292380790852,20.2585074698845,11.7008202153611));
#6185=CARTESIAN_POINT('Ctrl Pts',(-3.63602920899081,20.2696529221088,11.6223272004729));
#6186=CARTESIAN_POINT('Ctrl Pts',(-3.9064145225981,20.2807983743331,11.5342598989375));
#6187=CARTESIAN_POINT('Ctrl Pts',(-4.17340434525476,20.2919438265575,11.4368328841952));
#6188=CARTESIAN_POINT('Ctrl Pts',(-4.44036459984117,20.3030880444669,11.3394166591106));
#6189=CARTESIAN_POINT('Ctrl Pts',(-4.70392986384737,20.3142322623763,11.2326428820652));
#6190=CARTESIAN_POINT('Ctrl Pts',(-4.96344230817149,20.3253764802858,11.1167751935286));
#6191=CARTESIAN_POINT('Ctrl Pts',(-5.23112562292012,20.3368715790971,10.9972593567428));
#6192=CARTESIAN_POINT('Ctrl Pts',(-5.49449649858255,20.3483666779084,10.8680677908843));
#6193=CARTESIAN_POINT('Ctrl Pts',(-5.75285652074247,20.3598617767198,10.729542958661));
#6194=CARTESIAN_POINT('Ctrl Pts',(-6.00334380137742,20.3710065971057,10.5952392524066));
#6195=CARTESIAN_POINT('Ctrl Pts',(-6.24912084279441,20.3821514174917,10.4521627969435));
#6196=CARTESIAN_POINT('Ctrl Pts',(-6.48957628823942,20.3932962378776,10.3006723008317));
#6197=CARTESIAN_POINT('Ctrl Pts',(-6.74136789952962,20.4049664759016,10.1420398521444));
#6198=CARTESIAN_POINT('Ctrl Pts',(-6.98732380660484,20.4166367139257,9.97418109459459));
#6199=CARTESIAN_POINT('Ctrl Pts',(-7.22677526496643,20.4283069519497,9.79755936545778));
#6200=CARTESIAN_POINT('Ctrl Pts',(-7.46622672332803,20.4399771899737,9.62093763632096));
#6201=CARTESIAN_POINT('Ctrl Pts',(-7.69917346821445,20.4516474279977,9.43555314181044));
#6202=CARTESIAN_POINT('Ctrl Pts',(-7.9249847794445,20.4633176660218,9.24191898339155));
#6203=CARTESIAN_POINT('Ctrl Pts',(-8.14066853729478,20.474464498208,9.05696924500836));
#6204=CARTESIAN_POINT('Ctrl Pts',(-8.34990739550198,20.4856113303942,8.86443818228698));
#6205=CARTESIAN_POINT('Ctrl Pts',(-8.55217478046388,20.4967581625804,8.66479986926402));
#6206=CARTESIAN_POINT('Ctrl Pts',(-8.75440768931906,20.5079030948094,8.46519558422725));
#6207=CARTESIAN_POINT('Ctrl Pts',(-8.9496713075049,20.5190480270384,8.25848665482182));
#6208=CARTESIAN_POINT('Ctrl Pts',(-9.13747528589881,20.5301929592674,8.04518462495352));
#6209=CARTESIAN_POINT('Ctrl Pts',(-9.3252583249383,20.5413366488833,7.83190637736524));
#6210=CARTESIAN_POINT('Ctrl Pts',(-9.5055832087329,20.5524803384992,7.61203669738287));
#6211=CARTESIAN_POINT('Ctrl Pts',(-9.67799849801041,20.5636240281151,7.38612180528512));
#6212=CARTESIAN_POINT('Ctrl Pts',(-9.85585682286771,20.5751195165727,7.15307493086235));
#6213=CARTESIAN_POINT('Ctrl Pts',(-10.0252978522716,20.5866150050304,6.91359518794776));
#6214=CARTESIAN_POINT('Ctrl Pts',(-10.1858721211816,20.598110493488,6.66831758248921));
#6215=CARTESIAN_POINT('Ctrl Pts',(-10.3415405228375,20.6092547716255,6.43053370177853));
#6216=CARTESIAN_POINT('Ctrl Pts',(-10.4888757631469,20.620399049763,6.18730120579808));
#6217=CARTESIAN_POINT('Ctrl Pts',(-10.6275127035771,20.6315433279005,5.93922755796635));
#6218=CARTESIAN_POINT('Ctrl Pts',(-10.7727033288179,20.6432144215182,5.67942690221995));
#6219=CARTESIAN_POINT('Ctrl Pts',(-10.9083532859157,20.654885515136,5.41431662760413));
#6220=CARTESIAN_POINT('Ctrl Pts',(-11.0340969861489,20.6665566087537,5.14462379093558));
#6221=CARTESIAN_POINT('Ctrl Pts',(-11.159840686382,20.6782277023714,4.87493095426703));
#6222=CARTESIAN_POINT('Ctrl Pts',(-11.2756779958382,20.6898987959892,4.60065586355721));
#6223=CARTESIAN_POINT('Ctrl Pts',(-11.3813005554201,20.7015698896069,4.32255108902081));
#6224=CARTESIAN_POINT('Ctrl Pts',(-11.4819409370545,20.7126904619584,4.05756441614999));
#6225=CARTESIAN_POINT('Ctrl Pts',(-11.5733394354702,20.7238110343099,3.7890178396337));
#6226=CARTESIAN_POINT('Ctrl Pts',(-11.6552609185346,20.7349316066614,3.51757632054809));
#6227=CARTESIAN_POINT('Ctrl Pts',(-11.7411699266226,20.7465934724425,3.23292239600646));
#6228=CARTESIAN_POINT('Ctrl Pts',(-11.8166563253145,20.7582553382236,2.94508500430039));
#6229=CARTESIAN_POINT('Ctrl Pts',(-11.8815075908379,20.7699172040048,2.65484982981369));
#6230=CARTESIAN_POINT('Ctrl Pts',(-11.9433326930578,20.7810348905784,2.37815793821194));
#6231=CARTESIAN_POINT('Ctrl Pts',(-11.995492397791,20.792152577152,2.09928720024168));
#6232=CARTESIAN_POINT('Ctrl Pts',(-12.0378545291329,20.8032702637256,1.81893061589332));
#6233=CARTESIAN_POINT('Ctrl Pts',(-12.0802138904517,20.8143872233234,1.53859236381978));
#6234=CARTESIAN_POINT('Ctrl Pts',(-12.1127769187808,20.8255041829211,1.25676872584638));
#6235=CARTESIAN_POINT('Ctrl Pts',(-12.1354629727721,20.8366211425188,0.974160503447343));
#6236=CARTESIAN_POINT('Ctrl Pts',(-12.1581504142312,20.8477387820242,0.691534996870884));
#6237=CARTESIAN_POINT('Ctrl Pts',(-12.1709596530285,20.8588564215296,0.408125078448854));
#6238=CARTESIAN_POINT('Ctrl Pts',(-12.1738620090751,20.869974061035,0.124635604858819));
#6239=CARTESIAN_POINT('Ctrl Pts',(-12.1742883992265,20.8716073727016,0.0829876755153614));
#6240=CARTESIAN_POINT('Ctrl Pts',(-12.1745010602666,20.8732406843683,0.0413380318515849));
#6241=CARTESIAN_POINT('Ctrl Pts',(-12.1744999960254,20.8748739960349,-0.000311089488517879));
#6242=CARTESIAN_POINT('',(-3.14788895504393,20.,11.7604951161383));
#6243=CARTESIAN_POINT('Origin',(0.,20.,0.));
#6244=CARTESIAN_POINT('',(-12.1737246773372,20.6251260039651,-0.000249401258526419));
#6245=CARTESIAN_POINT('Ctrl Pts',(-3.14788895504386,20.,11.7604951161383));
#6246=CARTESIAN_POINT('Ctrl Pts',(-5.10402892604601,20.0794174078617,11.2369022445433));
#6247=CARTESIAN_POINT('Ctrl Pts',(-8.7479903792511,20.2382522235851,9.19518133472436));
#6248=CARTESIAN_POINT('Ctrl Pts',(-11.6635919119852,20.4466275582401,4.5523794220281));
#6249=CARTESIAN_POINT('Ctrl Pts',(-12.1729512588234,20.5755854850334,1.26311059284835));
#6250=CARTESIAN_POINT('Ctrl Pts',(-12.1737246773372,20.6251260039651,-0.000249401258526419));
#6251=CARTESIAN_POINT('Ctrl Pts',(-12.1737246773372,20.6251260039651,-0.000249401258526419));
#6252=CARTESIAN_POINT('Ctrl Pts',(-12.1741911104616,20.6550028928951,-0.762156362199578));
#6253=CARTESIAN_POINT('Ctrl Pts',(-11.9165818304369,20.7642971896869,-3.54900219940989));
#6254=CARTESIAN_POINT('Ctrl Pts',(-9.8146932898574,20.9530088943404,-8.04643346012397));
#6255=CARTESIAN_POINT('Ctrl Pts',(-4.76736202235426,21.1912611179255,-11.7619196070543));
#6256=CARTESIAN_POINT('Ctrl Pts',(1.44252672235886,21.4295133415106,-12.6091655852676));
#6257=CARTESIAN_POINT('Ctrl Pts',(7.30065724870191,21.6677655650957,-10.3813184923891));
#6258=CARTESIAN_POINT('Ctrl Pts',(11.3783496330833,21.9060177886808,-5.62180304001539));
#6259=CARTESIAN_POINT('Ctrl Pts',(12.6811956770552,22.1442700122659,0.50872888397338));
#6260=CARTESIAN_POINT('Ctrl Pts',(10.8914562364704,22.382522235851,6.51518676137968));
#6261=CARTESIAN_POINT('Ctrl Pts',(6.73471108682879,22.605281261584,10.6455116559698));
#6262=CARTESIAN_POINT('Ctrl Pts',(3.2064497298399,22.7486228794554,11.8556871280485));
#6263=CARTESIAN_POINT('Ctrl Pts',(1.5908148051505,22.812547089465,12.070351758578));
#6264=CARTESIAN_POINT('Origin',(0.,13.3748739960349,0.));
#6265=CARTESIAN_POINT('',(1.59078448392775,26.0623070005467,12.0701224093086));
#6266=CARTESIAN_POINT('',(1.59078448392773,25.8125631998879,12.0701224093087));
#6267=CARTESIAN_POINT('',(1.59078448392774,13.3748739960349,12.0701224093086));
#6268=CARTESIAN_POINT('',(-12.1744999967658,23.8748739960011,0.000280623926547941));
#6269=CARTESIAN_POINT('Ctrl Pts',(-12.1744999967658,23.8748739960349,0.00028062306491734));
#6270=CARTESIAN_POINT('Ctrl Pts',(-12.1745065428157,23.8860100974646,-0.283712015376132));
#6271=CARTESIAN_POINT('Ctrl Pts',(-12.1645717688562,23.8971461988943,-0.567720156626778));
#6272=CARTESIAN_POINT('Ctrl Pts',(-12.1447184939399,23.908282300324,-0.8510363993127));
#6273=CARTESIAN_POINT('Ctrl Pts',(-12.1248634023349,23.9194194207708,-1.13437856706043));
#6274=CARTESIAN_POINT('Ctrl Pts',(-12.0950880117066,23.9305565412177,-1.41702844262597));
#6275=CARTESIAN_POINT('Ctrl Pts',(-12.0554671639295,23.9416936616646,-1.6982819876032));
#6276=CARTESIAN_POINT('Ctrl Pts',(-12.0158465226463,23.9528307240675,-1.97953406675724));
#6277=CARTESIAN_POINT('Ctrl Pts',(-11.9663805663668,23.9639677864705,-2.25938956526504));
#6278=CARTESIAN_POINT('Ctrl Pts',(-11.9071957223858,23.9751048488735,-2.53715200151623));
#6279=CARTESIAN_POINT('Ctrl Pts',(-11.8479967642311,23.9862445672002,-2.81498067748367));
#6280=CARTESIAN_POINT('Ctrl Pts',(-11.7790743410825,23.9973842855269,-3.09071503164591));
#6281=CARTESIAN_POINT('Ctrl Pts',(-11.7006058479935,24.0085240038537,-3.36366957947735));
#6282=CARTESIAN_POINT('Ctrl Pts',(-11.6335067433188,24.0180496758352,-3.59707543519565));
#6283=CARTESIAN_POINT('Ctrl Pts',(-11.5594283093542,24.0275753478167,-3.82844876548518));
#6284=CARTESIAN_POINT('Ctrl Pts',(-11.4785103889095,24.0371010197983,-4.05736977630798));
#6285=CARTESIAN_POINT('Ctrl Pts',(-11.3838171384972,24.0482483260728,-4.32526191297343));
#6286=CARTESIAN_POINT('Ctrl Pts',(-11.2797273169031,24.0593956323473,-4.58987760285483));
#6287=CARTESIAN_POINT('Ctrl Pts',(-11.1664931690163,24.0705429386218,-4.85055466481025));
#6288=CARTESIAN_POINT('Ctrl Pts',(-11.053278253932,24.081688351528,-5.11118745080703));
#6289=CARTESIAN_POINT('Ctrl Pts',(-10.9309222196804,24.0928337644342,-5.36788269991822));
#6290=CARTESIAN_POINT('Ctrl Pts',(-10.7997253247509,24.1039791773405,-5.61999850177324));
#6291=CARTESIAN_POINT('Ctrl Pts',(-10.6685429947127,24.115123352933,-5.87208631486202));
#6292=CARTESIAN_POINT('Ctrl Pts',(-10.5285218869459,24.1262675285254,-6.11959545930329));
#6293=CARTESIAN_POINT('Ctrl Pts',(-10.3800086368805,24.1374117041179,-6.36190780727653));
#6294=CARTESIAN_POINT('Ctrl Pts',(-10.2268184035207,24.14890683239,-6.61185106227649));
#6295=CARTESIAN_POINT('Ctrl Pts',(-10.0645926378427,24.1604019606621,-6.85626464349746));
#6296=CARTESIAN_POINT('Ctrl Pts',(-9.89376139950918,24.1718970889342,-7.09450037843273));
#6297=CARTESIAN_POINT('Ctrl Pts',(-9.72813688326918,24.1830418601,-7.32547498667565));
#6298=CARTESIAN_POINT('Ctrl Pts',(-9.55442385726194,24.1941866312657,-7.55064253139713));
#6299=CARTESIAN_POINT('Ctrl Pts',(-9.37305720387854,24.2053314024315,-7.76944328139543));
#6300=CARTESIAN_POINT('Ctrl Pts',(-9.18313814126281,24.2170017092568,-7.99856165880439));
#6301=CARTESIAN_POINT('Ctrl Pts',(-8.98482646679887,24.2286720160821,-8.22069809174982));
#6302=CARTESIAN_POINT('Ctrl Pts',(-8.77866826149681,24.2403423229074,-8.43524948087421));
#6303=CARTESIAN_POINT('Ctrl Pts',(-8.57251005619474,24.2520126297327,-8.6498008699986));
#6304=CARTESIAN_POINT('Ctrl Pts',(-8.35850555884004,24.263682936558,-8.85676697946432));
#6305=CARTESIAN_POINT('Ctrl Pts',(-8.13724527165577,24.2753532433833,-9.05558886207384));
#6306=CARTESIAN_POINT('Ctrl Pts',(-7.92590068440107,24.2865005496194,-9.24550061375804));
#6307=CARTESIAN_POINT('Ctrl Pts',(-7.70787322336667,24.2976478558555,-9.42803877404122));
#6308=CARTESIAN_POINT('Ctrl Pts',(-7.48370125772818,24.3087951620916,-9.60274261526766));
#6309=CARTESIAN_POINT('Ctrl Pts',(-7.25956736767171,24.3199405749591,-9.77741678306721));
#6310=CARTESIAN_POINT('Ctrl Pts',(-7.02929126696434,24.3310859878265,-9.94425912456056));
#6311=CARTESIAN_POINT('Ctrl Pts',(-6.79344378337951,24.342231400694,-10.1028496876902));
#6312=CARTESIAN_POINT('Ctrl Pts',(-6.55762248253287,24.3533755762473,-10.2614226448012));
#6313=CARTESIAN_POINT('Ctrl Pts',(-6.31623125517515,24.3645197518006,-10.4117455039978));
#6314=CARTESIAN_POINT('Ctrl Pts',(-6.06987027004878,24.3756639273539,-10.5534413891762));
#6315=CARTESIAN_POINT('Ctrl Pts',(-5.81575087656889,24.3871590556551,-10.6995995658927));
#6316=CARTESIAN_POINT('Ctrl Pts',(-5.55634388989934,24.3986541839563,-10.836578445479));
#6317=CARTESIAN_POINT('Ctrl Pts',(-5.29233710829935,24.4101493122576,-10.9640146927172));
#6318=CARTESIAN_POINT('Ctrl Pts',(-5.03637692415595,24.4212940833839,-11.0875668420671));
#6319=CARTESIAN_POINT('Ctrl Pts',(-4.776093436397,24.4324388545102,-11.2021493190998));
#6320=CARTESIAN_POINT('Ctrl Pts',(-4.51213635499412,24.4435836256365,-11.3074787536365));
#6321=CARTESIAN_POINT('Ctrl Pts',(-4.2357322807886,24.4552539325252,-11.4177750362176));
#6322=CARTESIAN_POINT('Ctrl Pts',(-3.95530011241909,24.4669242394138,-11.517924499486));
#6323=CARTESIAN_POINT('Ctrl Pts',(-3.67160795292729,24.4785945463025,-11.6076589065152));
#6324=CARTESIAN_POINT('Ctrl Pts',(-3.38791579343547,24.4902648531912,-11.6973933135444));
#6325=CARTESIAN_POINT('Ctrl Pts',(-3.10096396534875,24.5019351600798,-11.7767125715228));
#6326=CARTESIAN_POINT('Ctrl Pts',(-2.81153844769576,24.5136054669685,-11.8454084694082));
#6327=CARTESIAN_POINT('Ctrl Pts',(-2.53508343133578,24.5247527732184,-11.9110257851439));
#6328=CARTESIAN_POINT('Ctrl Pts',(-2.25628900057298,24.5359000794684,-11.9669705731406));
#6329=CARTESIAN_POINT('Ctrl Pts',(-1.97584835600998,24.5470473857183,-12.0130959175415));
#6330=CARTESIAN_POINT('Ctrl Pts',(-1.6954553442541,24.5581927985997,-12.0592134275587));
#6331=CARTESIAN_POINT('Ctrl Pts',(-1.41341694004873,24.5693382114812,-12.0955147805296));
#6332=CARTESIAN_POINT('Ctrl Pts',(-1.13043533186683,24.5804836243626,-12.1219043970189));
#6333=CARTESIAN_POINT('Ctrl Pts',(-0.847485139039559,24.59162779993,-12.1482910838509));
#6334=CARTESIAN_POINT('Ctrl Pts',(-0.563592216852303,24.6027719754975,-12.1647682066768));
#6335=CARTESIAN_POINT('Ctrl Pts',(-0.279463903351351,24.6139161510649,-12.1712920504244));
#6336=CARTESIAN_POINT('Ctrl Pts',(0.0136121878273971,24.6254112793557,-12.178021343262));
#6337=CARTESIAN_POINT('Ctrl Pts',(0.306938440053928,24.6369064076464,-12.1741602840482));
#6338=CARTESIAN_POINT('Ctrl Pts',(0.599737050830368,24.6484015359371,-12.1597189819445));
#6339=CARTESIAN_POINT('Ctrl Pts',(0.883611525722312,24.6595463070775,-12.1457178326885));
#6340=CARTESIAN_POINT('Ctrl Pts',(1.16698976785634,24.670691078218,-12.1217718491366));
#6341=CARTESIAN_POINT('Ctrl Pts',(1.44916568538033,24.6818358493584,-12.0879431280229));
#6342=CARTESIAN_POINT('Ctrl Pts',(1.7446477106423,24.6935061562243,-12.0525192012952));
#6343=CARTESIAN_POINT('Ctrl Pts',(2.0388109751728,24.7051764630901,-12.006258099938));
#6344=CARTESIAN_POINT('Ctrl Pts',(2.33085267230887,24.716846769956,-11.9492918647923));
#6345=CARTESIAN_POINT('Ctrl Pts',(2.62289436944495,24.7285170768218,-11.8923256296465));
#6346=CARTESIAN_POINT('Ctrl Pts',(2.91281417157252,24.7401873836877,-11.8246543335607));
#6347=CARTESIAN_POINT('Ctrl Pts',(3.19982230071158,24.7518576905535,-11.7464712783827));
#6348=CARTESIAN_POINT('Ctrl Pts',(3.47396826343337,24.7630049968009,-11.6717919687945));
#6349=CARTESIAN_POINT('Ctrl Pts',(3.74553966481412,24.7741523030483,-11.587500048405));
#6350=CARTESIAN_POINT('Ctrl Pts',(4.01385752465415,24.7852996092957,-11.4937982417379));
#6351=CARTESIAN_POINT('Ctrl Pts',(4.28212981073978,24.7964450221745,-11.4001123503108));
#6352=CARTESIAN_POINT('Ctrl Pts',(4.54714940684029,24.8075904350533,-11.2970198514592));
#6353=CARTESIAN_POINT('Ctrl Pts',(4.80825400749799,24.8187358479322,-11.1847728474645));
#6354=CARTESIAN_POINT('Ctrl Pts',(5.06932962149008,24.8298800234971,-11.0725383046305));
#6355=CARTESIAN_POINT('Ctrl Pts',(5.32649086291784,24.841024199062,-10.9511513913509));
#6356=CARTESIAN_POINT('Ctrl Pts',(5.57909572397968,24.8521683746269,-10.8209122144425));
#6357=CARTESIAN_POINT('Ctrl Pts',(5.83965562527876,24.8636635029195,-10.6865715412747));
#6358=CARTESIAN_POINT('Ctrl Pts',(6.09536724836163,24.8751586312122,-10.5428121455003));
#6359=CARTESIAN_POINT('Ctrl Pts',(6.34555247030226,24.8866537595048,-10.390015115323));
#6360=CARTESIAN_POINT('Ctrl Pts',(6.58811235911965,24.8977985306427,-10.2418751478064));
#6361=CARTESIAN_POINT('Ctrl Pts',(6.82547749579582,24.9089433017806,-10.0852404450836));
#6362=CARTESIAN_POINT('Ctrl Pts',(7.05705760223552,24.9200880729185,-9.92050342718201));
#6363=CARTESIAN_POINT('Ctrl Pts',(7.29955795273287,24.9317583797885,-9.74799817534841));
#6364=CARTESIAN_POINT('Ctrl Pts',(7.53571429569325,24.9434286866585,-9.56660827088475));
#6365=CARTESIAN_POINT('Ctrl Pts',(7.76488490244142,24.9550989935286,-9.37683383140799));
#6366=CARTESIAN_POINT('Ctrl Pts',(7.99405550918959,24.9667693003986,-9.18705939193122));
#6367=CARTESIAN_POINT('Ctrl Pts',(8.21624012692051,24.9784396072687,-8.98890063818444));
#6368=CARTESIAN_POINT('Ctrl Pts',(8.43083778298808,24.9901099141387,-8.78290524410578));
#6369=CARTESIAN_POINT('Ctrl Pts',(8.63581832193552,25.0012572203849,-8.58614145985624));
#6370=CARTESIAN_POINT('Ctrl Pts',(8.83393818577717,25.0124045266311,-8.38216922295967));
#6371=CARTESIAN_POINT('Ctrl Pts',(9.02469819859376,25.0235518328773,-8.17149145959895));
#6372=CARTESIAN_POINT('Ctrl Pts',(9.21542581084571,25.0346972457549,-7.96084947983034));
#6373=CARTESIAN_POINT('Ctrl Pts',(9.39879588886446,25.0458426586325,-7.74350444513577));
#6374=CARTESIAN_POINT('Ctrl Pts',(9.57434752759173,25.0569880715101,-7.5199946589674));
#6375=CARTESIAN_POINT('Ctrl Pts',(9.74987967736235,25.0681322470739,-7.2965096858544));
#6376=CARTESIAN_POINT('Ctrl Pts',(9.91759495631258,25.0792764226377,-7.06686153759513));
#6377=CARTESIAN_POINT('Ctrl Pts',(10.0770732542511,25.0904205982015,-6.83162095541444));
#6378=CARTESIAN_POINT('Ctrl Pts',(10.2415738477981,25.101915726495,-6.58897216937083));
#6379=CARTESIAN_POINT('Ctrl Pts',(10.3973100804441,25.1134108547885,-6.34037324759497));
#6380=CARTESIAN_POINT('Ctrl Pts',(10.5438688836484,25.1249059830821,-6.0864833208045));
#6381=CARTESIAN_POINT('Ctrl Pts',(10.6859607575328,25.1360507542187,-5.84033164196093));
#6382=CARTESIAN_POINT('Ctrl Pts',(10.8194262115696,25.1471955253553,-5.58920695028821));
#6383=CARTESIAN_POINT('Ctrl Pts',(10.9439347333879,25.1583402964919,-5.3337362890704));
#6384=CARTESIAN_POINT('Ctrl Pts',(11.0743144998257,25.1700106033639,-5.06621881592986));
#6385=CARTESIAN_POINT('Ctrl Pts',(11.19487213416,25.1816809102359,-4.79393592517833));
#6386=CARTESIAN_POINT('Ctrl Pts',(11.3052834849987,25.1933512171079,-4.51763384680682));
#6387=CARTESIAN_POINT('Ctrl Pts',(11.4156948358375,25.2050215239798,-4.2413317684353));
#6388=CARTESIAN_POINT('Ctrl Pts',(11.5159597868368,25.2166918308518,-3.96101081724842));
#6389=CARTESIAN_POINT('Ctrl Pts',(11.6058127307487,25.2283621377238,-3.67743947724378));
#6390=CARTESIAN_POINT('Ctrl Pts',(11.6916389471497,25.2395094439717,-3.4065762853131));
#6391=CARTESIAN_POINT('Ctrl Pts',(11.7679914973803,25.2506567502196,-3.13266673460072));
#6392=CARTESIAN_POINT('Ctrl Pts',(11.834672744551,25.2618040564674,-2.85639130361768));
#6393=CARTESIAN_POINT('Ctrl Pts',(11.9013426659205,25.2729494693468,-2.58016279798063));
#6394=CARTESIAN_POINT('Ctrl Pts',(11.9583445012586,25.2840948822262,-2.30156947355845));
#6395=CARTESIAN_POINT('Ctrl Pts',(12.0055311474859,25.2952402951056,-2.02130455813741));
#6396=CARTESIAN_POINT('Ctrl Pts',(12.0527125552623,25.3063844706709,-1.7410707564762));
#6397=CARTESIAN_POINT('Ctrl Pts',(12.0900809054865,25.3175286462363,-1.45916599735268));
#6398=CARTESIAN_POINT('Ctrl Pts',(12.1175404384541,25.3286728218017,-1.17629246891674));
#6399=CARTESIAN_POINT('Ctrl Pts',(12.1458647278962,25.340167950094,-0.884510678439701));
#6400=CARTESIAN_POINT('Ctrl Pts',(12.163645951052,25.3516630783862,-0.591698407265157));
#6401=CARTESIAN_POINT('Ctrl Pts',(12.1708368293856,25.3631582066785,-0.29863208546831));
#6402=CARTESIAN_POINT('Ctrl Pts',(12.1778085387284,25.3743029778168,-0.0144980591447471));
#6403=CARTESIAN_POINT('Ctrl Pts',(12.1748258979266,25.3854477489552,0.269874481842067));
#6404=CARTESIAN_POINT('Ctrl Pts',(12.1618987628609,25.3965925200936,0.553776788898335));
#6405=CARTESIAN_POINT('Ctrl Pts',(12.148362044046,25.4082628269628,0.851066612358317));
#6406=CARTESIAN_POINT('Ctrl Pts',(12.1239204060494,25.419933133832,1.14784046916088));
#6407=CARTESIAN_POINT('Ctrl Pts',(12.088646326029,25.4316034407012,1.44328800112304));
#6408=CARTESIAN_POINT('Ctrl Pts',(12.0533722460086,25.4432737475704,1.73873553308519));
#6409=CARTESIAN_POINT('Ctrl Pts',(12.0072657724544,25.4549440544397,2.03285640811261));
#6410=CARTESIAN_POINT('Ctrl Pts',(11.9504614375384,25.4666143613089,2.32484874344699));
#6411=CARTESIAN_POINT('Ctrl Pts',(11.8962027685468,25.4777616675556,2.60375554685274));
#6412=CARTESIAN_POINT('Ctrl Pts',(11.832167798918,25.4889089738023,2.88080369527671));
#6413=CARTESIAN_POINT('Ctrl Pts',(11.7585086287844,25.5000562800489,3.15530110715318));
#6414=CARTESIAN_POINT('Ctrl Pts',(11.6848619696517,25.5112016929271,3.4297518956788));
#6415=CARTESIAN_POINT('Ctrl Pts',(11.6015944427383,25.5223471058052,3.70165255508999));
#6416=CARTESIAN_POINT('Ctrl Pts',(11.5089086211831,25.5334925186833,3.97032399172388));
#6417=CARTESIAN_POINT('Ctrl Pts',(11.4162330891935,25.5446366942475,4.23896560165561));
#6418=CARTESIAN_POINT('Ctrl Pts',(11.3141414373819,25.5557808698117,4.5043784525661));
#6419=CARTESIAN_POINT('Ctrl Pts',(11.2028856095872,25.5669250453759,4.76590015301466));
#6420=CARTESIAN_POINT('Ctrl Pts',(11.0881261097483,25.5784201736691,5.03565770311674));
#6421=CARTESIAN_POINT('Ctrl Pts',(10.9636159909716,25.5899153019623,5.30127477407346));
#6422=CARTESIAN_POINT('Ctrl Pts',(10.8296852946106,25.6014104302554,5.56204698557055));
#6423=CARTESIAN_POINT('Ctrl Pts',(10.6998366386309,25.6125552013926,5.81487118569636));
#6424=CARTESIAN_POINT('Ctrl Pts',(10.5611332838991,25.6236999725298,6.06314123540553));
#6425=CARTESIAN_POINT('Ctrl Pts',(10.4139230509799,25.6348447436669,6.30623952433371));
#6426=CARTESIAN_POINT('Ctrl Pts',(10.2597710660175,25.6465150505381,6.56080120144097));
#6427=CARTESIAN_POINT('Ctrl Pts',(10.0962907731105,25.6581853574093,6.80969135715406));
#6428=CARTESIAN_POINT('Ctrl Pts',(9.92393360285792,25.6698556642805,7.05223312831244));
#6429=CARTESIAN_POINT('Ctrl Pts',(9.75157643260539,25.6815259711516,7.29477489947081));
#6430=CARTESIAN_POINT('Ctrl Pts',(9.57034258650591,25.6931962780228,7.53096801767879));
#6431=CARTESIAN_POINT('Ctrl Pts',(9.38073392759741,25.704866584894,7.76017275771763));
#6432=CARTESIAN_POINT('Ctrl Pts',(9.1996225128482,25.7160138911413,7.97910576939877));
#6433=CARTESIAN_POINT('Ctrl Pts',(9.01081632348767,25.7271611973887,8.19172838519741));
#6434=CARTESIAN_POINT('Ctrl Pts',(8.81478010379239,25.738308503636,8.39750569941967));
#6435=CARTESIAN_POINT('Ctrl Pts',(8.61877718082369,25.7494539165148,8.60324806239169));
#6436=CARTESIAN_POINT('Ctrl Pts',(8.41554686318361,25.7605993293936,8.80214725200337));
#6437=CARTESIAN_POINT('Ctrl Pts',(8.20559199842654,25.7717447422724,8.99370392026324));
#6438=CARTESIAN_POINT('Ctrl Pts',(7.99566044192285,25.7828889178371,9.1852393227555));
#6439=CARTESIAN_POINT('Ctrl Pts',(7.77900602600686,25.7940330934018,9.36943365184792));
#6440=CARTESIAN_POINT('Ctrl Pts',(7.55616695615486,25.8051772689665,9.54582585116204));
#6441=CARTESIAN_POINT('Ctrl Pts',(7.32631023129463,25.8166723972593,9.72777299917411));
#6442=CARTESIAN_POINT('Ctrl Pts',(7.08987323231034,25.828167525552,9.90141845280155));
#6443=CARTESIAN_POINT('Ctrl Pts',(6.84748283278494,25.8396626538447,10.0663016597316));
#6444=CARTESIAN_POINT('Ctrl Pts',(6.612480189934,25.8508074249824,10.2261594324247));
#6445=CARTESIAN_POINT('Ctrl Pts',(6.37188190783972,25.8619521961202,10.3777810168315));
#6446=CARTESIAN_POINT('Ctrl Pts',(6.12628894824933,25.8730969672579,10.5207905583448));
#6447=CARTESIAN_POINT('Ctrl Pts',(5.86911496341343,25.8847672741281,10.6705437667506));
#6448=CARTESIAN_POINT('Ctrl Pts',(5.60646418974834,25.8964375809983,10.8108530211056));
#6449=CARTESIAN_POINT('Ctrl Pts',(5.33905692026464,25.9081078878685,10.9413400208646));
#6450=CARTESIAN_POINT('Ctrl Pts',(5.07164965078095,25.9197781947387,11.0718270206237));
#6451=CARTESIAN_POINT('Ctrl Pts',(4.79948619084612,25.9314485016088,11.1924916265437));
#6452=CARTESIAN_POINT('Ctrl Pts',(4.52331334430271,25.943118808479,11.3030122816554));
#6453=CARTESIAN_POINT('Ctrl Pts',(4.25951707437787,25.954266115174,11.4085799974284));
#6454=CARTESIAN_POINT('Ctrl Pts',(3.99198409131871,25.9654134218689,11.5049245009964));
#6455=CARTESIAN_POINT('Ctrl Pts',(3.72137844577119,25.9765607285639,11.5917985107295));
#6456=CARTESIAN_POINT('Ctrl Pts',(3.45082167223791,25.9877060220291,11.6786568308126));
#6457=CARTESIAN_POINT('Ctrl Pts',(3.17719359814242,25.9988513154943,11.7560479907674));
#6458=CARTESIAN_POINT('Ctrl Pts',(2.90117469334908,26.0099966089595,11.8237741710788));
#6459=CARTESIAN_POINT('Ctrl Pts',(2.62517723677871,26.0211410363727,11.8914950886848));
#6460=CARTESIAN_POINT('Ctrl Pts',(2.34678957918977,26.0322854637858,11.9495524615316));
#6461=CARTESIAN_POINT('Ctrl Pts',(2.06670498175388,26.043429891199,11.9977989968324));
#6462=CARTESIAN_POINT('Ctrl Pts',(1.90856353651569,26.0497222609815,12.025039969346));
#6463=CARTESIAN_POINT('Ctrl Pts',(1.749881326521,26.0560146307641,12.0491542053372));
#6464=CARTESIAN_POINT('Ctrl Pts',(1.59078448392775,26.0623070005467,12.0701224093086));
#6465=CARTESIAN_POINT('Ctrl Pts',(1.59078448392772,23.0623012722853,12.0701224093086));
#6466=CARTESIAN_POINT('Ctrl Pts',(1.40719576191192,23.0695648900095,12.0943185260093));
#6467=CARTESIAN_POINT('Ctrl Pts',(1.22306953313744,23.0768285077337,12.1143233119144));
#6468=CARTESIAN_POINT('Ctrl Pts',(1.03860091274412,23.0840921254579,12.1301178227603));
#6469=CARTESIAN_POINT('Ctrl Pts',(0.755501187515748,23.0952394315824,12.1543572932515));
#6470=CARTESIAN_POINT('Ctrl Pts',(0.471510238288568,23.1063867377068,12.1686853376153));
#6471=CARTESIAN_POINT('Ctrl Pts',(0.187335335693578,23.1175340438313,12.1730586017648));
#6472=CARTESIAN_POINT('Ctrl Pts',(-0.0967912998095614,23.1286794565864,
12.1774311231157));
#6473=CARTESIAN_POINT('Ctrl Pts',(-0.381101559686401,23.1398248693415,12.1718522358687));
#6474=CARTESIAN_POINT('Ctrl Pts',(-0.664886834336528,23.1509702820966,12.1563306860058));
#6475=CARTESIAN_POINT('Ctrl Pts',(-0.948640604399958,23.1621144575373,12.1408108592767));
#6476=CARTESIAN_POINT('Ctrl Pts',(-1.2318692393348,23.1732586329779,12.1153505885898));
#6477=CARTESIAN_POINT('Ctrl Pts',(-1.51386666477452,23.1844028084186,12.0800106776147));
#6478=CARTESIAN_POINT('Ctrl Pts',(-1.80474476760346,23.195897936804,12.0435578403501));
#6479=CARTESIAN_POINT('Ctrl Pts',(-2.09431256209703,23.2073930651893,11.9965930464181));
#6480=CARTESIAN_POINT('Ctrl Pts',(-2.38180219291559,23.2188881935747,11.9392407029854));
#6481=CARTESIAN_POINT('Ctrl Pts',(-2.66052949347102,23.2300329645888,11.8836363884227));
#6482=CARTESIAN_POINT('Ctrl Pts',(-2.93730316054589,23.2411777356028,11.8182684020138));
#6483=CARTESIAN_POINT('Ctrl Pts',(-3.21143391640613,23.2523225066169,11.743302025008));
#6484=CARTESIAN_POINT('Ctrl Pts',(-3.49849141578957,23.2639928136879,11.6648005790335));
#6485=CARTESIAN_POINT('Ctrl Pts',(-3.78265044479703,23.2756631207589,11.5757738130286));
#6486=CARTESIAN_POINT('Ctrl Pts',(-4.06313635096133,23.2873334278299,11.4764704174888));
#6487=CARTESIAN_POINT('Ctrl Pts',(-4.34362225712563,23.299003734901,11.3771670219491));
#6488=CARTESIAN_POINT('Ctrl Pts',(-4.62043472711151,23.310674041972,11.2675871171198));
#6489=CARTESIAN_POINT('Ctrl Pts',(-4.89282100638345,23.322344349043,11.1480380717637));
#6490=CARTESIAN_POINT('Ctrl Pts',(-5.15300038646404,23.3334916552407,11.0338465765346));
#6491=CARTESIAN_POINT('Ctrl Pts',(-5.40921927779757,23.3446389614383,10.9105257231928));
#6492=CARTESIAN_POINT('Ctrl Pts',(-5.66083590451648,23.355786267636,10.7783759032675));
#6493=CARTESIAN_POINT('Ctrl Pts',(-5.91240979416356,23.3669316804642,10.6462485289827));
#6494=CARTESIAN_POINT('Ctrl Pts',(-6.15938274378058,23.3780770932925,10.5052953060483));
#6495=CARTESIAN_POINT('Ctrl Pts',(-6.40113673390645,23.3892225061207,10.3558630139566));
#6496=CARTESIAN_POINT('Ctrl Pts',(-6.64286388556777,23.4003666816343,10.2064473111806));
#6497=CARTESIAN_POINT('Ctrl Pts',(-6.87937300783742,23.4115108571478,10.0485545591068));
#6498=CARTESIAN_POINT('Ctrl Pts',(-7.11007321917927,23.4226550326614,9.882576034006));
#6499=CARTESIAN_POINT('Ctrl Pts',(-7.34803865072143,23.4341501609919,9.71137050661351));
#6500=CARTESIAN_POINT('Ctrl Pts',(-7.57982312721504,23.4456452893225,9.53156184412831));
#6501=CARTESIAN_POINT('Ctrl Pts',(-7.80481195646738,23.457140417653,9.34362673559812));
#6502=CARTESIAN_POINT('Ctrl Pts',(-8.02294340543191,23.4682851887384,9.16141965593453));
#6503=CARTESIAN_POINT('Ctrl Pts',(-8.23468710462325,23.4794299598237,8.97157434171908));
#6504=CARTESIAN_POINT('Ctrl Pts',(-8.43951691801119,23.4905747309091,8.77456576934739));
#6505=CARTESIAN_POINT('Ctrl Pts',(-8.65400555820757,23.5022450378623,8.56826718372596));
#6506=CARTESIAN_POINT('Ctrl Pts',(-8.86091234015456,23.5139153448154,8.35411373254376));
#6507=CARTESIAN_POINT('Ctrl Pts',(-9.05967607823019,23.5255856517686,8.13269448630303));
#6508=CARTESIAN_POINT('Ctrl Pts',(-9.2584398163058,23.5372559587218,7.91127524006232));
#6509=CARTESIAN_POINT('Ctrl Pts',(-9.44906029292414,23.5489262656749,7.68259045429057));
#6510=CARTESIAN_POINT('Ctrl Pts',(-9.631023630308,23.5605965726281,7.44727024368318));
#6511=CARTESIAN_POINT('Ctrl Pts',(-9.8048323458045,23.5717438789489,7.22249582415408));
#6512=CARTESIAN_POINT('Ctrl Pts',(-9.97079470968131,23.5828911852698,6.99160050424424));
#6513=CARTESIAN_POINT('Ctrl Pts',(-10.128490951645,23.5940384915906,6.75515516420202));
#6514=CARTESIAN_POINT('Ctrl Pts',(-10.286160408936,23.6051839045438,6.51874998434983));
#6515=CARTESIAN_POINT('Ctrl Pts',(-10.4355663994461,23.6163293174971,6.27679688823947));
#6516=CARTESIAN_POINT('Ctrl Pts',(-10.5763322111555,23.6274747304504,6.0298961192773));
#6517=CARTESIAN_POINT('Ctrl Pts',(-10.7170823956828,23.6386189060904,5.78302276011893));
#6518=CARTESIAN_POINT('Ctrl Pts',(-10.8491941846832,23.6497630817305,5.53120305658148));
#6519=CARTESIAN_POINT('Ctrl Pts',(-10.9723359885886,23.6609072573705,5.27506333644663));
#6520=CARTESIAN_POINT('Ctrl Pts',(-11.0993557765869,23.6724023856074,5.01085725924436));
#6521=CARTESIAN_POINT('Ctrl Pts',(-11.2168313213538,23.6838975138443,4.74205492746937));
#6522=CARTESIAN_POINT('Ctrl Pts',(-11.3244509997133,23.6953926420812,4.46936906118676));
#6523=CARTESIAN_POINT('Ctrl Pts',(-11.4287905658947,23.7065374132952,4.20499431647958));
#6524=CARTESIAN_POINT('Ctrl Pts',(-11.5238660555388,23.7176821845091,3.93696952183191));
#6525=CARTESIAN_POINT('Ctrl Pts',(-11.6094427838768,23.7288269557231,3.66596351562464));
#6526=CARTESIAN_POINT('Ctrl Pts',(-11.6990549123853,23.7404972624715,3.38217812762871));
#6527=CARTESIAN_POINT('Ctrl Pts',(-11.7782507937505,23.7521675692198,3.09512390584126));
#6528=CARTESIAN_POINT('Ctrl Pts',(-11.8468195663286,23.7638378759682,2.80558664326246));
#6529=CARTESIAN_POINT('Ctrl Pts',(-11.9153883389068,23.7755081827165,2.51604938068365));
#6530=CARTESIAN_POINT('Ctrl Pts',(-11.9733299339243,23.7871784894648,2.22402940580713));
#6531=CARTESIAN_POINT('Ctrl Pts',(-12.0204946704578,23.7988487962132,1.93032591224761));
#6532=CARTESIAN_POINT('Ctrl Pts',(-12.0672414471629,23.8104156841837,1.63922513145235));
#6533=CARTESIAN_POINT('Ctrl Pts',(-12.1034122499846,23.8219825721543,1.34640866791079));
#6534=CARTESIAN_POINT('Ctrl Pts',(-12.1289081894145,23.8335494601249,1.05263307128082));
#6535=CARTESIAN_POINT('Ctrl Pts',(-12.1543967460716,23.8451129987108,0.758942542255195));
#6536=CARTESIAN_POINT('Ctrl Pts',(-12.1692165959912,23.8566765372968,0.464293654495028));
#6537=CARTESIAN_POINT('Ctrl Pts',(-12.1733207336769,23.8682400758828,0.169447823923155));
#6538=CARTESIAN_POINT('Ctrl Pts',(-12.1741055719096,23.8704513825889,0.11306416959796));
#6539=CARTESIAN_POINT('Ctrl Pts',(-12.1744986969062,23.872662689295,0.056673323816421));
#6540=CARTESIAN_POINT('Ctrl Pts',(-12.1744999967658,23.8748739960011,0.000280623926556051));
#6541=CARTESIAN_POINT('',(-12.1744999959752,23.6251260039651,0.000313050724133792));
#6542=CARTESIAN_POINT('Ctrl Pts',(1.5908148051505,22.812547089465,12.070351758578));
#6543=CARTESIAN_POINT('Ctrl Pts',(1.19923622262038,22.8280402873171,12.1223796458547));
#6544=CARTESIAN_POINT('Ctrl Pts',(-1.21473510391254,22.9229508930308,12.3241400337495));
#6545=CARTESIAN_POINT('Ctrl Pts',(-5.69424089117864,23.0972789066063,11.3422716237698));
#6546=CARTESIAN_POINT('Ctrl Pts',(-10.4276708680614,23.3355311301914,7.23430593172712));
#6547=CARTESIAN_POINT('Ctrl Pts',(-12.0452929662932,23.5114801626443,2.89768759261325));
#6548=CARTESIAN_POINT('Ctrl Pts',(-12.1750513728812,23.6080117872355,0.436676266174656));
#6549=CARTESIAN_POINT('Ctrl Pts',(-12.1746001704992,23.6251260039651,0.000313053299986626));
#6550=CARTESIAN_POINT('Ctrl Pts',(-12.1744999959752,23.6251260039651,0.000313050724133792));
#6551=CARTESIAN_POINT('Ctrl Pts',(-12.1745072760035,23.6362300684397,-0.28280626030774));
#6552=CARTESIAN_POINT('Ctrl Pts',(-12.1646342579426,23.6473341329143,-0.565958783664843));
#6553=CARTESIAN_POINT('Ctrl Pts',(-12.1449000764791,23.6584381973888,-0.848441148423234));
#6554=CARTESIAN_POINT('Ctrl Pts',(-12.1251680288802,23.6695410611767,-1.13089296825575));
#6555=CARTESIAN_POINT('Ctrl Pts',(-12.0955769658755,23.6806439249646,-1.41267450420121));
#6556=CARTESIAN_POINT('Ctrl Pts',(-12.0561980343215,23.6917467887524,-1.69308570581112));
#6557=CARTESIAN_POINT('Ctrl Pts',(-12.0168162232634,23.7028504644146,-1.97351741191864));
#6558=CARTESIAN_POINT('Ctrl Pts',(-11.9676451482731,23.7139541400767,-2.25257831493435));
#6559=CARTESIAN_POINT('Ctrl Pts',(-11.9088076155506,23.7250578157389,-2.52957534495496));
#6560=CARTESIAN_POINT('Ctrl Pts',(-11.8499700831609,23.7361614913382,-2.80657237340874));
#6561=CARTESIAN_POINT('Ctrl Pts',(-11.7814661517746,23.7472651669375,-3.08150526454602));
#6562=CARTESIAN_POINT('Ctrl Pts',(-11.7034695576592,23.7583688425369,-3.35369207932761));
#6563=CARTESIAN_POINT('Ctrl Pts',(-11.6254556305768,23.7694749856753,-3.62593938143092));
#6564=CARTESIAN_POINT('Ctrl Pts',(-11.5379448995412,23.7805811288137,-3.89543912724969));
#6565=CARTESIAN_POINT('Ctrl Pts',(-11.4411611446377,23.7916872719521,-4.16152398916932));
#6566=CARTESIAN_POINT('Ctrl Pts',(-11.3820531543148,23.7984700404219,-4.3240279285868));
#6567=CARTESIAN_POINT('Ctrl Pts',(-11.3194874657191,23.8052528088917,-4.48525848955029));
#6568=CARTESIAN_POINT('Ctrl Pts',(-11.2535239975975,23.8120355773616,-4.64506704854697));
#6569=CARTESIAN_POINT('Ctrl Pts',(-11.1451147212248,23.8231828842355,-4.90770833670762));
#6570=CARTESIAN_POINT('Ctrl Pts',(-11.027490726027,23.8343301911093,-5.1665920149544));
#6571=CARTESIAN_POINT('Ctrl Pts',(-10.9009381361996,23.8454774979832,-5.42106982068579));
#6572=CARTESIAN_POINT('Ctrl Pts',(-10.7744070412407,23.8566229114949,-5.67550440354045));
#6573=CARTESIAN_POINT('Ctrl Pts',(-10.6389504981074,23.8677683250065,-5.9255343691766));
#6574=CARTESIAN_POINT('Ctrl Pts',(-10.4949015330221,23.8789137385181,-6.17053417964529));
#6575=CARTESIAN_POINT('Ctrl Pts',(-10.3508685595493,23.8900579147204,-6.41550679143171));
#6576=CARTESIAN_POINT('Ctrl Pts',(-10.1982452040525,23.9012020909227,-6.65545013324551));
#6577=CARTESIAN_POINT('Ctrl Pts',(-10.037409578847,23.9123462671249,-6.88976481430757));
#6578=CARTESIAN_POINT('Ctrl Pts',(-9.87150892940053,23.9238413949434,-7.13145851688982));
#6579=CARTESIAN_POINT('Ctrl Pts',(-9.69687054816424,23.9353365227619,-7.36716304913461));
#6580=CARTESIAN_POINT('Ctrl Pts',(-9.51395741258113,23.9468316505804,-7.59625332658098));
#6581=CARTESIAN_POINT('Ctrl Pts',(-9.33661922343069,23.957976422359,-7.8183612403992));
#6582=CARTESIAN_POINT('Ctrl Pts',(-9.1515033916188,23.9691211941376,-8.03425189815682));
#6583=CARTESIAN_POINT('Ctrl Pts',(-8.95907314105923,23.9802659659162,-8.24338878757706));
#6584=CARTESIAN_POINT('Ctrl Pts',(-8.75756880151721,23.9919362717546,-8.4623875710529));
#6585=CARTESIAN_POINT('Ctrl Pts',(-8.54804383413787,24.003606577593,-8.67398007541675));
#6586=CARTESIAN_POINT('Ctrl Pts',(-8.33107475358735,24.0152768834315,-8.87759222425425));
#6587=CARTESIAN_POINT('Ctrl Pts',(-8.11410567303683,24.0269471892699,-9.08120437309175));
#6588=CARTESIAN_POINT('Ctrl Pts',(-7.88969272996757,24.0386174951083,-9.27683594321905));
#6589=CARTESIAN_POINT('Ctrl Pts',(-7.65845451946485,24.0502878009467,-9.46395924670476));
#6590=CARTESIAN_POINT('Ctrl Pts',(-7.43757914943243,24.0614351070725,-9.64269670021316));
#6591=CARTESIAN_POINT('Ctrl Pts',(-7.21041084144513,24.0725824131983,-9.81372509541071));
#6592=CARTESIAN_POINT('Ctrl Pts',(-6.97751105217776,24.0837297193241,-9.97661213873413));
#6593=CARTESIAN_POINT('Ctrl Pts',(-6.74465082092712,24.0948751320805,-10.139471515702));
#6594=CARTESIAN_POINT('Ctrl Pts',(-6.50606127048044,24.1060205448369,-10.2941921487503));
#6595=CARTESIAN_POINT('Ctrl Pts',(-6.26233416579329,24.1171659575934,-10.4403841426424));
#6596=CARTESIAN_POINT('Ctrl Pts',(-6.01863411861028,24.1283101330354,-10.5865599069465));
#6597=CARTESIAN_POINT('Ctrl Pts',(-5.76979788477571,24.1394543084775,-10.7242087855524));
#6598=CARTESIAN_POINT('Ctrl Pts',(-5.51644430519778,24.1505984839195,-10.8529854177388));
#6599=CARTESIAN_POINT('Ctrl Pts',(-5.25511210174971,24.1620936123039,-10.9858174902043));
#6600=CARTESIAN_POINT('Ctrl Pts',(-4.9889736812031,24.1735887406883,-11.1092093074788));
#6601=CARTESIAN_POINT('Ctrl Pts',(-4.71873469727067,24.1850838690726,-11.2228335596129));
#6602=CARTESIAN_POINT('Ctrl Pts',(-4.45673226505212,24.196228640088,-11.3329946843513));
#6603=CARTESIAN_POINT('Ctrl Pts',(-4.19087578555295,24.2073734111034,-11.4339747257494));
#6604=CARTESIAN_POINT('Ctrl Pts',(-3.92182874309239,24.2185181821189,-11.5255242639914));
#6605=CARTESIAN_POINT('Ctrl Pts',(-3.64009468169887,24.2301884891877,-11.6213908566577));
#6606=CARTESIAN_POINT('Ctrl Pts',(-3.35486221345111,24.2418587962565,-11.7069160450841));
#6607=CARTESIAN_POINT('Ctrl Pts',(-3.06691227567061,24.2535291033253,-11.7818716400808));
#6608=CARTESIAN_POINT('Ctrl Pts',(-2.77896233789011,24.2651994103942,-11.8568272350776));
#6609=CARTESIAN_POINT('Ctrl Pts',(-2.48829525746922,24.276869717463,-11.9212131606227));
#6610=CARTESIAN_POINT('Ctrl Pts',(-2.19570672218016,24.2885400245318,-11.9748620969167));
#6611=CARTESIAN_POINT('Ctrl Pts',(-1.91623044331381,24.2996873307296,-12.0261067742441));
#6612=CARTESIAN_POINT('Ctrl Pts',(-1.63491767399143,24.3108346369273,-12.0675709631649));
#6613=CARTESIAN_POINT('Ctrl Pts',(-1.35246828020352,24.3219819431251,-12.0991437631364));
#6614=CARTESIAN_POINT('Ctrl Pts',(-1.07006686043198,24.3331273559534,-12.1307112004694));
#6615=CARTESIAN_POINT('Ctrl Pts',(-0.786529466626027,24.3442727687818,-12.1523905734547));
#6616=CARTESIAN_POINT('Ctrl Pts',(-0.502562287985054,24.3554181816101,-12.1641227138128));
#6617=CARTESIAN_POINT('Ctrl Pts',(-0.218626634131015,24.3665623571237,-12.1758535517201));
#6618=CARTESIAN_POINT('Ctrl Pts',(0.0657384428316171,24.3777065326373,-12.1776393510993));
#6619=CARTESIAN_POINT('Ctrl Pts',(0.349824290943899,24.388850708151,-12.1694730048374));
#6620=CARTESIAN_POINT('Ctrl Pts',(0.642856581841975,24.4003458364815,-12.1610494836753));
#6621=CARTESIAN_POINT('Ctrl Pts',(0.935591475061742,24.411840964812,-12.1420368316069));
#6622=CARTESIAN_POINT('Ctrl Pts',(1.22725272951155,24.4233360931424,-12.1124853348892));
#6623=CARTESIAN_POINT('Ctrl Pts',(1.51002451090461,24.434480864228,-12.0838345311154));
#6624=CARTESIAN_POINT('Ctrl Pts',(1.79178685310391,24.4456256353135,-12.0452778196722));
#6625=CARTESIAN_POINT('Ctrl Pts',(2.07183781618613,24.456770406399,-11.9969136995071));
#6626=CARTESIAN_POINT('Ctrl Pts',(2.36509468764385,24.468440713352,-11.9462689510859));
#6627=CARTESIAN_POINT('Ctrl Pts',(2.65647458170317,24.480111020305,-11.8848696481258));
#6628=CARTESIAN_POINT('Ctrl Pts',(2.94518258695251,24.4917813272579,-11.8128891376967));
#6629=CARTESIAN_POINT('Ctrl Pts',(3.23389059220187,24.5034516342109,-11.7409086272675));
#6630=CARTESIAN_POINT('Ctrl Pts',(3.51992638522904,24.5151219411639,-11.6583469990491));
#6631=CARTESIAN_POINT('Ctrl Pts',(3.8025112313794,24.5267922481169,-11.5654381060656));
#6632=CARTESIAN_POINT('Ctrl Pts',(4.07243213870612,24.5379395544373,-11.4766928918955));
#6633=CARTESIAN_POINT('Ctrl Pts',(4.33928522123258,24.5490868607576,-11.3784809408964));
#6634=CARTESIAN_POINT('Ctrl Pts',(4.60240288097398,24.560234167078,-11.2710397910398));
#6635=CARTESIAN_POINT('Ctrl Pts',(4.86547585023803,24.5713795800308,-11.1636168900391));
#6636=CARTESIAN_POINT('Ctrl Pts',(5.12481441655924,24.5825249929836,-11.0469680206508));
#6637=CARTESIAN_POINT('Ctrl Pts',(5.37977018586658,24.5936704059364,-10.9213791710233));
#6638=CARTESIAN_POINT('Ctrl Pts',(5.63469765113895,24.604814581576,-10.7958042637012));
#6639=CARTESIAN_POINT('Ctrl Pts',(5.88524305174738,24.6159587572155,-10.6612914757993));
#6640=CARTESIAN_POINT('Ctrl Pts',(6.13078074465165,24.627102932855,-10.5181736870527));
#6641=CARTESIAN_POINT('Ctrl Pts',(6.38405091539444,24.6385980610923,-10.3705488300972));
#6642=CARTESIAN_POINT('Ctrl Pts',(6.63199260058101,24.6500931893295,-10.2137683531929));
#6643=CARTESIAN_POINT('Ctrl Pts',(6.87394827478413,24.6615883175668,-10.0482478754056));
#6644=CARTESIAN_POINT('Ctrl Pts',(7.10852944492335,24.6727330887802,-9.88777225321056));
#6645=CARTESIAN_POINT('Ctrl Pts',(7.33748386258186,24.6838778599937,-9.71908166691572));
#6646=CARTESIAN_POINT('Ctrl Pts',(7.5602423153278,24.6950226312072,-9.54259851316857));
#6647=CARTESIAN_POINT('Ctrl Pts',(7.79350501984766,24.7066929379563,-9.35779323535402));
#6648=CARTESIAN_POINT('Ctrl Pts',(8.01997310417797,24.7183632447054,-9.16444298150568));
#6649=CARTESIAN_POINT('Ctrl Pts',(8.23903153901835,24.7300335514546,-8.96308036051563));
#6650=CARTESIAN_POINT('Ctrl Pts',(8.45808997385872,24.7417038582037,-8.76171773952559));
#6651=CARTESIAN_POINT('Ctrl Pts',(8.66973851814809,24.7533741649529,-8.55234298490495));
#6652=CARTESIAN_POINT('Ctrl Pts',(8.87340530149632,24.765044471702,-8.33553409238886));
#6653=CARTESIAN_POINT('Ctrl Pts',(9.0679448319984,24.7761917778973,-8.12844141156305));
#6654=CARTESIAN_POINT('Ctrl Pts',(9.25526037748929,24.7873390840926,-7.91450441257048));
#6655=CARTESIAN_POINT('Ctrl Pts',(9.43487941609193,24.7984863902879,-7.69425114314608));
#6656=CARTESIAN_POINT('Ctrl Pts',(9.61446794641304,24.8096318031139,-7.47403528372458));
#6657=CARTESIAN_POINT('Ctrl Pts',(9.78636241125291,24.82077721594,-7.24750550239521));
#6658=CARTESIAN_POINT('Ctrl Pts',(9.95013033648356,24.8319226287661,-7.01522319937076));
#6659=CARTESIAN_POINT('Ctrl Pts',(10.1138800809248,24.8430668042778,-6.78296668329837));
#6660=CARTESIAN_POINT('Ctrl Pts',(10.2695049335853,24.8542109797896,-6.54495913870715));
#6661=CARTESIAN_POINT('Ctrl Pts',(10.4166148368308,24.8653551553013,-6.30179225229755));
#6662=CARTESIAN_POINT('Ctrl Pts',(10.5683575310261,24.8768502836335,-6.05096754458694));
#6663=CARTESIAN_POINT('Ctrl Pts',(10.711040117134,24.8883454119656,-5.79465352177918));
#6664=CARTESIAN_POINT('Ctrl Pts',(10.8442841370161,24.8998405402978,-5.53352977814893));
#6665=CARTESIAN_POINT('Ctrl Pts',(10.973467044506,24.9109853113819,-5.28036476221306));
#6666=CARTESIAN_POINT('Ctrl Pts',(11.0937780907119,24.9221300824661,-5.02267912115139));
#6667=CARTESIAN_POINT('Ctrl Pts',(11.2049196053669,24.9332748535502,-4.761116138813));
#6668=CARTESIAN_POINT('Ctrl Pts',(11.3213020399456,24.9449451605064,-4.48721905566886));
#6669=CARTESIAN_POINT('Ctrl Pts',(11.4276292249522,24.9566154674625,-4.20907045001883));
#6670=CARTESIAN_POINT('Ctrl Pts',(11.5236160012059,24.9682857744187,-3.92743230454083));
#6671=CARTESIAN_POINT('Ctrl Pts',(11.6196027774596,24.9799560813748,-3.64579415906282));
#6672=CARTESIAN_POINT('Ctrl Pts',(11.7052490450383,24.991626388331,-3.36066679415267));
#6673=CARTESIAN_POINT('Ctrl Pts',(11.7803292606082,25.0032966952871,-3.07283139167434));
#6674=CARTESIAN_POINT('Ctrl Pts',(11.8520447828511,25.0144440015614,-2.79789523103511));
#6675=CARTESIAN_POINT('Ctrl Pts',(11.9141418832278,25.0255913078357,-2.52040630438659));
#6676=CARTESIAN_POINT('Ctrl Pts',(11.9664583505487,25.03673861411,-2.24105439349054));
#6677=CARTESIAN_POINT('Ctrl Pts',(12.0187659319259,25.047884027016,-1.96174993047246));
#6678=CARTESIAN_POINT('Ctrl Pts',(12.0612961478269,25.0590294399221,-1.680583377044));
#6679=CARTESIAN_POINT('Ctrl Pts',(12.0939379121453,25.0701748528282,-1.39825463602789));
#6680=CARTESIAN_POINT('Ctrl Pts',(12.1265760527213,25.0813190284204,-1.11595723788416));
#6681=CARTESIAN_POINT('Ctrl Pts',(12.1493279031616,25.0924632040126,-0.832498174701055));
#6682=CARTESIAN_POINT('Ctrl Pts',(12.1621341151456,25.1036073796049,-0.548583644680526));
#6683=CARTESIAN_POINT('Ctrl Pts',(12.1753436207048,25.1151025078772,-0.255728070579462));
#6684=CARTESIAN_POINT('Ctrl Pts',(12.1779708973995,25.1265976361494,0.0376118263910138));
#6685=CARTESIAN_POINT('Ctrl Pts',(12.1700088495403,25.1380927644217,0.330658210410661));
#6686=CARTESIAN_POINT('Ctrl Pts',(12.1622894749236,25.1492375355872,0.61477290782209));
#6687=CARTESIAN_POINT('Ctrl Pts',(12.1446167235003,25.1603823067528,0.898611440186133));
#6688=CARTESIAN_POINT('Ctrl Pts',(12.1170370604352,25.1715270779183,1.18146651498856));
#6689=CARTESIAN_POINT('Ctrl Pts',(12.0881568685195,25.1831973847439,1.47765972174982));
#6690=CARTESIAN_POINT('Ctrl Pts',(12.0484129862963,25.1948676915696,1.77277417226269));
#6691=CARTESIAN_POINT('Ctrl Pts',(11.9979196669199,25.2065379983952,2.06600433594332));
#6692=CARTESIAN_POINT('Ctrl Pts',(11.9474263475436,25.2182083052209,2.35923449962396));
#6693=CARTESIAN_POINT('Ctrl Pts',(11.8861836565992,25.2298786120466,2.65058004732725));
#6694=CARTESIAN_POINT('Ctrl Pts',(11.814367381413,25.2415489188722,2.93924711907746));
#6695=CARTESIAN_POINT('Ctrl Pts',(11.7457695266862,25.2526962251084,3.21497768016523));
#6696=CARTESIAN_POINT('Ctrl Pts',(11.6675044717985,25.2638435313446,3.48834690833357));
#6697=CARTESIAN_POINT('Ctrl Pts',(11.5797598749238,25.2749908375808,3.75867150587886));
#6698=CARTESIAN_POINT('Ctrl Pts',(11.4920301814584,25.2861362504483,4.02895018882332));
#6699=CARTESIAN_POINT('Ctrl Pts',(11.3948242428908,25.2972816633159,4.29618501997487));
#6700=CARTESIAN_POINT('Ctrl Pts',(11.2883794518641,25.3084270761834,4.55970828022289));
#6701=CARTESIAN_POINT('Ctrl Pts',(11.1819464778628,25.319571251737,4.82320228529501));
#6702=CARTESIAN_POINT('Ctrl Pts',(11.0662767993538,25.3307154272905,5.08298529497744));
#6703=CARTESIAN_POINT('Ctrl Pts',(10.9416562506894,25.3418596028441,5.33840882115168));
#6704=CARTESIAN_POINT('Ctrl Pts',(10.8131111475577,25.3533547311452,5.60187615351543));
#6705=CARTESIAN_POINT('Ctrl Pts',(10.6750423980179,25.3648498594463,5.86070470407446));
#6706=CARTESIAN_POINT('Ctrl Pts',(10.5278159992574,25.3763449877474,6.11420808737982));
#6707=CARTESIAN_POINT('Ctrl Pts',(10.3850768775203,25.3874897588738,6.35998500371434));
#6708=CARTESIAN_POINT('Ctrl Pts',(10.233730207958,25.3986345300003,6.60075631358498));
#6709=CARTESIAN_POINT('Ctrl Pts',(10.0741552596408,25.4097793011267,6.83592320426813));
#6710=CARTESIAN_POINT('Ctrl Pts',(9.90705549622338,25.4214496080151,7.08217947576419));
#6711=CARTESIAN_POINT('Ctrl Pts',(9.7309329452156,25.4331199149036,7.322289790146));
#6712=CARTESIAN_POINT('Ctrl Pts',(9.54627340902399,25.444790221792,7.55560151478104));
#6713=CARTESIAN_POINT('Ctrl Pts',(9.36161387283237,25.4564605286804,7.7889132394161));
#6714=CARTESIAN_POINT('Ctrl Pts',(9.16841756655482,25.4681308355689,8.01542611667906));
#6715=CARTESIAN_POINT('Ctrl Pts',(8.96721873867355,25.4798011424573,8.2345272082119));
#6716=CARTESIAN_POINT('Ctrl Pts',(8.77503656446375,25.4909484487072,8.44380936251634));
#6717=CARTESIAN_POINT('Ctrl Pts',(8.57549596571777,25.5020957549571,8.64639194661431));
#6718=CARTESIAN_POINT('Ctrl Pts',(8.36908870550682,25.513243061207,8.84176478364802));
#6719=CARTESIAN_POINT('Ctrl Pts',(8.16271650354248,25.5243884740884,9.03710443663048));
#6720=CARTESIAN_POINT('Ctrl Pts',(7.94948016228641,25.5355338869698,9.22523660411167));
#6721=CARTESIAN_POINT('Ctrl Pts',(7.7299076598487,25.5466792998511,9.40568858830721));
#6722=CARTESIAN_POINT('Ctrl Pts',(7.51035953336922,25.5578234754186,9.58612053952967));
#6723=CARTESIAN_POINT('Ctrl Pts',(7.28447685633949,25.568967650986,9.75887384069105));
#6724=CARTESIAN_POINT('Ctrl Pts',(7.0528209389533,25.5801118265534,9.92351586148084));
#6725=CARTESIAN_POINT('Ctrl Pts',(6.81386970621717,25.5916069548442,10.0933427939062));
#6726=CARTESIAN_POINT('Ctrl Pts',(6.56877595494336,25.6031020831349,10.2545391062416));
#6727=CARTESIAN_POINT('Ctrl Pts',(6.31818951893479,25.6145972114257,10.4066772532265));
#6728=CARTESIAN_POINT('Ctrl Pts',(6.075240644456,25.6257419825662,10.5541784195467));
#6729=CARTESIAN_POINT('Ctrl Pts',(5.82712918612156,25.6368867537066,10.6931652624026));
#6730=CARTESIAN_POINT('Ctrl Pts',(5.57447472401569,25.6480315248471,10.8232934821758));
#6731=CARTESIAN_POINT('Ctrl Pts',(5.30990624911035,25.659701831713,10.9595579453506));
#6732=CARTESIAN_POINT('Ctrl Pts',(5.04035628965848,25.6713721385789,11.0861080739867));
#6733=CARTESIAN_POINT('Ctrl Pts',(4.7665637239795,25.6830424454448,11.2026032918801));
#6734=CARTESIAN_POINT('Ctrl Pts',(4.49277115830052,25.6947127523106,11.3190985097735));
#6735=CARTESIAN_POINT('Ctrl Pts',(4.21473629854894,25.7063830591765,11.4255386936461));
#6736=CARTESIAN_POINT('Ctrl Pts',(3.93322156640711,25.7180533660424,11.5216413049335));
#6737=CARTESIAN_POINT('Ctrl Pts',(3.66432536802045,25.7292005664975,11.6134362409698));
#6738=CARTESIAN_POINT('Ctrl Pts',(3.3921740921302,25.7403477669525,11.6958273819203));
#6739=CARTESIAN_POINT('Ctrl Pts',(3.11744366041665,25.7514949674076,11.7686020951568));
#6740=CARTESIAN_POINT('Ctrl Pts',(2.84275170720437,25.7626406065956,11.8413666156312));
#6741=CARTESIAN_POINT('Ctrl Pts',(2.56548157682794,25.7737862457837,11.9045173279686));
#6742=CARTESIAN_POINT('Ctrl Pts',(2.28632311610678,25.7849318849717,11.9578918233423));
#6743=CARTESIAN_POINT('Ctrl Pts',(2.05563452691691,25.7941423232771,12.0019989838584));
#6744=CARTESIAN_POINT('Ctrl Pts',(1.82365674195867,25.8033527615825,12.0394309579504));
#6745=CARTESIAN_POINT('Ctrl Pts',(1.59078448392773,25.8125631998879,12.0701224093086));
#6746=CARTESIAN_POINT('Origin',(0.,13.3748739960349,0.));
#6747=CARTESIAN_POINT('',(1.59078448392773,29.0623127728906,12.0701224093087));
#6748=CARTESIAN_POINT('',(1.59078448392775,28.8125580693322,12.0701224093086));
#6749=CARTESIAN_POINT('',(1.59078448392774,13.3748739960349,12.0701224093086));
#6750=CARTESIAN_POINT('',(-12.1744999986836,26.8748739959973,-0.000179033899940194));
#6751=CARTESIAN_POINT('Ctrl Pts',(-12.1744999986836,26.8748739960349,-0.000179034858391824));
#6752=CARTESIAN_POINT('Ctrl Pts',(-12.1744973429416,26.8819585649631,-0.180771412597766));
#6753=CARTESIAN_POINT('Ctrl Pts',(-12.170475924864,26.8890431338913,-0.361351713761423));
#6754=CARTESIAN_POINT('Ctrl Pts',(-12.1624403133837,26.8961277028195,-0.541752594251753));
#6755=CARTESIAN_POINT('Ctrl Pts',(-12.1497965769811,26.9072750090666,-0.825606683675804));
#6756=CARTESIAN_POINT('Ctrl Pts',(-12.127209485585,26.9184223153137,-1.109060343361));
#6757=CARTESIAN_POINT('Ctrl Pts',(-12.094727685764,26.9295696215608,-1.39140664696373));
#6758=CARTESIAN_POINT('Ctrl Pts',(-12.0622514029725,26.9407150344394,-1.67370499408291));
#6759=CARTESIAN_POINT('Ctrl Pts',(-12.0198837975782,26.9518604473179,-1.95489609573094));
#6760=CARTESIAN_POINT('Ctrl Pts',(-11.9677253505645,26.9630058601965,-2.23427844805787));
#6761=CARTESIAN_POINT('Ctrl Pts',(-11.9155726939485,26.9741500357611,-2.51362978460458));
#6762=CARTESIAN_POINT('Ctrl Pts',(-11.8536314150918,26.9852942113258,-2.79117251064493));
#6763=CARTESIAN_POINT('Ctrl Pts',(-11.7820532854202,26.9964383868904,-3.0662143808806));
#6764=CARTESIAN_POINT('Ctrl Pts',(-11.7082210150325,27.0079335151833,-3.3499178783647));
#6765=CARTESIAN_POINT('Ctrl Pts',(-11.6241351555881,27.0194286434761,-3.63096016396926));
#6766=CARTESIAN_POINT('Ctrl Pts',(-11.530018550358,27.030923771769,-3.90859597277591));
#6767=CARTESIAN_POINT('Ctrl Pts',(-11.4387705017224,27.0420685429066,-4.17776978884194));
#6768=CARTESIAN_POINT('Ctrl Pts',(-11.3380941917879,27.0532133140442,-4.44374143924996));
#6769=CARTESIAN_POINT('Ctrl Pts',(-11.2282428127532,27.0643580851818,-4.70584887006112));
#6770=CARTESIAN_POINT('Ctrl Pts',(-11.1132113520216,27.0760283920523,-4.98031607201867));
#6771=CARTESIAN_POINT('Ctrl Pts',(-10.9881188167639,27.0876986989227,-5.25054555485061));
#6772=CARTESIAN_POINT('Ctrl Pts',(-10.8533121666699,27.0993690057932,-5.51580141618739));
#6773=CARTESIAN_POINT('Ctrl Pts',(-10.7185055165759,27.1110393126637,-5.78105727752418));
#6774=CARTESIAN_POINT('Ctrl Pts',(-10.5739849114736,27.1227096195341,-6.04133922225082));
#6775=CARTESIAN_POINT('Ctrl Pts',(-10.4201526576011,27.1343799264046,-6.29594066381572));
#6776=CARTESIAN_POINT('Ctrl Pts',(-10.2732143410997,27.1455272326517,-6.53913223294777));
#6777=CARTESIAN_POINT('Ctrl Pts',(-10.1177367424751,27.1566745388988,-6.77721387905434));
#6778=CARTESIAN_POINT('Ctrl Pts',(-9.95410087098509,27.167821845146,-7.00958815482435));
#6779=CARTESIAN_POINT('Ctrl Pts',(-9.79049279302736,27.1789672580245,-7.24192296185269));
#6780=CARTESIAN_POINT('Ctrl Pts',(-9.61872936224129,27.190112670903,-7.46855211592874));
#6781=CARTESIAN_POINT('Ctrl Pts',(-9.43923450693786,27.2012580837816,-7.68890773602035));
#6782=CARTESIAN_POINT('Ctrl Pts',(-9.2597595783524,27.2124022593461,-7.9092388932142));
#6783=CARTESIAN_POINT('Ctrl Pts',(-9.07255510757798,27.2235464349107,-8.12329770037941));
#6784=CARTESIAN_POINT('Ctrl Pts',(-8.87808562861877,27.2346906104752,-8.33054895075426));
#6785=CARTESIAN_POINT('Ctrl Pts',(-8.67749191069513,27.2461857387681,-8.54432696404207));
#6786=CARTESIAN_POINT('Ctrl Pts',(-8.46916838599521,27.257680867061,-8.75086148201259));
#6787=CARTESIAN_POINT('Ctrl Pts',(-8.25366736632376,27.2691759953538,-8.94960475418229));
#6788=CARTESIAN_POINT('Ctrl Pts',(-8.04473454861487,27.2803207664914,-9.14229057960626));
#6789=CARTESIAN_POINT('Ctrl Pts',(-7.82905548443714,27.291465537629,-9.32765287209847));
#6790=CARTESIAN_POINT('Ctrl Pts',(-7.60716931389788,27.3026103087666,-9.50523146902223));
#6791=CARTESIAN_POINT('Ctrl Pts',(-7.37482002035491,27.3142806156371,-9.69118384921479));
#6792=CARTESIAN_POINT('Ctrl Pts',(-7.13566438620726,27.3259509225076,-9.86860058581242));
#6793=CARTESIAN_POINT('Ctrl Pts',(-6.89035922507428,27.3376212293782,-10.0370015442578));
#6794=CARTESIAN_POINT('Ctrl Pts',(-6.64505406394129,27.3492915362487,-10.2054025027032));
#6795=CARTESIAN_POINT('Ctrl Pts',(-6.39359965738751,27.3609618431192,-10.3647875003511));
#6796=CARTESIAN_POINT('Ctrl Pts',(-6.13668738798872,27.3726321499897,-10.5147286295035));
#6797=CARTESIAN_POINT('Ctrl Pts',(-5.89128854994562,27.3837794562368,-10.6579502006452));
#6798=CARTESIAN_POINT('Ctrl Pts',(-5.64083698966155,27.3949267624839,-10.7925985197516));
#6799=CARTESIAN_POINT('Ctrl Pts',(-5.38595316180751,27.4060740687311,-10.9183313188791));
#6800=CARTESIAN_POINT('Ctrl Pts',(-5.13111262593913,27.4172194816096,-11.0440427623067));
#6801=CARTESIAN_POINT('Ctrl Pts',(-4.87184156463934,27.4283648944882,-11.1608415910916));
#6802=CARTESIAN_POINT('Ctrl Pts',(-4.60878396953977,27.4395103073668,-11.2684320369834));
#6803=CARTESIAN_POINT('Ctrl Pts',(-4.3457555779199,27.4506544829314,-11.3760105386643));
#6804=CARTESIAN_POINT('Ctrl Pts',(-4.07894173873217,27.461798658496,-11.4743825978158));
#6805=CARTESIAN_POINT('Ctrl Pts',(-3.80900646198326,27.4729428340606,-11.5633005678556));
#6806=CARTESIAN_POINT('Ctrl Pts',(-3.53057037498807,27.4844379623534,-11.6550187454114));
#6807=CARTESIAN_POINT('Ctrl Pts',(-3.24881334259174,27.4959330906463,-11.7366776258322));
#6808=CARTESIAN_POINT('Ctrl Pts',(-2.96448245205888,27.5074282189391,-11.8080605537673));
#6809=CARTESIAN_POINT('Ctrl Pts',(-2.68881761199677,27.5185729900768,-11.877267819202));
#6810=CARTESIAN_POINT('Ctrl Pts',(-2.41073375712401,27.5297177612144,-11.9368161849391));
#6811=CARTESIAN_POINT('Ctrl Pts',(-2.13092449458315,27.540862532352,-11.9865596001682));
#6812=CARTESIAN_POINT('Ctrl Pts',(-1.83792072458815,27.5525328392224,-12.0386486842186));
#6813=CARTESIAN_POINT('Ctrl Pts',(-1.5430252199813,27.5642031460929,-12.0799857998834));
#6814=CARTESIAN_POINT('Ctrl Pts',(-1.24704447022982,27.5758734529634,-12.1104636715226));
#6815=CARTESIAN_POINT('Ctrl Pts',(-0.951063720478334,27.5875437598338,-12.1409415431618));
#6816=CARTESIAN_POINT('Ctrl Pts',(-0.653998060217559,27.5992140667043,-12.1605601451418));
#6817=CARTESIAN_POINT('Ctrl Pts',(-0.356659339898103,27.6108843735748,-12.1692746030839));
#6818=CARTESIAN_POINT('Ctrl Pts',(-0.0726457478549768,27.6220316798219,
-12.177598525714));
#6819=CARTESIAN_POINT('Ctrl Pts',(0.211701791907702,27.633178986069,-12.175976638602));
#6820=CARTESIAN_POINT('Ctrl Pts',(0.495674690478524,27.6443262923161,-12.1644053225474));
#6821=CARTESIAN_POINT('Ctrl Pts',(0.779599356289084,27.6554717051947,-12.1528359718793));
#6822=CARTESIAN_POINT('Ctrl Pts',(1.06314924152558,27.6666171180733,-12.1313205770283));
#6823=CARTESIAN_POINT('Ctrl Pts',(1.34561734240108,27.6777625309519,-12.0999076119543));
#6824=CARTESIAN_POINT('Ctrl Pts',(1.6280540849292,27.6889067065165,-12.0684981342074));
#6825=CARTESIAN_POINT('Ctrl Pts',(1.9094090178618,27.7000508820811,-12.02719330981));
#6826=CARTESIAN_POINT('Ctrl Pts',(2.18898058826488,27.7111950576458,-11.9760934462871));
#6827=CARTESIAN_POINT('Ctrl Pts',(2.47735643537739,27.7226901859386,-11.923384344251));
#6828=CARTESIAN_POINT('Ctrl Pts',(2.76383448278513,27.7341853142314,-11.8602533185206));
#6829=CARTESIAN_POINT('Ctrl Pts',(3.04765506100921,27.7456804425243,-11.7868676449303));
#6830=CARTESIAN_POINT('Ctrl Pts',(3.32282514244449,27.7568252136619,-11.7157186750269));
#6831=CARTESIAN_POINT('Ctrl Pts',(3.59549707841157,27.7679699847995,-11.6349309684199));
#6832=CARTESIAN_POINT('Ctrl Pts',(3.86499194570396,27.7791147559371,-11.5447082037461));
#6833=CARTESIAN_POINT('Ctrl Pts',(4.14719494139433,27.7907850628076,-11.4502309518185));
#6834=CARTESIAN_POINT('Ctrl Pts',(4.42591372566347,27.8024553696781,-11.3454075047072));
#6835=CARTESIAN_POINT('Ctrl Pts',(4.70038881294249,27.8141256765485,-11.2305296071541));
#6836=CARTESIAN_POINT('Ctrl Pts',(4.97486390022151,27.825795983419,-11.115651709601));
#6837=CARTESIAN_POINT('Ctrl Pts',(5.24509498441225,27.8374662902895,-10.9907194992353));
#6838=CARTESIAN_POINT('Ctrl Pts',(5.5103477343262,27.8491365971599,-10.8560820785773));
#6839=CARTESIAN_POINT('Ctrl Pts',(5.76371327723781,27.860283903407,-10.7274783857133));
#6840=CARTESIAN_POINT('Ctrl Pts',(6.01261255303692,27.8714312096541,-10.5899818243253));
#6841=CARTESIAN_POINT('Ctrl Pts',(6.2564216431686,27.8825785159013,-10.4439283065756));
#6842=CARTESIAN_POINT('Ctrl Pts',(6.50018932235742,27.8937239287798,-10.2978995959973));
#6843=CARTESIAN_POINT('Ctrl Pts',(6.73886831324427,27.9048693416584,-10.1433169677941));
#6844=CARTESIAN_POINT('Ctrl Pts',(6.97186101791719,27.916014754537,-9.98056131672196));
#6845=CARTESIAN_POINT('Ctrl Pts',(7.20482785678025,27.9271589301016,-9.81782373405559));
#6846=CARTESIAN_POINT('Ctrl Pts',(7.43210945134621,27.9383031056662,-9.64691509303569));
#6847=CARTESIAN_POINT('Ctrl Pts',(7.6531377944767,27.9494472812308,-9.46825919315438));
#6848=CARTESIAN_POINT('Ctrl Pts',(7.88112676915815,27.9609424095236,-9.28397705604092));
#6849=CARTESIAN_POINT('Ctrl Pts',(8.10246201817212,27.9724375378165,-9.09145197819303));
#6850=CARTESIAN_POINT('Ctrl Pts',(8.31655655151377,27.9839326661093,-8.89119437283166));
#6851=CARTESIAN_POINT('Ctrl Pts',(8.52412575084056,27.9950774372469,-8.69704036919988));
#6852=CARTESIAN_POINT('Ctrl Pts',(8.7248888707482,28.0062222083845,-8.49561840443982));
#6853=CARTESIAN_POINT('Ctrl Pts',(8.91834724194499,28.0173669795222,-8.28743221523363));
#6854=CARTESIAN_POINT('Ctrl Pts',(9.12092821293592,28.0290372863926,-8.06942893062317));
#6855=CARTESIAN_POINT('Ctrl Pts',(9.31549872612246,28.0407075932631,-7.84400836552933));
#6856=CARTESIAN_POINT('Ctrl Pts',(9.50153151667196,28.0523779001336,-7.61179013686593));
#6857=CARTESIAN_POINT('Ctrl Pts',(9.68756430722147,28.0640482070041,-7.37957190820253));
#6858=CARTESIAN_POINT('Ctrl Pts',(9.86505917222155,28.0757185138745,-7.14055628329797));
#6859=CARTESIAN_POINT('Ctrl Pts',(10.0335383821488,28.087388820745,-6.89540120543738));
#6860=CARTESIAN_POINT('Ctrl Pts',(10.194467256614,28.0985361269921,-6.66123266460331));
#6861=CARTESIAN_POINT('Ctrl Pts',(10.3472188441184,28.1096834332392,-6.42139291309911));
#6862=CARTESIAN_POINT('Ctrl Pts',(10.4914060523786,28.1208307394863,-6.1764754750677));
#6863=CARTESIAN_POINT('Ctrl Pts',(10.6355687704599,28.1319761523649,-5.93159963623197));
#6864=CARTESIAN_POINT('Ctrl Pts',(10.7711698782457,28.1431215652434,-5.68164806252201));
#6865=CARTESIAN_POINT('Ctrl Pts',(10.8978669207609,28.154266978122,-5.42724118013789));
#6866=CARTESIAN_POINT('Ctrl Pts',(11.0245498979363,28.1654111536866,-5.1728625408699));
#6867=CARTESIAN_POINT('Ctrl Pts',(11.1423306648156,28.1765553292512,-4.91402981929681));
#6868=CARTESIAN_POINT('Ctrl Pts',(11.250913280774,28.1876995048158,-4.65138695428623));
#6869=CARTESIAN_POINT('Ctrl Pts',(11.3629153838978,28.1991946331086,-4.38047293188917));
#6870=CARTESIAN_POINT('Ctrl Pts',(11.4651304890387,28.2106897614015,-4.10550516952863));
#6871=CARTESIAN_POINT('Ctrl Pts',(11.5572874357625,28.2221848896944,-3.82721274260596));
#6872=CARTESIAN_POINT('Ctrl Pts',(11.6466355538357,28.2333296608319,-3.55740232132468));
#6873=CARTESIAN_POINT('Ctrl Pts',(11.7265294669145,28.2444744319695,-3.28446716262288));
#6874=CARTESIAN_POINT('Ctrl Pts',(11.7967723708194,28.2556192031071,-3.00908821423886));
#6875=CARTESIAN_POINT('Ctrl Pts',(11.8703276043836,28.2672895099776,-2.72072367147365));
#6876=CARTESIAN_POINT('Ctrl Pts',(11.9332996556248,28.2789598168481,-2.42967962578353));
#6877=CARTESIAN_POINT('Ctrl Pts',(11.9855220652797,28.2906301237186,-2.13675245938659));
#6878=CARTESIAN_POINT('Ctrl Pts',(12.0377444749345,28.3023004305891,-1.84382529298966));
#6879=CARTESIAN_POINT('Ctrl Pts',(12.0792171927608,28.3139707374596,-1.54901533771966));
#6880=CARTESIAN_POINT('Ctrl Pts',(12.1098355954862,28.3256410443301,-1.25312892405157));
#6881=CARTESIAN_POINT('Ctrl Pts',(12.1390818454577,28.3367883505772,-0.970502554057997));
#6882=CARTESIAN_POINT('Ctrl Pts',(12.1584339953508,28.3479356568243,-0.686809677550053));
#6883=CARTESIAN_POINT('Ctrl Pts',(12.1678361799058,28.3590829630714,-0.40275668706502));
#6884=CARTESIAN_POINT('Ctrl Pts',(12.177236767501,28.37022837595,-0.118751942944197));
#6885=CARTESIAN_POINT('Ctrl Pts',(12.1766907550221,28.3813737888286,0.165612526537045));
#6886=CARTESIAN_POINT('Ctrl Pts',(12.1661943454187,28.3925192017072,0.449628067964166));
#6887=CARTESIAN_POINT('Ctrl Pts',(12.1556991010799,28.4036633772718,0.733612079254089));
#6888=CARTESIAN_POINT('Ctrl Pts',(12.1352556752733,28.4148075528364,1.0172469733435));
#6889=CARTESIAN_POINT('Ctrl Pts',(12.104912365353,28.425951728401,1.29982571028703));
#6890=CARTESIAN_POINT('Ctrl Pts',(12.07361348296,28.4374468566938,1.59130342572396));
#6891=CARTESIAN_POINT('Ctrl Pts',(12.0317810995415,28.4489419849867,1.88165708895882));
#6892=CARTESIAN_POINT('Ctrl Pts',(11.9795260125188,28.4604371132795,2.1701167630765));
#6893=CARTESIAN_POINT('Ctrl Pts',(11.9288635952924,28.4715818844171,2.44978454655556));
#6894=CARTESIAN_POINT('Ctrl Pts',(11.8684044580646,28.4827266555547,2.727671809539));
#6895=CARTESIAN_POINT('Ctrl Pts',(11.7983016566862,28.4938714266923,3.00308645693653));
#6896=CARTESIAN_POINT('Ctrl Pts',(11.7248931322342,28.5055417335628,3.29148838211453));
#6897=CARTESIAN_POINT('Ctrl Pts',(11.6409096368336,28.5172120404333,3.57717857842725));
#6898=CARTESIAN_POINT('Ctrl Pts',(11.5465861114499,28.5288823473038,3.85937811322915));
#6899=CARTESIAN_POINT('Ctrl Pts',(11.4522625860663,28.5405526541742,4.14157764803105));
#6900=CARTESIAN_POINT('Ctrl Pts',(11.3475991453805,28.5522229610447,4.42028620590779));
#6901=CARTESIAN_POINT('Ctrl Pts',(11.2328897869991,28.5638932679152,4.6947457101671));
#6902=CARTESIAN_POINT('Ctrl Pts',(11.1233210874371,28.5750405741623,4.95690541002459));
#6903=CARTESIAN_POINT('Ctrl Pts',(11.0045543630941,28.5861878804094,5.21526682176328));
#6904=CARTESIAN_POINT('Ctrl Pts',(10.8768785996751,28.5973351866565,5.46918295341547));
#6905=CARTESIAN_POINT('Ctrl Pts',(10.7492245219682,28.6084805995351,5.72305595744509));
#6906=CARTESIAN_POINT('Ctrl Pts',(10.6126645460732,28.6196260124137,5.97248495058034));
#6907=CARTESIAN_POINT('Ctrl Pts',(10.467534458856,28.6307714252922,6.21684587251955));
#6908=CARTESIAN_POINT('Ctrl Pts',(10.3224204833328,28.6419156008568,6.46117966660059));
#6909=CARTESIAN_POINT('Ctrl Pts',(10.1687384324912,28.6530597764214,6.70044628368926));
#6910=CARTESIAN_POINT('Ctrl Pts',(10.0068690633192,28.664203951986,6.93404800961067));
#6911=CARTESIAN_POINT('Ctrl Pts',(9.83990209886954,28.6756990802789,7.17500632845005));
#6912=CARTESIAN_POINT('Ctrl Pts',(9.66422395039496,28.6871942085718,7.40993692714886));
#6913=CARTESIAN_POINT('Ctrl Pts',(9.48030035284617,28.6986893368646,7.63821677290091));
#6914=CARTESIAN_POINT('Ctrl Pts',(9.30198251686694,28.7098341080022,7.85953893403023));
#6915=CARTESIAN_POINT('Ctrl Pts',(9.11591458607458,28.7209788791398,8.0746095348416));
#6916=CARTESIAN_POINT('Ctrl Pts',(8.92256215039984,28.7321236502774,8.28289411511775));
#6917=CARTESIAN_POINT('Ctrl Pts',(8.72009211035867,28.7437939571479,8.50100043046518));
#6918=CARTESIAN_POINT('Ctrl Pts',(8.50963424411612,28.7554642640184,8.71166509837527));
#6919=CARTESIAN_POINT('Ctrl Pts',(8.29176759747592,28.7671345708889,8.91431659519946));
#6920=CARTESIAN_POINT('Ctrl Pts',(8.07390095083574,28.7788048777594,9.11696809202363));
#6921=CARTESIAN_POINT('Ctrl Pts',(7.84862577543433,28.7904751846298,9.31160619568754));
#6922=CARTESIAN_POINT('Ctrl Pts',(7.61656299213793,28.8021454915003,9.49770595653471));
#6923=CARTESIAN_POINT('Ctrl Pts',(7.39490001937539,28.8132927977474,9.67546572324015));
#6924=CARTESIAN_POINT('Ctrl Pts',(7.1669782326602,28.8244401039945,9.84548870117948));
#6925=CARTESIAN_POINT('Ctrl Pts',(6.93336099330262,28.8355874102417,10.0073450818161));
#6926=CARTESIAN_POINT('Ctrl Pts',(6.69978343380331,28.8467328231202,10.1691739711672));
#6927=CARTESIAN_POINT('Ctrl Pts',(6.4605125722004,28.8578782359988,10.3228388806969));
#6928=CARTESIAN_POINT('Ctrl Pts',(6.21614189045049,28.8690236488774,10.4679525336995));
#6929=CARTESIAN_POINT('Ctrl Pts',(5.97179833764248,28.880167824442,10.6130500768324));
#6930=CARTESIAN_POINT('Ctrl Pts',(5.72235632451495,28.8913120000066,10.7495981229213));
#6931=CARTESIAN_POINT('Ctrl Pts',(5.46843621193559,28.9024561755712,10.8772540489772));
#6932=CARTESIAN_POINT('Ctrl Pts',(5.20651963916487,28.913951303864,11.0089301194815));
#6933=CARTESIAN_POINT('Ctrl Pts',(4.93983860834559,28.9254464321569,11.1311447906857));
#6934=CARTESIAN_POINT('Ctrl Pts',(4.66910021250546,28.9369415604497,11.2435738737993));
#6935=CARTESIAN_POINT('Ctrl Pts',(4.40661358487263,28.9480863315873,11.3525762588609));
#6936=CARTESIAN_POINT('Ctrl Pts',(4.14031351438245,28.9592311027249,11.4523806207873));
#6937=CARTESIAN_POINT('Ctrl Pts',(3.87086458095965,28.9703758738625,11.5427404738161));
#6938=CARTESIAN_POINT('Ctrl Pts',(3.58870968516636,28.982046180733,11.6373612785503));
#6939=CARTESIAN_POINT('Ctrl Pts',(3.30310211058205,28.9937164876035,11.7216253225375));
#6940=CARTESIAN_POINT('Ctrl Pts',(3.01482379511558,29.005386794474,11.7953078694202));
#6941=CARTESIAN_POINT('Ctrl Pts',(2.72654547964909,29.0170571013444,11.8689904163028));
#6942=CARTESIAN_POINT('Ctrl Pts',(2.43559675052545,29.0287274082149,11.9320913915042));
#6943=CARTESIAN_POINT('Ctrl Pts',(2.14277402700613,29.0403977150854,11.9844469926312));
#6944=CARTESIAN_POINT('Ctrl Pts',(1.95948187699894,29.0477027343538,12.0172189393578));
#6945=CARTESIAN_POINT('Ctrl Pts',(1.77541980190147,29.0550077536222,12.0457883562595));
#6946=CARTESIAN_POINT('Ctrl Pts',(1.59078448392773,29.0623127728906,12.0701224093086));
#6947=CARTESIAN_POINT('Ctrl Pts',(1.59078448392775,26.0623070005467,12.0701224093086));
#6948=CARTESIAN_POINT('Ctrl Pts',(1.30899806788644,26.0734518121,12.1072605130676));
#6949=CARTESIAN_POINT('Ctrl Pts',(1.02591071152476,26.0845966236534,12.1345265044841));
#6950=CARTESIAN_POINT('Ctrl Pts',(0.742228150596408,26.0957414352068,12.1518536702209));
#6951=CARTESIAN_POINT('Ctrl Pts',(0.458543333616702,26.1068863353918,12.1691809737561));
#6952=CARTESIAN_POINT('Ctrl Pts',(0.174263569054537,26.1180312355769,12.1765692799692));
#6953=CARTESIAN_POINT('Ctrl Pts',(-0.109902562578879,26.129176135762,12.1740039295516));
#6954=CARTESIAN_POINT('Ctrl Pts',(-0.394127988996509,26.1403233614686,12.1714380438419));
#6955=CARTESIAN_POINT('Ctrl Pts',(-0.67823946826702,26.1514705871751,12.1589143533114));
#6956=CARTESIAN_POINT('Ctrl Pts',(-0.961529148741264,26.1626178128817,12.1364703248564));
#6957=CARTESIAN_POINT('Ctrl Pts',(-1.1203906032984,26.1688688859425,12.123884299836));
#6958=CARTESIAN_POINT('Ctrl Pts',(-1.27899367264829,26.1751199590034,12.1081795891686));
#6959=CARTESIAN_POINT('Ctrl Pts',(-1.43721416924489,26.1813710320642,12.089369945606));
#6960=CARTESIAN_POINT('Ctrl Pts',(-1.71936290002593,26.1925183383113,12.0558274073648));
#6961=CARTESIAN_POINT('Ctrl Pts',(-2.00037900433126,26.2036656445584,12.0123981199221));
#6962=CARTESIAN_POINT('Ctrl Pts',(-2.27956106827265,26.2148129508055,11.9591827306892));
#6963=CARTESIAN_POINT('Ctrl Pts',(-2.55869571317684,26.2259583636841,11.9059763800833));
#6964=CARTESIAN_POINT('Ctrl Pts',(-2.83599667771954,26.2371037765627,11.8429872961323));
#6965=CARTESIAN_POINT('Ctrl Pts',(-3.11077177834478,26.2482491894413,11.7703674196286));
#6966=CARTESIAN_POINT('Ctrl Pts',(-3.38551637466469,26.2593933650059,11.6977556050594));
#6967=CARTESIAN_POINT('Ctrl Pts',(-3.6577354091752,26.2705375405705,11.6155152010359));
#6968=CARTESIAN_POINT('Ctrl Pts',(-3.92674971414901,26.2816817161351,11.5238486163447));
#6969=CARTESIAN_POINT('Ctrl Pts',(-4.20423582609698,26.2931768444279,11.4292952646783));
#6970=CARTESIAN_POINT('Ctrl Pts',(-4.47831180682542,26.3046719727208,11.3247124991569));
#6971=CARTESIAN_POINT('Ctrl Pts',(-4.74825085465416,26.3161671010137,11.2103775168937));
#6972=CARTESIAN_POINT('Ctrl Pts',(-5.0099624974065,26.3273118721513,11.0995273221078));
#6973=CARTESIAN_POINT('Ctrl Pts',(-5.26778539315454,26.338456643289,10.9795106872953));
#6974=CARTESIAN_POINT('Ctrl Pts',(-5.52107796274178,26.3496014144266,10.8506289393439));
#6975=CARTESIAN_POINT('Ctrl Pts',(-5.78631463548921,26.3612717212971,10.7156697257349));
#6976=CARTESIAN_POINT('Ctrl Pts',(-6.04658315982574,26.3729420281675,10.5709893503964));
#6977=CARTESIAN_POINT('Ctrl Pts',(-6.30117522427093,26.384612335038,10.4169880984397));
#6978=CARTESIAN_POINT('Ctrl Pts',(-6.5557672887161,26.3962826419084,10.262986846483));
#6979=CARTESIAN_POINT('Ctrl Pts',(-6.80468261074529,26.4079529487789,10.0996648990647));
#6980=CARTESIAN_POINT('Ctrl Pts',(-7.04724619648092,26.4196232556493,9.92747557519963));
#6981=CARTESIAN_POINT('Ctrl Pts',(-7.27893938198356,26.4307705618965,9.76300285422281));
#6982=CARTESIAN_POINT('Ctrl Pts',(-7.50490681694821,26.4419178681436,9.59039094205251));
#6983=CARTESIAN_POINT('Ctrl Pts',(-7.72458077897762,26.4530651743908,9.41006387008343));
#6984=CARTESIAN_POINT('Ctrl Pts',(-7.9442174294129,26.4642105872694,9.22976742664427));
#6985=CARTESIAN_POINT('Ctrl Pts',(-8.15756253496308,26.4753560001481,9.04175860884122));
#6986=CARTESIAN_POINT('Ctrl Pts',(-8.36408102412932,26.4865014130267,8.84650206984658));
#6987=CARTESIAN_POINT('Ctrl Pts',(-8.57057658653295,26.4976455885913,8.65126720736302));
#6988=CARTESIAN_POINT('Ctrl Pts',(-8.77024685209962,26.5087897641558,8.44878641357831));
#6989=CARTESIAN_POINT('Ctrl Pts',(-8.96259232915518,26.5199339397204,8.23956242717833));
#6990=CARTESIAN_POINT('Ctrl Pts',(-9.16099515603928,26.5314290680132,8.0237495524013));
#6991=CARTESIAN_POINT('Ctrl Pts',(-9.35160416569127,26.542924196306,7.80076210097047));
#6992=CARTESIAN_POINT('Ctrl Pts',(-9.53391383017232,26.5544193245989,7.5711912754103));
#6993=CARTESIAN_POINT('Ctrl Pts',(-9.71066692374877,26.5655640957365,7.34861748192455));
#6994=CARTESIAN_POINT('Ctrl Pts',(-9.87961891449672,26.5767088668741,7.11985589637044));
#6995=CARTESIAN_POINT('Ctrl Pts',(-10.0403506524587,26.5878536380117,6.88547812614872));
#6996=CARTESIAN_POINT('Ctrl Pts',(-10.2086617539316,26.5995239448822,6.64004818700301));
#6997=CARTESIAN_POINT('Ctrl Pts',(-10.3679585107329,26.6111942517526,6.38845991414234));
#6998=CARTESIAN_POINT('Ctrl Pts',(-10.5178105333709,26.622864558623,6.13140374091549));
#6999=CARTESIAN_POINT('Ctrl Pts',(-10.6676625560089,26.6345348654935,5.87434756768864));
#7000=CARTESIAN_POINT('Ctrl Pts',(-10.8080696830999,26.6462051723639,5.61182378836291));
#7001=CARTESIAN_POINT('Ctrl Pts',(-10.9386561591369,26.6578754792344,5.34455345956773));
#7002=CARTESIAN_POINT('Ctrl Pts',(-11.0629966322907,26.6689875907038,5.09006677648294));
#7003=CARTESIAN_POINT('Ctrl Pts',(-11.1784731441786,26.6800997021732,4.83119636045063));
#7004=CARTESIAN_POINT('Ctrl Pts',(-11.284791078264,26.6912118136426,4.56858189922576));
#7005=CARTESIAN_POINT('Ctrl Pts',(-11.3910898863404,26.7023219261046,4.30601468089191));
#7006=CARTESIAN_POINT('Ctrl Pts',(-11.4882333044429,26.7134320385665,4.03970501227435));
#7007=CARTESIAN_POINT('Ctrl Pts',(-11.5759747961597,26.7245421510285,3.77031268844835));
#7008=CARTESIAN_POINT('Ctrl Pts',(-11.6637063953042,26.7356510108608,3.50095073774466));
#7009=CARTESIAN_POINT('Ctrl Pts',(-11.742038101081,26.7467598706931,3.22850708261955));
#7010=CARTESIAN_POINT('Ctrl Pts',(-11.8107728310722,26.7578687305254,2.95365796645564));
#7011=CARTESIAN_POINT('Ctrl Pts',(-11.8795114701164,26.7689782221362,2.67879321918694));
#7012=CARTESIAN_POINT('Ctrl Pts',(-11.938651974578,26.780087713747,2.40152299895952));
#7013=CARTESIAN_POINT('Ctrl Pts',(-11.9880477658973,26.7911972053578,2.12253645729935));
#7014=CARTESIAN_POINT('Ctrl Pts',(-12.0374432737353,26.8023066332115,1.84355151673624));
#7015=CARTESIAN_POINT('Ctrl Pts',(-12.0770941352764,26.8134160610651,1.56285054084612));
#7016=CARTESIAN_POINT('Ctrl Pts',(-12.1069051509043,26.8245254889188,1.28113149871751));
#7017=CARTESIAN_POINT('Ctrl Pts',(-12.136721994767,26.8356370887331,0.9993573788041));
#7018=CARTESIAN_POINT('Ctrl Pts',(-12.1566951200387,26.8467486885475,0.716565063644844));
#7019=CARTESIAN_POINT('Ctrl Pts',(-12.1667811943891,26.8578602883618,0.433457746337774));
#7020=CARTESIAN_POINT('Ctrl Pts',(-12.1719290135767,26.8635315242403,0.288962947910597));
#7021=CARTESIAN_POINT('Ctrl Pts',(-12.1745021246081,26.8692027601188,0.144386144645321));
#7022=CARTESIAN_POINT('Ctrl Pts',(-12.1744999986836,26.8748739959973,-0.000179033899942618));
#7023=CARTESIAN_POINT('',(-12.174499996235,26.6251260039329,-0.000302777009382115));
#7024=CARTESIAN_POINT('Ctrl Pts',(1.59078448392773,25.8125631998879,12.0701224093086));
#7025=CARTESIAN_POINT('Ctrl Pts',(1.30903389514245,25.8237068476434,12.1072557912064));
#7026=CARTESIAN_POINT('Ctrl Pts',(1.02597395944363,25.8348504953989,12.1345207225652));
#7027=CARTESIAN_POINT('Ctrl Pts',(0.742310031349682,25.8459941431544,12.1518486687153));
#7028=CARTESIAN_POINT('Ctrl Pts',(0.458617504427568,25.8571389144058,12.1691783618586));
#7029=CARTESIAN_POINT('Ctrl Pts',(0.174321129593775,25.8682836856572,12.1765690496002));
#7030=CARTESIAN_POINT('Ctrl Pts',(-0.109870438808507,25.8794284569086,12.1740042195112));
#7031=CARTESIAN_POINT('Ctrl Pts',(-0.394068654609052,25.8905734888424,12.1714393294294));
#7032=CARTESIAN_POINT('Ctrl Pts',(-0.678161792355716,25.9017185207762,12.1589184614899));
#7033=CARTESIAN_POINT('Ctrl Pts',(-0.961442061063879,25.91286355271,12.1364772241873));
#7034=CARTESIAN_POINT('Ctrl Pts',(-1.24477735406477,25.9240107494521,12.1140316279041));
#7035=CARTESIAN_POINT('Ctrl Pts',(-1.52729919663202,25.9351579461943,12.0816618336698));
#7036=CARTESIAN_POINT('Ctrl Pts',(-1.80830429338909,25.9463051429365,12.0394553793978));
#7037=CARTESIAN_POINT('Ctrl Pts',(-1.89233667555125,25.9496386251668,12.0268338684856));
#7038=CARTESIAN_POINT('Ctrl Pts',(-1.97623346896302,25.9529721073972,12.0133330526306));
#7039=CARTESIAN_POINT('Ctrl Pts',(-2.05997600562754,25.9563055896275,11.9989561673605));
#7040=CARTESIAN_POINT('Ctrl Pts',(-2.34001460716402,25.9674528958737,11.9508792520215));
#7041=CARTESIAN_POINT('Ctrl Pts',(-2.61841122728923,25.9786002021198,11.8929873201509));
#7042=CARTESIAN_POINT('Ctrl Pts',(-2.89447058977853,25.989747508366,11.8254171281569));
#7043=CARTESIAN_POINT('Ctrl Pts',(-3.17048306361892,26.0008929212436,11.7578584129518));
#7044=CARTESIAN_POINT('Ctrl Pts',(-3.44415881339921,26.0120383341212,11.6806247829667));
#7045=CARTESIAN_POINT('Ctrl Pts',(-3.71481443132733,26.0231837469987,11.5939037425193));
#7046=CARTESIAN_POINT('Ctrl Pts',(-3.98544000227735,26.0343279225623,11.5071923294544));
#7047=CARTESIAN_POINT('Ctrl Pts',(-4.25304585691818,26.0454720981259,11.4109956904718));
#7048=CARTESIAN_POINT('Ctrl Pts',(-4.51696419368029,26.0566162736895,11.30555105791));
#7049=CARTESIAN_POINT('Ctrl Pts',(-4.78919385506674,26.0681114019831,11.1967857596382));
#7050=CARTESIAN_POINT('Ctrl Pts',(-5.05749970102558,26.0796065302767,11.0781806539634));
#7051=CARTESIAN_POINT('Ctrl Pts',(-5.32117022412959,26.0911016585703,10.9500501229829));
#7052=CARTESIAN_POINT('Ctrl Pts',(-5.57680439892114,26.1022464297069,10.8258248505966));
#7053=CARTESIAN_POINT('Ctrl Pts',(-5.828081373454,26.1133912008435,10.6926463228308));
#7054=CARTESIAN_POINT('Ctrl Pts',(-6.07437599581028,26.12453597198,10.550848615705));
#7055=CARTESIAN_POINT('Ctrl Pts',(-6.33228473064399,26.1362062788521,10.4023643861377));
#7056=CARTESIAN_POINT('Ctrl Pts',(-6.58472964219707,26.1478765857242,10.2444286953485));
#7057=CARTESIAN_POINT('Ctrl Pts',(-6.83102404874258,26.1595468925963,10.0774778935754));
#7058=CARTESIAN_POINT('Ctrl Pts',(-7.07731845528811,26.1712171994684,9.91052709180227));
#7059=CARTESIAN_POINT('Ctrl Pts',(-7.31746208403958,26.1828875063405,9.73456137455852));
#7060=CARTESIAN_POINT('Ctrl Pts',(-7.55080426673173,26.1945578132126,9.55006833355165));
#7061=CARTESIAN_POINT('Ctrl Pts',(-7.77368930304789,26.2057051194604,9.37384328212515));
#7062=CARTESIAN_POINT('Ctrl Pts',(-7.99043566959423,26.2168524257083,9.18978577348594));
#7063=CARTESIAN_POINT('Ctrl Pts',(-8.20049831293366,26.2279997319561,8.99834860791536));
#7064=CARTESIAN_POINT('Ctrl Pts',(-8.41052527716152,26.2391451448355,8.80694395792146));
#7065=CARTESIAN_POINT('Ctrl Pts',(-8.61387058758587,26.2502905577149,8.60816233308373));
#7066=CARTESIAN_POINT('Ctrl Pts',(-8.81002389705792,26.2614359705943,8.40249541405816));
#7067=CARTESIAN_POINT('Ctrl Pts',(-9.00615543046492,26.2725801461596,8.19685132725613));
#7068=CARTESIAN_POINT('Ctrl Pts',(-9.19509637319099,26.283724321725,7.98432366558186));
#7069=CARTESIAN_POINT('Ctrl Pts',(-9.37637387833569,26.2948684972904,7.76544030584642));
#7070=CARTESIAN_POINT('Ctrl Pts',(-9.56336018036558,26.3063636255827,7.53966386447199));
#7071=CARTESIAN_POINT('Ctrl Pts',(-9.74219235219411,26.3178587538749,7.30712515292804));
#7072=CARTESIAN_POINT('Ctrl Pts',(-9.91239608982264,26.3293538821672,7.06844070559192));
#7073=CARTESIAN_POINT('Ctrl Pts',(-10.0774122300974,26.3404986533055,6.83703106211519));
#7074=CARTESIAN_POINT('Ctrl Pts',(-10.2343179534282,26.3516434244438,6.59984499127896));
#7075=CARTESIAN_POINT('Ctrl Pts',(-10.3827242058869,26.3627881955821,6.35747499519189));
#7076=CARTESIAN_POINT('Ctrl Pts',(-10.5381286090834,26.3744585024514,6.10367595390744));
#7077=CARTESIAN_POINT('Ctrl Pts',(-10.6842124964244,26.3861288093207,5.84419259488536));
#7078=CARTESIAN_POINT('Ctrl Pts',(-10.8205817294359,26.3977991161899,5.57973666821271));
#7079=CARTESIAN_POINT('Ctrl Pts',(-10.9569509624474,26.4094694230592,5.31528074154007));
#7080=CARTESIAN_POINT('Ctrl Pts',(-11.0836053951668,26.4211397299285,5.04585254943003));
#7081=CARTESIAN_POINT('Ctrl Pts',(-11.2002070324854,26.4328100367977,4.77219160129437));
#7082=CARTESIAN_POINT('Ctrl Pts',(-11.311144830923,26.4439134670834,4.51182353269197));
#7083=CARTESIAN_POINT('Ctrl Pts',(-11.4130186487047,26.4550168973691,4.24754059388121));
#7084=CARTESIAN_POINT('Ctrl Pts',(-11.5055675162661,26.4661203276549,3.97999577620921));
#7085=CARTESIAN_POINT('Ctrl Pts',(-11.5980993129953,26.4772217098896,3.71250030773821));
#7086=CARTESIAN_POINT('Ctrl Pts',(-11.6813095047598,26.4883230921244,3.44174441751769));
#7087=CARTESIAN_POINT('Ctrl Pts',(-11.7549861724547,26.4994244743592,3.16839870208905));
#7088=CARTESIAN_POINT('Ctrl Pts',(-11.8286604607754,26.5105254980769,2.89506181430902));
#7089=CARTESIAN_POINT('Ctrl Pts',(-11.8928017662328,26.5216265217947,2.61913552911646));
#7090=CARTESIAN_POINT('Ctrl Pts',(-11.9472483674234,26.5327275455124,2.34130448619971));
#7091=CARTESIAN_POINT('Ctrl Pts',(-12.0016914005901,26.5438278417519,2.06349165025601));
#7092=CARTESIAN_POINT('Ctrl Pts',(-12.0464409474768,26.5549281379914,1.78377457205652));
#7093=CARTESIAN_POINT('Ctrl Pts',(-12.0813864435219,26.5660284342308,1.50284791389073));
#7094=CARTESIAN_POINT('Ctrl Pts',(-12.1163370539098,26.5771303550208,1.22188014154935));
#7095=CARTESIAN_POINT('Ctrl Pts',(-12.1414807111354,26.5882322758107,0.939702704299309));
#7096=CARTESIAN_POINT('Ctrl Pts',(-12.1567585846212,26.5993341966006,0.657016716103665));
#7097=CARTESIAN_POINT('Ctrl Pts',(-12.1685896895518,26.6079314657114,0.438106172572895));
#7098=CARTESIAN_POINT('Ctrl Pts',(-12.1745054475292,26.6165287348221,0.218890818353648));
#7099=CARTESIAN_POINT('Ctrl Pts',(-12.174499996235,26.6251260039329,-0.000302777009381836));
#7100=CARTESIAN_POINT('Ctrl Pts',(-12.174499996235,26.6251260039651,-0.000302777830488094));
#7101=CARTESIAN_POINT('Ctrl Pts',(-12.1744924727439,26.6369913152146,-0.302817471666667));
#7102=CARTESIAN_POINT('Ctrl Pts',(-12.1632051823574,26.648856626464,-0.605278801658912));
#7103=CARTESIAN_POINT('Ctrl Pts',(-12.1406760102577,26.6607219377135,-0.906882717860236));
#7104=CARTESIAN_POINT('Ctrl Pts',(-12.1341314731588,26.6641687119366,-0.994496146796198));
#7105=CARTESIAN_POINT('Ctrl Pts',(-12.1266386202186,26.6676154861597,-1.08203724349874));
#7106=CARTESIAN_POINT('Ctrl Pts',(-12.1181992022146,26.6710622603828,-1.16948635966588));
#7107=CARTESIAN_POINT('Ctrl Pts',(-12.0909050509449,26.6822095666301,-1.45230792437143));
#7108=CARTESIAN_POINT('Ctrl Pts',(-12.0537015189063,26.6933568728774,-1.73421580133404));
#7109=CARTESIAN_POINT('Ctrl Pts',(-12.0066737159719,26.7045041791248,-2.01450652225056));
#7110=CARTESIAN_POINT('Ctrl Pts',(-11.9596539007038,26.7156495920035,-2.29474963582362));
#7111=CARTESIAN_POINT('Ctrl Pts',(-11.9028131901233,26.7267950048823,-2.57337587876628));
#7112=CARTESIAN_POINT('Ctrl Pts',(-11.8362881790818,26.737940417761,-2.84968987641259));
#7113=CARTESIAN_POINT('Ctrl Pts',(-11.7697705533498,26.7490845933258,-3.12597319891336));
#7114=CARTESIAN_POINT('Ctrl Pts',(-11.6935708363978,26.7602287688906,-3.39994452942677));
#7115=CARTESIAN_POINT('Ctrl Pts',(-11.6078763665936,26.7713729444554,-3.67092038974925));
#7116=CARTESIAN_POINT('Ctrl Pts',(-11.5194832038473,26.7828680727481,-3.95042983039985));
#7117=CARTESIAN_POINT('Ctrl Pts',(-11.4209876598191,26.7943632010408,-4.22675179091095));
#7118=CARTESIAN_POINT('Ctrl Pts',(-11.3126507894069,26.8058583293335,-4.49915351671094));
#7119=CARTESIAN_POINT('Ctrl Pts',(-11.2076158915104,26.8170031004714,-4.763252778092));
#7120=CARTESIAN_POINT('Ctrl Pts',(-11.0933307897004,26.8281478716092,-5.02366697453654));
#7121=CARTESIAN_POINT('Ctrl Pts',(-10.9700825475829,26.839292642747,-5.27974801948126));
#7122=CARTESIAN_POINT('Ctrl Pts',(-10.8410224898273,26.8509629496171,-5.54790465914499));
#7123=CARTESIAN_POINT('Ctrl Pts',(-10.7021337694083,26.8626332564873,-5.81130936507168));
#7124=CARTESIAN_POINT('Ctrl Pts',(-10.553800908055,26.8743035633574,-6.06924514607354));
#7125=CARTESIAN_POINT('Ctrl Pts',(-10.4054680467018,26.8859738702276,-6.32718092707538));
#7126=CARTESIAN_POINT('Ctrl Pts',(-10.2476912192782,26.8976441770977,-6.57964749669029));
#7127=CARTESIAN_POINT('Ctrl Pts',(-10.0809087053182,26.9093144839679,-6.82596000025198));
#7128=CARTESIAN_POINT('Ctrl Pts',(-9.92160048999432,26.9204617902149,-7.06123409717429));
#7129=CARTESIAN_POINT('Ctrl Pts',(-9.75402843997352,26.931609096462,-7.29096385566852));
#7130=CARTESIAN_POINT('Ctrl Pts',(-9.57860392681835,26.9427564027091,-7.51457231405355));
#7131=CARTESIAN_POINT('Ctrl Pts',(-9.40320920949447,26.9539018155876,-7.73814279257031));
#7132=CARTESIAN_POINT('Ctrl Pts',(-9.2199648564318,26.9650472284661,-7.95559383695199));
#7133=CARTESIAN_POINT('Ctrl Pts',(-9.02932357316257,26.9761926413446,-8.16638023001199));
#7134=CARTESIAN_POINT('Ctrl Pts',(-8.83870345403747,26.9873368169091,-8.37714322250773));
#7135=CARTESIAN_POINT('Ctrl Pts',(-8.64068822334226,26.9984809924736,-8.58124284331955));
#7136=CARTESIAN_POINT('Ctrl Pts',(-8.43576944971309,27.0096251680382,-8.77816860405902));
#7137=CARTESIAN_POINT('Ctrl Pts',(-8.22439736760149,27.0211202963311,-8.98129595706688));
#7138=CARTESIAN_POINT('Ctrl Pts',(-8.00568009069493,27.032615424624,-9.17679007677322));
#7139=CARTESIAN_POINT('Ctrl Pts',(-7.78019749632778,27.0441105529169,-9.36413248347838));
#7140=CARTESIAN_POINT('Ctrl Pts',(-7.56158732985657,27.0552553240544,-9.54576492757846));
#7141=CARTESIAN_POINT('Ctrl Pts',(-7.3366183506728,27.066400095192,-9.71973503020182));
#7142=CARTESIAN_POINT('Ctrl Pts',(-7.10585275617098,27.0775448663295,-9.88561110188022));
#7143=CARTESIAN_POINT('Ctrl Pts',(-6.86420532619913,27.0892151732001,-10.0593091199987));
#7144=CARTESIAN_POINT('Ctrl Pts',(-6.61620170182717,27.1008854800707,-10.2241312000397));
#7145=CARTESIAN_POINT('Ctrl Pts',(-6.3625226287518,27.1125557869413,-10.3796317877187));
#7146=CARTESIAN_POINT('Ctrl Pts',(-6.10884355567643,27.1242260938118,-10.5351323753978));
#7147=CARTESIAN_POINT('Ctrl Pts',(-5.84948932452369,27.1358964006824,-10.6813113028628));
#7148=CARTESIAN_POINT('Ctrl Pts',(-5.58517250510067,27.147566707553,-10.8177769591662));
#7149=CARTESIAN_POINT('Ctrl Pts',(-5.33270094929267,27.1587140138001,-10.9481269559485));
#7150=CARTESIAN_POINT('Ctrl Pts',(-5.07562641811087,27.1698613200473,-11.0696540694031));
#7151=CARTESIAN_POINT('Ctrl Pts',(-4.81458622303291,27.1810086262944,-11.1820485489458));
#7152=CARTESIAN_POINT('Ctrl Pts',(-4.55359036559887,27.192154039173,-11.2944239383005));
#7153=CARTESIAN_POINT('Ctrl Pts',(-4.28863043395543,27.2032994520515,-11.397669685218));
#7154=CARTESIAN_POINT('Ctrl Pts',(-4.02036484236643,27.2144448649301,-11.4915236928905));
#7155=CARTESIAN_POINT('Ctrl Pts',(-3.75212903242545,27.2255890404947,-11.5853672813102));
#7156=CARTESIAN_POINT('Ctrl Pts',(-3.48058854705728,27.2367332160593,-11.6698211243842));
#7157=CARTESIAN_POINT('Ctrl Pts',(-3.20641930561617,27.2478773916239,-11.7446722170766));
#7158=CARTESIAN_POINT('Ctrl Pts',(-2.92361591777954,27.2593725199168,-11.8218805227401));
#7159=CARTESIAN_POINT('Ctrl Pts',(-2.63801580485302,27.2708676482096,-11.8888713695227));
#7160=CARTESIAN_POINT('Ctrl Pts',(-2.35037625108813,27.2823627765025,-11.9454669949869));
#7161=CARTESIAN_POINT('Ctrl Pts',(-2.07150359171745,27.2935075476401,-12.0003376564636));
#7162=CARTESIAN_POINT('Ctrl Pts',(-1.79071424363557,27.3046523187777,-12.0454373261581));
#7163=CARTESIAN_POINT('Ctrl Pts',(-1.50870843413845,27.3157970899153,-12.0806559884288));
#7164=CARTESIAN_POINT('Ctrl Pts',(-1.21340453821725,27.3274673967858,-12.1175353995168));
#7165=CARTESIAN_POINT('Ctrl Pts',(-0.916767010429212,27.3391377036562,-12.1435794559706));
#7166=CARTESIAN_POINT('Ctrl Pts',(-0.619606806006443,27.3508080105267,-12.1587226983738));
#7167=CARTESIAN_POINT('Ctrl Pts',(-0.322446601583674,27.3624783173972,-12.173865940777));
#7168=CARTESIAN_POINT('Ctrl Pts',(-0.0247640560390245,27.3741486242676,
-12.1781083608214));
#7169=CARTESIAN_POINT('Ctrl Pts',(0.272627745971015,27.3858189311381,-12.1714470940035));
#7170=CARTESIAN_POINT('Ctrl Pts',(0.556692040867883,27.3969662373852,-12.1650843494728));
#7171=CARTESIAN_POINT('Ctrl Pts',(0.840575917591387,27.4081135436323,-12.1487718259602));
#7172=CARTESIAN_POINT('Ctrl Pts',(1.12357154681536,27.4192608498795,-12.1225425232988));
#7173=CARTESIAN_POINT('Ctrl Pts',(1.40651910926765,27.430406262758,-12.0963176756811));
#7174=CARTESIAN_POINT('Ctrl Pts',(1.68857845992167,27.4415516756366,-12.0601794363548));
#7175=CARTESIAN_POINT('Ctrl Pts',(1.96904604421539,27.4526970885152,-12.0142127468162));
#7176=CARTESIAN_POINT('Ctrl Pts',(2.24948249224993,27.4638412640798,-11.9682511602942));
#7177=CARTESIAN_POINT('Ctrl Pts',(2.52832726361977,27.4749854396443,-11.9124633454658));
#7178=CARTESIAN_POINT('Ctrl Pts',(2.80488492567751,27.4861296152089,-11.8469857264921));
#7179=CARTESIAN_POINT('Ctrl Pts',(3.09015195034895,27.4976247435018,-11.7794460842771));
#7180=CARTESIAN_POINT('Ctrl Pts',(3.37298518903564,27.5091198717946,-11.7015965039929));
#7181=CARTESIAN_POINT('Ctrl Pts',(3.65263463056838,27.5206150000875,-11.6136432916451));
#7182=CARTESIAN_POINT('Ctrl Pts',(3.92376070634925,27.5317597712251,-11.5283707833737));
#7183=CARTESIAN_POINT('Ctrl Pts',(4.19189392120749,27.5429045423627,-11.4336014988325));
#7184=CARTESIAN_POINT('Ctrl Pts',(4.4563667833834,27.5540493135003,-11.329573925879));
#7185=CARTESIAN_POINT('Ctrl Pts',(4.73331095948184,27.5657196203708,-11.2206408949203));
#7186=CARTESIAN_POINT('Ctrl Pts',(5.00624097019272,27.5773899272413,-11.1015555262876));
#7187=CARTESIAN_POINT('Ctrl Pts',(5.27441341956718,27.5890602341118,-10.9726484191142));
#7188=CARTESIAN_POINT('Ctrl Pts',(5.54258586894163,27.6007305409822,-10.8437413119408));
#7189=CARTESIAN_POINT('Ctrl Pts',(5.80600045840199,27.6124008478527,-10.7050126194888));
#7190=CARTESIAN_POINT('Ctrl Pts',(6.06394187656684,27.6240711547232,-10.5568489222693));
#7191=CARTESIAN_POINT('Ctrl Pts',(6.31032374244294,27.6352184609703,-10.4153251280848));
#7192=CARTESIAN_POINT('Ctrl Pts',(6.55178579543794,27.6463657672174,-10.2651511261732));
#7193=CARTESIAN_POINT('Ctrl Pts',(6.78772230773284,27.6575130734645,-10.1066946190684));
#7194=CARTESIAN_POINT('Ctrl Pts',(7.02361874624126,27.6686584863431,-9.94826502578106));
#7195=CARTESIAN_POINT('Ctrl Pts',(7.25399129643232,27.6798038992216,-9.78155588460602));
#7196=CARTESIAN_POINT('Ctrl Pts',(7.47826284030866,27.6909493121002,-9.60697846053892));
#7197=CARTESIAN_POINT('Ctrl Pts',(7.70250948655965,27.7020934876648,-9.43242041727788));
#7198=CARTESIAN_POINT('Ctrl Pts',(7.92065626853127,27.7132376632294,-9.24999599917782));
#7199=CARTESIAN_POINT('Ctrl Pts',(8.13215783644281,27.724381838794,-9.06015778964041));
#7200=CARTESIAN_POINT('Ctrl Pts',(8.35032001839985,27.7358769670868,-8.86434118922249));
#7201=CARTESIAN_POINT('Ctrl Pts',(8.56141143418563,27.7473720953797,-8.66063647097069));
#7202=CARTESIAN_POINT('Ctrl Pts',(8.76487225201568,27.7588672236726,-8.44958369719158));
#7203=CARTESIAN_POINT('Ctrl Pts',(8.96213183819983,27.7700119948102,-8.24496354839487));
#7204=CARTESIAN_POINT('Ctrl Pts',(9.15221888712477,27.7811567659477,-8.03343683132685));
#7205=CARTESIAN_POINT('Ctrl Pts',(9.33466142474239,27.7923015370853,-7.81553237696745));
#7206=CARTESIAN_POINT('Ctrl Pts',(9.52570710651933,27.8039718439558,-7.58735255887823));
#7207=CARTESIAN_POINT('Ctrl Pts',(9.70836976594012,27.8156421508263,-7.35217928526387));
#7208=CARTESIAN_POINT('Ctrl Pts',(9.8821548593783,27.8273124576968,-7.11065859012131));
#7209=CARTESIAN_POINT('Ctrl Pts',(10.0559399528165,27.8389827645673,-6.86913789497875));
#7210=CARTESIAN_POINT('Ctrl Pts',(10.2208472914441,27.8506530714378,-6.62127005576414));
#7211=CARTESIAN_POINT('Ctrl Pts',(10.3764337811701,27.8623233783083,-6.36773682205794));
#7212=CARTESIAN_POINT('Ctrl Pts',(10.5250477180731,27.8734706845554,-6.12556558943235));
#7213=CARTESIAN_POINT('Ctrl Pts',(10.6652022492297,27.8846179908025,-5.87815325893289));
#7214=CARTESIAN_POINT('Ctrl Pts',(10.7965414680425,27.8957652970496,-5.62611256364813));
#7215=CARTESIAN_POINT('Ctrl Pts',(10.9278583789057,27.9069107099282,-5.37411467744332));
#7216=CARTESIAN_POINT('Ctrl Pts',(11.0503628435203,27.9180561228068,-5.11749023242191));
#7217=CARTESIAN_POINT('Ctrl Pts',(11.1637449230495,27.9292015356854,-4.85687652129296));
#7218=CARTESIAN_POINT('Ctrl Pts',(11.2771144154065,27.94034571125,-4.59629174233456));
#7219=CARTESIAN_POINT('Ctrl Pts',(11.3813634385435,27.9514898868146,-4.33171882614916));
#7220=CARTESIAN_POINT('Ctrl Pts',(11.4762297207817,27.9626340623792,-4.06381614321401));
#7221=CARTESIAN_POINT('Ctrl Pts',(11.5740835349712,27.974129190672,-3.78747666054106));
#7222=CARTESIAN_POINT('Ctrl Pts',(11.6619539607177,27.9856243189649,-3.50759456690958));
#7223=CARTESIAN_POINT('Ctrl Pts',(11.7396078726036,27.9971194472577,-3.22491197515578));
#7224=CARTESIAN_POINT('Ctrl Pts',(11.8148949902295,28.0082642183954,-2.95084519578453));
#7225=CARTESIAN_POINT('Ctrl Pts',(11.8805790712358,28.019408989533,-2.67414637087711));
#7226=CARTESIAN_POINT('Ctrl Pts',(11.9364987602759,28.0305537606706,-2.39550570776437));
#7227=CARTESIAN_POINT('Ctrl Pts',(11.9950553625732,28.042224067541,-2.1037256429279));
#7228=CARTESIAN_POINT('Ctrl Pts',(12.0429044652634,28.0538943744115,-1.80981650877137));
#7229=CARTESIAN_POINT('Ctrl Pts',(12.0799209821079,28.065564681282,-1.51458222491547));
#7230=CARTESIAN_POINT('Ctrl Pts',(12.1169374989523,28.0772349881525,-1.21934794105957));
#7231=CARTESIAN_POINT('Ctrl Pts',(12.1431213969226,28.0889052950229,-0.922788841490883));
#7232=CARTESIAN_POINT('Ctrl Pts',(12.158409857211,28.1005756018934,-0.625715585608539));
#7233=CARTESIAN_POINT('Ctrl Pts',(12.1730131706264,28.1117229081405,-0.34195556130913));
#7234=CARTESIAN_POINT('Ctrl Pts',(12.1776804928749,28.1228702143876,-0.0576417030646985));
#7235=CARTESIAN_POINT('Ctrl Pts',(12.1723925340344,28.1340175206348,0.226517653580774));
#7236=CARTESIAN_POINT('Ctrl Pts',(12.167105473353,28.1451629335133,0.510628745795714));
#7237=CARTESIAN_POINT('Ctrl Pts',(12.1518665124317,28.1563083463919,0.794585122204064));
#7238=CARTESIAN_POINT('Ctrl Pts',(12.126708476824,28.1674537592705,1.07767887987282));
#7239=CARTESIAN_POINT('Ctrl Pts',(12.1015532341492,28.1785979348351,1.36074120973675));
#7240=CARTESIAN_POINT('Ctrl Pts',(12.0664811392585,28.1897421103997,1.64294084645477));
#7241=CARTESIAN_POINT('Ctrl Pts',(12.0215769591466,28.2008862859643,1.92357419022913));
#7242=CARTESIAN_POINT('Ctrl Pts',(11.9752586551788,28.2123814142571,2.21304524811395));
#7243=CARTESIAN_POINT('Ctrl Pts',(11.9184790037928,28.22387654255,2.50084946845287));
#7244=CARTESIAN_POINT('Ctrl Pts',(11.8513884385692,28.2353716708428,2.78622366800464));
#7245=CARTESIAN_POINT('Ctrl Pts',(11.7863427099908,28.2465164419804,3.06290001832938));
#7246=CARTESIAN_POINT('Ctrl Pts',(11.711605351783,28.257661213118,3.33729201072506));
#7247=CARTESIAN_POINT('Ctrl Pts',(11.6273649772611,28.2688059842556,3.60871638336431));
#7248=CARTESIAN_POINT('Ctrl Pts',(11.5391522172666,28.2804762911261,3.89293987092784));
#7249=CARTESIAN_POINT('Ctrl Pts',(11.4405187337417,28.2921465979966,4.1739088224095));
#7250=CARTESIAN_POINT('Ctrl Pts',(11.3317394027964,28.3038169048671,4.4508574855988));
#7251=CARTESIAN_POINT('Ctrl Pts',(11.2229600718511,28.3154872117375,4.72780614878812));
#7252=CARTESIAN_POINT('Ctrl Pts',(11.1040350243111,28.327157518608,5.00073421461789));
#7253=CARTESIAN_POINT('Ctrl Pts',(10.9752970363654,28.3388278254785,5.26889981054376));
#7254=CARTESIAN_POINT('Ctrl Pts',(10.8523283952496,28.3499751317256,5.52504766131596));
#7255=CARTESIAN_POINT('Ctrl Pts',(10.7203702820013,28.3611224379727,5.77692701782369));
#7256=CARTESIAN_POINT('Ctrl Pts',(10.5797447276347,28.3722697442198,6.02390668487535));
#7257=CARTESIAN_POINT('Ctrl Pts',(10.4391430585005,28.3834151570984,6.2708444024621));
#7258=CARTESIAN_POINT('Ctrl Pts',(10.2898770193584,28.394560569977,6.51288386038532));
#7259=CARTESIAN_POINT('Ctrl Pts',(10.1323141949373,28.4057059828556,6.74941918279437));
#7260=CARTESIAN_POINT('Ctrl Pts',(9.97476886243759,28.4168501584201,6.98592824610783));
#7261=CARTESIAN_POINT('Ctrl Pts',(9.80892873173758,28.4279943339847,7.21693417212062));
#7262=CARTESIAN_POINT('Ctrl Pts',(9.63520493625646,28.4391385095493,7.44185971960901));
#7263=CARTESIAN_POINT('Ctrl Pts',(9.45601022553033,28.4506336378422,7.67386862953109));
#7264=CARTESIAN_POINT('Ctrl Pts',(9.26842743225017,28.462128766135,7.89940774747224));
#7265=CARTESIAN_POINT('Ctrl Pts',(9.07295386254082,28.4736238944279,8.11787893838075));
#7266=CARTESIAN_POINT('Ctrl Pts',(8.88343808312899,28.4847686655655,8.32969140021698));
#7267=CARTESIAN_POINT('Ctrl Pts',(8.68650559273321,28.4959134367031,8.53486019031224));
#7268=CARTESIAN_POINT('Ctrl Pts',(8.48264897593018,28.5070582078407,8.73287562038706));
#7269=CARTESIAN_POINT('Ctrl Pts',(8.26917942628235,28.5187285147112,8.94022854002387));
#7270=CARTESIAN_POINT('Ctrl Pts',(8.04811724601421,28.5303988215817,9.13973700657147));
#7271=CARTESIAN_POINT('Ctrl Pts',(7.82007023915216,28.5420691284521,9.33086018032243));
#7272=CARTESIAN_POINT('Ctrl Pts',(7.59202323229009,28.5537394353226,9.5219833540734));
#7273=CARTESIAN_POINT('Ctrl Pts',(7.35699166160939,28.5654097421931,9.70472102625257));
#7274=CARTESIAN_POINT('Ctrl Pts',(7.1156227436877,28.5770800490636,9.87858103269464));
#7275=CARTESIAN_POINT('Ctrl Pts',(6.88507088945431,28.5882273455408,10.0446494196576));
#7276=CARTESIAN_POINT('Ctrl Pts',(6.64866836787934,28.5993746420181,10.202667962098));
#7277=CARTESIAN_POINT('Ctrl Pts',(6.4069999951961,28.6105219384953,10.3522365366889));
#7278=CARTESIAN_POINT('Ctrl Pts',(6.1653727278874,28.6216673389289,10.5017796711604));
#7279=CARTESIAN_POINT('Ctrl Pts',(5.91848162441142,28.6328127393624,10.6428755669444));
#7280=CARTESIAN_POINT('Ctrl Pts',(5.66693938316602,28.6439581397959,10.7751681322159));
#7281=CARTESIAN_POINT('Ctrl Pts',(5.41542512736357,28.655102300243,10.9074459792198));
#7282=CARTESIAN_POINT('Ctrl Pts',(5.15926100311546,28.6662464606901,11.0309223273304));
#7283=CARTESIAN_POINT('Ctrl Pts',(4.89908424391283,28.6773906211372,11.1452870676822));
#7284=CARTESIAN_POINT('Ctrl Pts',(4.63611072826147,28.6886545751535,11.2608811658217));
#7285=CARTESIAN_POINT('Ctrl Pts',(4.36903806075543,28.6999185291697,11.3671665133374));
#7286=CARTESIAN_POINT('Ctrl Pts',(4.09854619613597,28.711182483186,11.4638723530986));
#7287=CARTESIAN_POINT('Ctrl Pts',(3.83091820433177,28.7223271784151,11.5595543054096));
#7288=CARTESIAN_POINT('Ctrl Pts',(3.5599433215539,28.7334718736442,11.6458585229986));
#7289=CARTESIAN_POINT('Ctrl Pts',(3.28629764156213,28.7446165688734,11.7225721606251));
#7290=CARTESIAN_POINT('Ctrl Pts',(3.00825955990872,28.7559401522832,11.8005171610467));
#7291=CARTESIAN_POINT('Ctrl Pts',(2.72746448770561,28.767263735693,11.8685610136402));
#7292=CARTESIAN_POINT('Ctrl Pts',(2.44463594005741,28.7785873191028,11.9265336695362));
#7293=CARTESIAN_POINT('Ctrl Pts',(2.16180739240921,28.7899109025126,11.9845063254321));
#7294=CARTESIAN_POINT('Ctrl Pts',(1.87694565348214,28.8012344859224,12.0324077339315));
#7295=CARTESIAN_POINT('Ctrl Pts',(1.59078448392775,28.8125580693322,12.0701224093086));
#7296=CARTESIAN_POINT('Origin',(0.,13.3748739960349,0.));
#7297=CARTESIAN_POINT('',(1.59071714630986,32.0622959365534,12.0696162300787));
#7298=CARTESIAN_POINT('',(1.59078448392771,31.8125557231064,12.0701224093087));
#7299=CARTESIAN_POINT('',(1.59078448392774,13.3748739960349,12.0701224093086));
#7300=CARTESIAN_POINT('',(-12.174396721221,29.8748739960031,-4.71261348963091E-6));
#7301=CARTESIAN_POINT('Ctrl Pts',(-12.1734593809614,29.8748739960349,-4.71306082890088E-6));
#7302=CARTESIAN_POINT('Ctrl Pts',(-12.1734729483294,29.9143848671652,-1.00768895467666));
#7303=CARTESIAN_POINT('Ctrl Pts',(-11.8010964029253,30.0333131461572,-4.04082287428804));
#7304=CARTESIAN_POINT('Ctrl Pts',(-9.30992091872449,30.2316588330109,-8.62536224638919));
#7305=CARTESIAN_POINT('Ctrl Pts',(-4.04710485413492,30.469911056596,-12.0288172192438));
#7306=CARTESIAN_POINT('Ctrl Pts',(2.2026844913737,30.7081632801811,-12.4987872382004));
#7307=CARTESIAN_POINT('Ctrl Pts',(7.91530200229061,30.9464155037662,-9.92066003887209));
#7308=CARTESIAN_POINT('Ctrl Pts',(11.6976034309138,31.1846677273513,-4.92316720896363));
#7309=CARTESIAN_POINT('Ctrl Pts',(12.6271934885173,31.4229199509364,1.27494548820119));
#7310=CARTESIAN_POINT('Ctrl Pts',(10.4773717109103,31.6611721745215,7.16213539565936));
#7311=CARTESIAN_POINT('Ctrl Pts',(6.26861872634805,31.8742975030605,10.866008505099));
#7312=CARTESIAN_POINT('Ctrl Pts',(2.96313964180942,32.0080054237378,11.8875089580627));
#7313=CARTESIAN_POINT('Ctrl Pts',(1.59071714630986,32.0622959365534,12.0696162300787));
#7314=CARTESIAN_POINT('Ctrl Pts',(1.59078448392773,29.0623127728906,12.0701224093086));
#7315=CARTESIAN_POINT('Ctrl Pts',(1.30906809259831,29.0734587642939,12.107251284145));
#7316=CARTESIAN_POINT('Ctrl Pts',(1.02601695318895,29.0846047556973,12.1345174913886));
#7317=CARTESIAN_POINT('Ctrl Pts',(0.742335843504071,29.0957507471006,12.1518470919218));
#7318=CARTESIAN_POINT('Ctrl Pts',(0.458691979131175,29.1068952751145,12.1691744172018));
#7319=CARTESIAN_POINT('Ctrl Pts',(0.174418575804354,29.1180398031285,12.176567724411));
#7320=CARTESIAN_POINT('Ctrl Pts',(-0.109776022248343,29.1291843311424,12.1740050712549));
#7321=CARTESIAN_POINT('Ctrl Pts',(-0.3939500234525,29.1403280514627,12.1714426038256));
#7322=CARTESIAN_POINT('Ctrl Pts',(-0.67804496411194,29.1514717717831,12.1589256196025));
#7323=CARTESIAN_POINT('Ctrl Pts',(-0.961352806067982,29.1626154921034,12.1364842945667));
#7324=CARTESIAN_POINT('Ctrl Pts',(-1.24468790631768,29.1737602846101,12.1140408103524));
#7325=CARTESIAN_POINT('Ctrl Pts',(-1.52723549039379,29.1849050771168,12.0816710959945));
#7326=CARTESIAN_POINT('Ctrl Pts',(-1.80829146499432,29.1960498696235,12.0394573061924));
#7327=CARTESIAN_POINT('Ctrl Pts',(-2.08935117658927,29.2071948103143,11.9972429551045));
#7328=CARTESIAN_POINT('Ctrl Pts',(-2.36891897565992,29.2183397510051,11.945184309298));
#7329=CARTESIAN_POINT('Ctrl Pts',(-2.64629886222554,29.2294846916959,11.8834150218607));
#7330=CARTESIAN_POINT('Ctrl Pts',(-2.92373516566913,29.2406318991796,11.8216331710381));
#7331=CARTESIAN_POINT('Ctrl Pts',(-3.19898240695043,29.2517791066633,11.7501367899863));
#7332=CARTESIAN_POINT('Ctrl Pts',(-3.47135621080027,29.262926314147,11.6691103477402));
#7333=CARTESIAN_POINT('Ctrl Pts',(-3.59942127187903,29.2681675223215,11.6310132322006));
#7334=CARTESIAN_POINT('Ctrl Pts',(-3.72685129803498,29.273408730496,11.5908100241812));
#7335=CARTESIAN_POINT('Ctrl Pts',(-3.85357632161499,29.2786499386705,11.5485237058028));
#7336=CARTESIAN_POINT('Ctrl Pts',(-4.12310246901941,29.2897972449176,11.4585867055287));
#7337=CARTESIAN_POINT('Ctrl Pts',(-4.38951899259722,29.3009445511647,11.3591966162271));
#7338=CARTESIAN_POINT('Ctrl Pts',(-4.6521593504558,29.3120918574118,11.2505939233432));
#7339=CARTESIAN_POINT('Ctrl Pts',(-4.91475509888349,29.3232372702904,11.1420096766126));
#7340=CARTESIAN_POINT('Ctrl Pts',(-5.17357571569878,29.334382683169,11.0242160522333));
#7341=CARTESIAN_POINT('Ctrl Pts',(-5.42797407681333,29.3455280960475,10.8975019005019));
#7342=CARTESIAN_POINT('Ctrl Pts',(-5.6823441957571,29.3566722716121,10.7708018160101));
#7343=CARTESIAN_POINT('Ctrl Pts',(-5.93229280062091,29.3678164471767,10.6351833005704));
#7344=CARTESIAN_POINT('Ctrl Pts',(-6.17719572531667,29.3789606227413,10.4909819950818));
#7345=CARTESIAN_POINT('Ctrl Pts',(-6.42981114063938,29.3904557510341,10.3422394975337));
#7346=CARTESIAN_POINT('Ctrl Pts',(-6.67705766802888,29.401950879327,10.1843650133687));
#7347=CARTESIAN_POINT('Ctrl Pts',(-6.91827962488502,29.4134460076199,10.0177770628968));
#7348=CARTESIAN_POINT('Ctrl Pts',(-7.15214943773397,29.4245907787575,9.85626650512033));
#7349=CARTESIAN_POINT('Ctrl Pts',(-7.38035625506969,29.435735549895,9.68656592549784));
#7350=CARTESIAN_POINT('Ctrl Pts',(-7.60233273639457,29.4468803210327,9.50910023162778));
#7351=CARTESIAN_POINT('Ctrl Pts',(-7.83477659936034,29.4585506279031,9.32326607847403));
#7352=CARTESIAN_POINT('Ctrl Pts',(-8.06038815211785,29.4702209347736,9.1289170547268));
#7353=CARTESIAN_POINT('Ctrl Pts',(-8.27855472469357,29.4818912416441,8.92658848162353));
#7354=CARTESIAN_POINT('Ctrl Pts',(-8.49672129726929,29.4935615485146,8.72425990852026));
#7355=CARTESIAN_POINT('Ctrl Pts',(-8.70744264963627,29.5052318553851,8.51395202063495));
#7356=CARTESIAN_POINT('Ctrl Pts',(-8.91014947085614,29.5169021622556,8.29624533490916));
#7357=CARTESIAN_POINT('Ctrl Pts',(-9.10377205847044,29.5280494685027,8.08829509634546));
#7358=CARTESIAN_POINT('Ctrl Pts',(-9.29014048970121,29.5391967747498,7.87353252575311));
#7359=CARTESIAN_POINT('Ctrl Pts',(-9.46878458047568,29.550344080997,7.65248775357047));
#7360=CARTESIAN_POINT('Ctrl Pts',(-9.64739832857408,29.5614894938755,7.43148052581425));
#7361=CARTESIAN_POINT('Ctrl Pts',(-9.81829018797549,29.5726349067541,7.2041934341806));
#7362=CARTESIAN_POINT('Ctrl Pts',(-9.98103016933431,29.5837803196327,6.97118978430787));
#7363=CARTESIAN_POINT('Ctrl Pts',(-10.143752084027,29.5949244951972,6.73821200146009));
#7364=CARTESIAN_POINT('Ctrl Pts',(-10.2983237750866,29.6060686707618,6.49951914625352));
#7365=CARTESIAN_POINT('Ctrl Pts',(-10.4443578030689,29.6172128463264,6.2557046230999));
#7366=CARTESIAN_POINT('Ctrl Pts',(-10.594990739265,29.6287079746193,6.00421188529549));
#7367=CARTESIAN_POINT('Ctrl Pts',(-10.7365394011799,29.6402031029121,5.74726991837197));
#7368=CARTESIAN_POINT('Ctrl Pts',(-10.868628337183,29.651698231205,5.48555998218799));
#7369=CARTESIAN_POINT('Ctrl Pts',(-10.9966913673694,29.6628430023426,5.23182663803549));
#7370=CARTESIAN_POINT('Ctrl Pts',(-11.1158626482813,29.6739877734802,4.97361191341933));
#7371=CARTESIAN_POINT('Ctrl Pts',(-11.2258473549232,29.6851325446178,4.71156040117959));
#7372=CARTESIAN_POINT('Ctrl Pts',(-11.341018430374,29.6968028514883,4.43715175465375));
#7373=CARTESIAN_POINT('Ctrl Pts',(-11.4461155690856,29.7084731583587,4.15853605659713));
#7374=CARTESIAN_POINT('Ctrl Pts',(-11.5408569815104,29.7201434652292,3.8764765422123));
#7375=CARTESIAN_POINT('Ctrl Pts',(-11.6355983939352,29.7318137720997,3.59441702782744));
#7376=CARTESIAN_POINT('Ctrl Pts',(-11.7199839815676,29.7434840789702,3.30891401794856));
#7377=CARTESIAN_POINT('Ctrl Pts',(-11.7937916549543,29.7551543858407,3.02074968336178));
#7378=CARTESIAN_POINT('Ctrl Pts',(-11.8651552549867,29.7664382412116,2.74212764620159));
#7379=CARTESIAN_POINT('Ctrl Pts',(-11.9266493212993,29.7777220965825,2.46094394049381));
#7380=CARTESIAN_POINT('Ctrl Pts',(-11.9781123416308,29.7890059519535,2.17790610019643));
#7381=CARTESIAN_POINT('Ctrl Pts',(-12.0295653763274,29.8002876178598,1.89492317918895));
#7382=CARTESIAN_POINT('Ctrl Pts',(-12.0709912069458,29.8115692837662,1.61008709067454));
#7383=CARTESIAN_POINT('Ctrl Pts',(-12.1022795090425,29.8228509496725,1.32411515171836));
#7384=CARTESIAN_POINT('Ctrl Pts',(-12.1335625490621,29.8341307182245,1.03819130761862));
#7385=CARTESIAN_POINT('Ctrl Pts',(-12.1547114378685,29.8454104867765,0.751132245746415));
#7386=CARTESIAN_POINT('Ctrl Pts',(-12.1656676092229,29.8566902553285,0.463661376334469));
#7387=CARTESIAN_POINT('Ctrl Pts',(-12.1715549693444,29.8627515022189,0.309187292468078));
#7388=CARTESIAN_POINT('Ctrl Pts',(-12.1745000598421,29.8688127491093,0.154594386717212));
#7389=CARTESIAN_POINT('Ctrl Pts',(-12.1744999999991,29.8748739959996,-4.71256420053583E-6));
#7390=CARTESIAN_POINT('',(-12.1744999986658,29.6251260039304,0.000180241411394071));
#7391=CARTESIAN_POINT('Ctrl Pts',(1.59078448392775,28.8125580693322,12.0701224093086));
#7392=CARTESIAN_POINT('Ctrl Pts',(1.56741528365208,28.813482803771,12.0732023582884));
#7393=CARTESIAN_POINT('Ctrl Pts',(1.5440374216093,28.8144075382099,12.0762144014192));
#7394=CARTESIAN_POINT('Ctrl Pts',(1.52065129953035,28.8153322726487,12.0791584920158));
#7395=CARTESIAN_POINT('Ctrl Pts',(1.2387408895783,28.8264795788958,12.114648334419));
#7396=CARTESIAN_POINT('Ctrl Pts',(0.955545409716462,28.8376268851429,12.1402700844111));
#7397=CARTESIAN_POINT('Ctrl Pts',(0.671769844144576,28.84877419139,12.1559522673667));
#7398=CARTESIAN_POINT('Ctrl Pts',(0.388042477816675,28.8599196042686,12.1716317867055));
#7399=CARTESIAN_POINT('Ctrl Pts',(0.103735488728669,28.8710650171472,12.1773750948538));
#7400=CARTESIAN_POINT('Ctrl Pts',(-0.180442727021527,28.8822104300257,12.1731627226561));
#7401=CARTESIAN_POINT('Ctrl Pts',(-0.464589394575869,28.8933546055903,12.1689508180973));
#7402=CARTESIAN_POINT('Ctrl Pts',(-0.748607050689398,28.9044987811549,12.154785444124));
#7403=CARTESIAN_POINT('Ctrl Pts',(-1.03178776018544,28.9156429567196,12.1306992489276));
#7404=CARTESIAN_POINT('Ctrl Pts',(-1.32388640551311,28.9271380850124,12.1058545305126));
#7405=CARTESIAN_POINT('Ctrl Pts',(-1.61509423925263,28.9386332133053,12.0704540273365));
#7406=CARTESIAN_POINT('Ctrl Pts',(-1.90463906235076,28.9501283415981,12.0245914813006));
#7407=CARTESIAN_POINT('Ctrl Pts',(-2.18535892082461,28.9612731127357,11.9801267683947));
#7408=CARTESIAN_POINT('Ctrl Pts',(-2.46451536486885,28.9724178838733,11.9258283526591));
#7409=CARTESIAN_POINT('Ctrl Pts',(-2.74141308360023,28.9835626550109,11.8618339456876));
#7410=CARTESIAN_POINT('Ctrl Pts',(-3.03136801487957,28.9952329618814,11.7948218592005));
#7411=CARTESIAN_POINT('Ctrl Pts',(-3.31884576343318,29.0069032687519,11.717177414097));
#7412=CARTESIAN_POINT('Ctrl Pts',(-3.60306239103951,29.0185735756224,11.6291182665014));
#7413=CARTESIAN_POINT('Ctrl Pts',(-3.88727901864584,29.0302438824928,11.5410591189058));
#7414=CARTESIAN_POINT('Ctrl Pts',(-4.16823420743134,29.0419141893633,11.442585376495));
#7415=CARTESIAN_POINT('Ctrl Pts',(-4.44516356389173,29.0535844962338,11.3339741988523));
#7416=CARTESIAN_POINT('Ctrl Pts',(-4.70968243040855,29.0647318024809,11.2302303922428));
#7417=CARTESIAN_POINT('Ctrl Pts',(-4.97060736729662,29.075879108728,11.117206805338));
#7418=CARTESIAN_POINT('Ctrl Pts',(-5.22728514945102,29.0870264149751,10.9951780438667));
#7419=CARTESIAN_POINT('Ctrl Pts',(-5.48391933491689,29.0981718278537,10.873170008965));
#7420=CARTESIAN_POINT('Ctrl Pts',(-5.73630756506488,29.1093172407323,10.7421599676865));
#7421=CARTESIAN_POINT('Ctrl Pts',(-5.98381850576247,29.1204626536109,10.6024698226448));
#7422=CARTESIAN_POINT('Ctrl Pts',(-6.2313019689003,29.1316068291754,10.4627951853795));
#7423=CARTESIAN_POINT('Ctrl Pts',(-6.47390899154312,29.14275100474,10.3144424996335));
#7424=CARTESIAN_POINT('Ctrl Pts',(-6.71103358465277,29.1538951803046,10.1577792098304));
#7425=CARTESIAN_POINT('Ctrl Pts',(-6.95562571292541,29.1653903085975,9.99618227476502));
#7426=CARTESIAN_POINT('Ctrl Pts',(-7.19438425759036,29.1768854368903,9.82574297352866));
#7427=CARTESIAN_POINT('Ctrl Pts',(-7.42667603774404,29.1883805651832,9.64691314775864));
#7428=CARTESIAN_POINT('Ctrl Pts',(-7.65188785452438,29.1995253363208,9.47353383175558));
#7429=CARTESIAN_POINT('Ctrl Pts',(-7.87102104620591,29.2106701074584,9.29226805311522));
#7430=CARTESIAN_POINT('Ctrl Pts',(-8.08353098601621,29.221814878596,9.10356946741858));
#7431=CARTESIAN_POINT('Ctrl Pts',(-8.30606190926227,29.2334851854665,8.90597273134222));
#7432=CARTESIAN_POINT('Ctrl Pts',(-8.52132966920872,29.245155492337,8.70022553865971));
#7433=CARTESIAN_POINT('Ctrl Pts',(-8.7287500754548,29.2568257992075,8.4868941533548));
#7434=CARTESIAN_POINT('Ctrl Pts',(-8.93617048170086,29.2684961060779,8.27356276804991));
#7435=CARTESIAN_POINT('Ctrl Pts',(-9.13574330666112,29.2801664129484,8.05264743678594));
#7436=CARTESIAN_POINT('Ctrl Pts',(-9.32692999639901,29.2918367198189,7.82475731842672));
#7437=CARTESIAN_POINT('Ctrl Pts',(-9.50954872309849,29.302984026066,7.6070800141164));
#7438=CARTESIAN_POINT('Ctrl Pts',(-9.68457097741769,29.3141313323131,7.38297431499236));
#7439=CARTESIAN_POINT('Ctrl Pts',(-9.85155459629223,29.3252786385603,7.1529939386437));
#7440=CARTESIAN_POINT('Ctrl Pts',(-10.0185098530204,29.3364240514388,6.9230526244327));
#7441=CARTESIAN_POINT('Ctrl Pts',(-10.1774290435821,29.3475694643174,6.68723884089972));
#7442=CARTESIAN_POINT('Ctrl Pts',(-10.3279118601732,29.358714877196,6.44613735957391));
#7443=CARTESIAN_POINT('Ctrl Pts',(-10.4783779708334,29.3698590527605,6.20506264425865));
#7444=CARTESIAN_POINT('Ctrl Pts',(-10.6204094365009,29.3810032283251,5.95870162955929));
#7445=CARTESIAN_POINT('Ctrl Pts',(-10.753649997694,29.3921474038897,5.70766694693163));
#7446=CARTESIAN_POINT('Ctrl Pts',(-10.8910865748418,29.4036425321825,5.44872667216268));
#7447=CARTESIAN_POINT('Ctrl Pts',(-11.019169440786,29.4151376604754,5.18481385036724));
#7448=CARTESIAN_POINT('Ctrl Pts',(-11.1375588475103,29.4266327887682,4.91662823164873));
#7449=CARTESIAN_POINT('Ctrl Pts',(-11.2523398929623,29.4377775599059,4.6566165756786));
#7450=CARTESIAN_POINT('Ctrl Pts',(-11.3580095056908,29.4489223310435,4.39258898024842));
#7451=CARTESIAN_POINT('Ctrl Pts',(-11.4543065619484,29.4600671021811,4.12520441128752));
#7452=CARTESIAN_POINT('Ctrl Pts',(-11.5551445408871,29.4717374090516,3.84521122581278));
#7453=CARTESIAN_POINT('Ctrl Pts',(-11.6457046540313,29.483407715922,3.56153714931589));
#7454=CARTESIAN_POINT('Ctrl Pts',(-11.7257449261543,29.4950780227925,3.274958958028));
#7455=CARTESIAN_POINT('Ctrl Pts',(-11.8057851982772,29.506748329663,2.98838076674009));
#7456=CARTESIAN_POINT('Ctrl Pts',(-11.8753055475832,29.5184186365335,2.69889878615673));
#7457=CARTESIAN_POINT('Ctrl Pts',(-11.9341245976263,29.530088943404,2.4073056179742));
#7458=CARTESIAN_POINT('Ctrl Pts',(-11.9917048891097,29.5415134677853,2.12185354749385));
#7459=CARTESIAN_POINT('Ctrl Pts',(-12.0390440781821,29.5529379921666,1.83431123741328));
#7460=CARTESIAN_POINT('Ctrl Pts',(-12.0760155945832,29.5643625165479,1.54541179281881));
#7461=CARTESIAN_POINT('Ctrl Pts',(-12.1129779697708,29.5757842162137,1.25658377865915));
#7462=CARTESIAN_POINT('Ctrl Pts',(-12.1395777632545,29.5872059158794,0.966399535564798));
#7463=CARTESIAN_POINT('Ctrl Pts',(-12.1557400447632,29.5986276155452,0.675599151968931));
#7464=CARTESIAN_POINT('Ctrl Pts',(-12.168238897098,29.6074604116736,0.450713138721019));
#7465=CARTESIAN_POINT('Ctrl Pts',(-12.1744966634544,29.616293207802,0.225458828196562));
#7466=CARTESIAN_POINT('Ctrl Pts',(-12.1744999986658,29.6251260039304,0.000180241411402181));
#7467=CARTESIAN_POINT('Ctrl Pts',(-12.1744999986658,29.6251260039651,0.00018024052605028));
#7468=CARTESIAN_POINT('Ctrl Pts',(-12.1745042222142,29.6363114795878,-0.285102936417017));
#7469=CARTESIAN_POINT('Ctrl Pts',(-12.1644766085762,29.6474969552104,-0.570385273907491));
#7470=CARTESIAN_POINT('Ctrl Pts',(-12.1444433863984,29.6586824308331,-0.854953264549404));
#7471=CARTESIAN_POINT('Ctrl Pts',(-12.1244071877467,29.6698695683589,-1.13956353541974));
#7472=CARTESIAN_POINT('Ctrl Pts',(-12.0943624266308,29.6810567058848,-1.42345898533909));
#7473=CARTESIAN_POINT('Ctrl Pts',(-12.0543873318725,29.6922438434107,-1.70592974743708));
#7474=CARTESIAN_POINT('Ctrl Pts',(-12.0144104223308,29.7034314888086,-1.98841333310159));
#7475=CARTESIAN_POINT('Ctrl Pts',(-11.9645023183561,29.7146191342066,-2.2694718422521));
#7476=CARTESIAN_POINT('Ctrl Pts',(-11.9047927944751,29.7258067796045,-2.54840318054546));
#7477=CARTESIAN_POINT('Ctrl Pts',(-11.8450710809749,29.7369967089452,-2.8273914622972));
#7478=CARTESIAN_POINT('Ctrl Pts',(-11.7755440050082,29.7481866382859,-3.10425144891475));
#7479=CARTESIAN_POINT('Ctrl Pts',(-11.6963922226106,29.7593765676266,-3.37829235337227));
#7480=CARTESIAN_POINT('Ctrl Pts',(-11.6752552402276,29.7623647674141,-3.4514732419674));
#7481=CARTESIAN_POINT('Ctrl Pts',(-11.6534321750649,29.7653529672017,-3.52445317187036));
#7482=CARTESIAN_POINT('Ctrl Pts',(-11.6309270707671,29.7683411669892,-3.59721916547995));
#7483=CARTESIAN_POINT('Ctrl Pts',(-11.5469730825569,29.7794884732363,-3.86866849043174));
#7484=CARTESIAN_POINT('Ctrl Pts',(-11.4534995431357,29.7906357794834,-4.13721802276228));
#7485=CARTESIAN_POINT('Ctrl Pts',(-11.3507321374569,29.8017830857305,-4.40219606488654));
#7486=CARTESIAN_POINT('Ctrl Pts',(-11.247982186809,29.8129284986091,-4.66712910052394));
#7487=CARTESIAN_POINT('Ctrl Pts',(-11.1359416179192,29.8240739114877,-4.92849160846213));
#7488=CARTESIAN_POINT('Ctrl Pts',(-11.0148848982189,29.8352193243662,-5.18563023450271));
#7489=CARTESIAN_POINT('Ctrl Pts',(-10.8938416176952,29.8463634999308,-5.44274031416114));
#7490=CARTESIAN_POINT('Ctrl Pts',(-10.7637842986543,29.8575076754954,-5.69562720699591));
#7491=CARTESIAN_POINT('Ctrl Pts',(-10.6250346954393,29.86865185106,-5.94365947634216));
#7492=CARTESIAN_POINT('Ctrl Pts',(-10.4819155853449,29.8801469793528,-6.19950278573525));
#7493=CARTESIAN_POINT('Ctrl Pts',(-10.329547980573,29.8916421076457,-6.45018048931594));
#7494=CARTESIAN_POINT('Ctrl Pts',(-10.1683357975651,29.9031372359385,-6.69502780860221));
#7495=CARTESIAN_POINT('Ctrl Pts',(-10.0120371605734,29.9142820070761,-6.93241248736197));
#7496=CARTESIAN_POINT('Ctrl Pts',(-9.84742525859584,29.9254267782137,-7.16431669157156));
#7497=CARTESIAN_POINT('Ctrl Pts',(-9.67491234763068,29.9365715493513,-7.39016382197738));
#7498=CARTESIAN_POINT('Ctrl Pts',(-9.49426452765975,29.9482418562218,-7.62666085588776));
#7499=CARTESIAN_POINT('Ctrl Pts',(-9.30495281210028,29.9599121630923,-7.85651557113396));
#7500=CARTESIAN_POINT('Ctrl Pts',(-9.10749884104637,29.9715824699628,-8.07910360809534));
#7501=CARTESIAN_POINT('Ctrl Pts',(-8.91004486999248,29.9832527768333,-8.30169164505669));
#7502=CARTESIAN_POINT('Ctrl Pts',(-8.70444887265217,29.9949230837037,-8.51701275857697));
#7503=CARTESIAN_POINT('Ctrl Pts',(-8.49127863272491,30.0065933905742,-8.7244849378877));
#7504=CARTESIAN_POINT('Ctrl Pts',(-8.28766154076552,30.0177406968213,-8.92265932577667));
#7505=CARTESIAN_POINT('Ctrl Pts',(-8.07707334551595,30.0288880030684,-9.11373199757563));
#7506=CARTESIAN_POINT('Ctrl Pts',(-7.86003364885051,30.0400353093155,-9.29722115951523));
#7507=CARTESIAN_POINT('Ctrl Pts',(-7.64303081634977,30.0511807221941,-9.48067915584417));
#7508=CARTESIAN_POINT('Ctrl Pts',(-7.41957887379889,30.0623261350727,-9.656556041771));
#7509=CARTESIAN_POINT('Ctrl Pts',(-7.19023147912979,30.0734715479513,-9.82440947469776));
#7510=CARTESIAN_POINT('Ctrl Pts',(-6.96090954558389,30.0846157235159,-9.99224427328623));
#7511=CARTESIAN_POINT('Ctrl Pts',(-6.72569368202658,30.0957598990805,-10.1520572400168));
#7512=CARTESIAN_POINT('Ctrl Pts',(-6.48516857886181,30.1069040746452,-10.3034479061013));
#7513=CARTESIAN_POINT('Ctrl Pts',(-6.2370688515653,30.118399202938,-10.4596061718149));
#7514=CARTESIAN_POINT('Ctrl Pts',(-5.98332031440759,30.1298943312309,-10.6068029039343));
#7515=CARTESIAN_POINT('Ctrl Pts',(-5.72459575688008,30.1413894595237,-10.7446476754853));
#7516=CARTESIAN_POINT('Ctrl Pts',(-5.47375680077022,30.1525342306613,-10.8782911105402));
#7517=CARTESIAN_POINT('Ctrl Pts',(-5.21824090472264,30.1636790017989,-11.0031440843534));
#7518=CARTESIAN_POINT('Ctrl Pts',(-4.95868598336946,30.1748237729366,-11.1188975878158));
#7519=CARTESIAN_POINT('Ctrl Pts',(-4.68689165538149,30.186494079807,-11.240109489797));
#7520=CARTESIAN_POINT('Ctrl Pts',(-4.4106685032706,30.1981643866775,-11.3513429650037));
#7521=CARTESIAN_POINT('Ctrl Pts',(-4.13077334331136,30.2098346935479,-11.4522994126153));
#7522=CARTESIAN_POINT('Ctrl Pts',(-3.85087818335214,30.2215050004184,-11.5532558602268));
#7523=CARTESIAN_POINT('Ctrl Pts',(-3.56731133412171,30.2331753072889,-11.643935174666));
#7524=CARTESIAN_POINT('Ctrl Pts',(-3.28084986321212,30.2448456141593,-11.7240980218122));
#7525=CARTESIAN_POINT('Ctrl Pts',(-3.00722606054148,30.2559929204064,-11.8006683996693));
#7526=CARTESIAN_POINT('Ctrl Pts',(-2.730879655486,30.2671402266535,-11.8676670436835));
#7527=CARTESIAN_POINT('Ctrl Pts',(-2.4524974507845,30.2782875329007,-11.9249195596405));
#7528=CARTESIAN_POINT('Ctrl Pts',(-2.1741625292645,30.2894329457793,-11.982162351265));
#7529=CARTESIAN_POINT('Ctrl Pts',(-1.89379275962855,30.3005783586578,-12.0296622660807));
#7530=CARTESIAN_POINT('Ctrl Pts',(-1.61208596895292,30.3117237715364,-12.0672958478155));
#7531=CARTESIAN_POINT('Ctrl Pts',(-1.33041045210901,30.322867947101,-12.1049252516379));
#7532=CARTESIAN_POINT('Ctrl Pts',(-1.04739847494732,30.3340121226655,-12.1326904742397));
#7533=CARTESIAN_POINT('Ctrl Pts',(-0.76375507464333,30.3451562982301,-12.1505196776087));
#7534=CARTESIAN_POINT('Ctrl Pts',(-0.471179167432266,30.3566514265229,-12.1689103588125));
#7535=CARTESIAN_POINT('Ctrl Pts',(-0.177931718560721,30.3681465548158,-12.1767290407253));
#7536=CARTESIAN_POINT('Ctrl Pts',(0.11520968357079,30.3796416831087,-12.1739548618685));
#7537=CARTESIAN_POINT('Ctrl Pts',(0.399416501840013,30.3907864542463,-12.1712652365189));
#7538=CARTESIAN_POINT('Ctrl Pts',(0.683523362930164,30.4019312253839,-12.1586189056607));
#7539=CARTESIAN_POINT('Ctrl Pts',(0.966822262734164,30.4130759965215,-12.136049808825));
#7540=CARTESIAN_POINT('Ctrl Pts',(1.26348022510641,30.4247463033919,-12.1124164580266));
#7541=CARTESIAN_POINT('Ctrl Pts',(1.55925187642808,30.4364166102624,-12.0779020256309));
#7542=CARTESIAN_POINT('Ctrl Pts',(1.85332979011732,30.4480869171329,-12.0326064898285));
#7543=CARTESIAN_POINT('Ctrl Pts',(2.14740770380658,30.4597572240034,-11.9873109540262));
#7544=CARTESIAN_POINT('Ctrl Pts',(2.43979154960908,30.4714275308739,-11.9312343745664));
#7545=CARTESIAN_POINT('Ctrl Pts',(2.72968448063129,30.4830978377444,-11.8645384607325));
#7546=CARTESIAN_POINT('Ctrl Pts',(3.00658596375755,30.4942451439915,-11.8008315003939));
#7547=CARTESIAN_POINT('Ctrl Pts',(3.28129758340433,30.5053924502386,-11.7274170609569));
#7548=CARTESIAN_POINT('Ctrl Pts',(3.55313282753996,30.5165397564857,-11.6444706775301));
#7549=CARTESIAN_POINT('Ctrl Pts',(3.8249219004943,30.5276851693643,-11.5615383825358));
#7550=CARTESIAN_POINT('Ctrl Pts',(4.09383531829407,30.5388305822429,-11.4690774537046));
#7551=CARTESIAN_POINT('Ctrl Pts',(4.35920126481122,30.5499759951215,-11.3673134285489));
#7552=CARTESIAN_POINT('Ctrl Pts',(4.62453775158353,30.561120170686,-11.2655607007818));
#7553=CARTESIAN_POINT('Ctrl Pts',(4.8863273044804,30.5722643462505,-11.1545070344914));
#7554=CARTESIAN_POINT('Ctrl Pts',(5.14391647798478,30.583408521815,-11.0344267416806));
#7555=CARTESIAN_POINT('Ctrl Pts',(5.40961765786553,30.5949036501079,-10.9105648765014));
#7556=CARTESIAN_POINT('Ctrl Pts',(5.67084934137553,30.6063987784008,-10.7770987550051));
#7557=CARTESIAN_POINT('Ctrl Pts',(5.92691877280664,30.6178939066936,-10.6343821687276));
#7558=CARTESIAN_POINT('Ctrl Pts',(6.17518352774736,30.6290386778313,-10.4960154057753));
#7559=CARTESIAN_POINT('Ctrl Pts',(6.41859580509325,30.6401834489689,-10.3489538491387));
#7560=CARTESIAN_POINT('Ctrl Pts',(6.65655017324196,30.6513282201065,-10.1935661101065));
#7561=CARTESIAN_POINT('Ctrl Pts',(6.90572536609043,30.662998526977,-10.0308510057743));
#7562=CARTESIAN_POINT('Ctrl Pts',(7.14891525866527,30.6746688338475,-9.85900575003922));
#7563=CARTESIAN_POINT('Ctrl Pts',(7.38545872235907,30.686339140718,-9.67850451827814));
#7564=CARTESIAN_POINT('Ctrl Pts',(7.62200218605287,30.6980094475885,-9.49800328651705));
#7565=CARTESIAN_POINT('Ctrl Pts',(7.85189895947368,30.709679754459,-9.30884628923451));
#7566=CARTESIAN_POINT('Ctrl Pts',(8.07452674462437,30.7213500613295,-9.11155684284227));
#7567=CARTESIAN_POINT('Ctrl Pts',(8.28717754530411,30.7324973675766,-8.92310885234291));
#7568=CARTESIAN_POINT('Ctrl Pts',(8.49326006179604,30.7436446738237,-8.72718501437767));
#7569=CARTESIAN_POINT('Ctrl Pts',(8.69225549345207,30.7547919800708,-8.5242679853787));
#7570=CARTESIAN_POINT('Ctrl Pts',(8.89121712575945,30.7659373929494,-8.32138542181121));
#7571=CARTESIAN_POINT('Ctrl Pts',(9.08309388979978,30.7770828058279,-8.11151222901553));
#7572=CARTESIAN_POINT('Ctrl Pts',(9.26740381715853,30.7882282187065,-7.89516793613129));
#7573=CARTESIAN_POINT('Ctrl Pts',(9.45169328325129,30.799372394271,-7.67884766082539));
#7574=CARTESIAN_POINT('Ctrl Pts',(9.62841741714045,30.8105165698356,-7.45605792294662));
#7575=CARTESIAN_POINT('Ctrl Pts',(9.79713372166527,30.8216607454001,-7.22735228765066));
#7576=CARTESIAN_POINT('Ctrl Pts',(9.97116324537299,30.833155873693,-6.99144424727527));
#7577=CARTESIAN_POINT('Ctrl Pts',(10.1366722171862,30.8446510019859,-6.74924189735682));
#7578=CARTESIAN_POINT('Ctrl Pts',(10.2932216574201,30.8561461302788,-6.50138740279476));
#7579=CARTESIAN_POINT('Ctrl Pts',(10.4449996662147,30.8672909014164,-6.26108720370593));
#7580=CARTESIAN_POINT('Ctrl Pts',(10.5883560576881,30.878435672554,-6.0154745345967));
#7581=CARTESIAN_POINT('Ctrl Pts',(10.7229356202183,30.8895804436917,-5.76516278474886));
#7582=CARTESIAN_POINT('Ctrl Pts',(10.863861330924,30.9012507505621,-5.50304749337706));
#7583=CARTESIAN_POINT('Ctrl Pts',(10.9951623959182,30.9129210574326,-5.23577956394943));
#7584=CARTESIAN_POINT('Ctrl Pts',(11.1164852149522,30.9245913643031,-4.96409173119816));
#7585=CARTESIAN_POINT('Ctrl Pts',(11.2378080339862,30.9362616711736,-4.69240389844691));
#7586=CARTESIAN_POINT('Ctrl Pts',(11.3491524782764,30.9479319780441,-4.41629647229572));
#7587=CARTESIAN_POINT('Ctrl Pts',(11.4502225594297,30.9596022849146,-4.13652675435896));
#7588=CARTESIAN_POINT('Ctrl Pts',(11.5467632210884,30.9707495911617,-3.86929481614853));
#7589=CARTESIAN_POINT('Ctrl Pts',(11.6339589947617,30.9818968974088,-3.59864180777725));
#7590=CARTESIAN_POINT('Ctrl Pts',(11.7115853118451,30.993044203656,-3.32523980088261));
#7591=CARTESIAN_POINT('Ctrl Pts',(11.7891984441082,31.0041896165345,-3.05188423128495));
#7592=CARTESIAN_POINT('Ctrl Pts',(11.8572452920049,31.015335029413,-2.77578085187103));
#7593=CARTESIAN_POINT('Ctrl Pts',(11.9155512731645,31.0264804422916,-2.49761648508908));
#7594=CARTESIAN_POINT('Ctrl Pts',(11.9738507814546,31.0376246178562,-2.21948299887197));
#7595=CARTESIAN_POINT('Ctrl Pts',(12.022411527657,31.0487687934208,-1.9392892431739));
#7596=CARTESIAN_POINT('Ctrl Pts',(12.0611098753863,31.0599129689854,-1.65773303757252));
#7597=CARTESIAN_POINT('Ctrl Pts',(12.1010269127024,31.0714080972782,-1.36731005506706));
#7598=CARTESIAN_POINT('Ctrl Pts',(12.1304502618443,31.0829032255711,-1.07543771211255));
#7599=CARTESIAN_POINT('Ctrl Pts',(12.1493017737572,31.094398353864,-0.782889941294685));
#7600=CARTESIAN_POINT('Ctrl Pts',(12.1675787151288,31.1055431250016,-0.499258661197821));
#7601=CARTESIAN_POINT('Ctrl Pts',(12.17591869138,31.1166878961392,-0.214992794448297));
#7602=CARTESIAN_POINT('Ctrl Pts',(12.1743033368384,31.1278326672768,0.069199079805505));
#7603=CARTESIAN_POINT('Ctrl Pts',(12.1726118096663,31.1395029741473,0.366792125161997));
#7604=CARTESIAN_POINT('Ctrl Pts',(12.1600034675358,31.1511732810177,0.664303713974559));
#7605=CARTESIAN_POINT('Ctrl Pts',(12.136518471558,31.1628435878882,0.960921245228644));
#7606=CARTESIAN_POINT('Ctrl Pts',(12.1130334755802,31.1745138947587,1.25753877648276));
#7607=CARTESIAN_POINT('Ctrl Pts',(12.0786718609865,31.1861842016292,1.55326191641704));
#7608=CARTESIAN_POINT('Ctrl Pts',(12.0335361321028,31.1978545084997,1.84728406244831));
#7609=CARTESIAN_POINT('Ctrl Pts',(11.9904231447464,31.2090018147468,2.12812971129163));
#7610=CARTESIAN_POINT('Ctrl Pts',(11.9374676168789,31.2201491209939,2.40750735169076));
#7611=CARTESIAN_POINT('Ctrl Pts',(11.8747939778081,31.231296427241,2.68471939587967));
#7612=CARTESIAN_POINT('Ctrl Pts',(11.8121309838468,31.2424418401196,2.96188435563876));
#7613=CARTESIAN_POINT('Ctrl Pts',(11.7397532329452,31.2535872529982,3.2368841934707));
#7614=CARTESIAN_POINT('Ctrl Pts',(11.6578361044304,31.2647326658768,3.50903228999679));
#7615=CARTESIAN_POINT('Ctrl Pts',(11.5759280699893,31.2758768414414,3.7811501738566));
#7616=CARTESIAN_POINT('Ctrl Pts',(11.4844828494922,31.287021017006,4.0504166932242));
#7617=CARTESIAN_POINT('Ctrl Pts',(11.383725818712,31.2981651925706,4.31615995236384));
#7618=CARTESIAN_POINT('Ctrl Pts',(11.2797957443419,31.3096603208635,4.59027200659853));
#7619=CARTESIAN_POINT('Ctrl Pts',(11.1659579563437,31.3211554491563,4.8606350145712));
#7620=CARTESIAN_POINT('Ctrl Pts',(11.0425141946155,31.3326505774492,5.12653201606268));
#7621=CARTESIAN_POINT('Ctrl Pts',(10.922832844588,31.3437953485868,5.38432480900107));
#7622=CARTESIAN_POINT('Ctrl Pts',(10.7941225236154,31.3549401197244,5.63791954766483));
#7623=CARTESIAN_POINT('Ctrl Pts',(10.6567061908373,31.366084890862,5.88668526525489));
#7624=CARTESIAN_POINT('Ctrl Pts',(10.5128099409518,31.3777551977325,6.14718162065625));
#7625=CARTESIAN_POINT('Ctrl Pts',(10.3593670062242,31.3894255046029,6.40238228983842));
#7626=CARTESIAN_POINT('Ctrl Pts',(10.1968015149776,31.4010958114734,6.65159297568257));
#7627=CARTESIAN_POINT('Ctrl Pts',(10.0342360237311,31.4127661183439,6.90080366152668));
#7628=CARTESIAN_POINT('Ctrl Pts',(9.86254816662018,31.4244364252143,7.14402408782862));
#7629=CARTESIAN_POINT('Ctrl Pts',(9.68221394281234,31.4361067320848,7.38059505836828));
#7630=CARTESIAN_POINT('Ctrl Pts',(9.50996133266801,31.4472540383319,7.60656418557765));
#7631=CARTESIAN_POINT('Ctrl Pts',(9.32976884399584,31.4584013445791,7.82653423106822));
#7632=CARTESIAN_POINT('Ctrl Pts',(9.1420795592616,31.4695486508262,8.0399522126771));
#7633=CARTESIAN_POINT('Ctrl Pts',(8.95442215352886,31.4806940637047,8.25333394526852));
#7634=CARTESIAN_POINT('Ctrl Pts',(8.75927067002798,31.4918394765833,8.4601656355874));
#7635=CARTESIAN_POINT('Ctrl Pts',(8.557107679775,31.5029848894619,8.65992831417996));
#7636=CARTESIAN_POINT('Ctrl Pts',(8.35496713275467,31.5141290650264,8.85966881601174));
#7637=CARTESIAN_POINT('Ctrl Pts',(8.14581682298889,31.525273240591,9.05234168573748));
#7638=CARTESIAN_POINT('Ctrl Pts',(7.93017617569519,31.5364174161556,9.23746480764265));
#7639=CARTESIAN_POINT('Ctrl Pts',(7.70774456633725,31.5479125444485,9.42841783274024));
#7640=CARTESIAN_POINT('Ctrl Pts',(7.47840742626827,31.5594076727413,9.61133769016819));
#7641=CARTESIAN_POINT('Ctrl Pts',(7.24277279859588,31.5709028010342,9.78573923819348));
#7642=CARTESIAN_POINT('Ctrl Pts',(7.01432002011553,31.5820475721717,9.95482524482681));
#7643=CARTESIAN_POINT('Ctrl Pts',(6.7799481729941,31.5931923433093,10.1159043417915));
#7644=CARTESIAN_POINT('Ctrl Pts',(6.54024278067394,31.6043371144468,10.2685770494184));
#7645=CARTESIAN_POINT('Ctrl Pts',(6.28923399347095,31.6160074213174,10.4284490940541));
#7646=CARTESIAN_POINT('Ctrl Pts',(6.03237681530382,31.6276777281879,10.5791026894094));
#7647=CARTESIAN_POINT('Ctrl Pts',(5.77037590892342,31.6393480350584,10.7201311614978));
#7648=CARTESIAN_POINT('Ctrl Pts',(5.50837500254302,31.6510183419289,10.8611596335862));
#7649=CARTESIAN_POINT('Ctrl Pts',(5.24123066753183,31.6626886487994,10.9925628311192));
#7650=CARTESIAN_POINT('Ctrl Pts',(4.96967631529749,31.6743589556699,11.1139897233699));
#7651=CARTESIAN_POINT('Ctrl Pts',(4.70170325855833,31.6858753529563,11.2338152213559));
#7652=CARTESIAN_POINT('Ctrl Pts',(4.429353113389,31.6973917502427,11.3439629082076));
#7653=CARTESIAN_POINT('Ctrl Pts',(4.15334703314022,31.708908147529,11.4441320628655));
#7654=CARTESIAN_POINT('Ctrl Pts',(3.88623292576372,31.7200535258431,11.5410741096094));
#7655=CARTESIAN_POINT('Ctrl Pts',(3.61569501806569,31.7311989041571,11.628670387502));
#7656=CARTESIAN_POINT('Ctrl Pts',(3.34240593741423,31.7423442824711,11.7066977751857));
#7657=CARTESIAN_POINT('Ctrl Pts',(3.0554705590327,31.7540461892436,11.7886213484063));
#7658=CARTESIAN_POINT('Ctrl Pts',(2.76550256063917,31.7657480960162,11.8599959936606));
#7659=CARTESIAN_POINT('Ctrl Pts',(2.47329796532737,31.7774500027887,11.9206227783916));
#7660=CARTESIAN_POINT('Ctrl Pts',(2.18109337001554,31.7891519095613,11.9812495631225));
#7661=CARTESIAN_POINT('Ctrl Pts',(1.88665251084213,31.8008538163338,12.0311284164936));
#7662=CARTESIAN_POINT('Ctrl Pts',(1.59078448392773,31.8125557231064,12.0701224093086));
#7663=CARTESIAN_POINT('Origin',(0.,13.3748739960349,0.));
#7664=CARTESIAN_POINT('',(1.59078448392775,35.0623145891265,12.0701224093086));
#7665=CARTESIAN_POINT('',(1.59078448392778,34.8125669141531,12.0701224093086));
#7666=CARTESIAN_POINT('',(1.59078448392774,13.3748739960349,12.0701224093086));
#7667=CARTESIAN_POINT('',(-12.1744999985554,32.8748739960349,0.000187550598588881));
#7668=CARTESIAN_POINT('Ctrl Pts',(-12.1744999985554,32.8748739960349,0.000187550598588881));
#7669=CARTESIAN_POINT('Ctrl Pts',(-12.1745043615588,32.8859843814439,-0.283028740965722));
#7670=CARTESIAN_POINT('Ctrl Pts',(-12.1646216592697,32.8970947668528,-0.566289459754149));
#7671=CARTESIAN_POINT('Ctrl Pts',(-12.1448686657604,32.9082051522618,-0.848890653400877));
#7672=CARTESIAN_POINT('Ctrl Pts',(-12.125118898305,32.9193137231254,-1.13144569269124));
#7673=CARTESIAN_POINT('Ctrl Pts',(-12.0955020767017,32.930422293989,-1.4133411523803));
#7674=CARTESIAN_POINT('Ctrl Pts',(-12.0560869992745,32.9415308648526,-1.69387618081272));
#7675=CARTESIAN_POINT('Ctrl Pts',(-12.0166757019596,32.9526383703461,-1.97438430446705));
#7676=CARTESIAN_POINT('Ctrl Pts',(-11.9674680629165,32.9637458758396,-2.2535319898437));
#7677=CARTESIAN_POINT('Ctrl Pts',(-11.9085845275246,32.9748533813331,-2.5306253774118));
#7678=CARTESIAN_POINT('Ctrl Pts',(-11.849696245945,32.9859617821245,-2.80774109952985));
#7679=CARTESIAN_POINT('Ctrl Pts',(-11.7811305632598,32.9970701829159,-3.08280192803896));
#7680=CARTESIAN_POINT('Ctrl Pts',(-11.703058959395,33.0081785837073,-3.35512462405274));
#7681=CARTESIAN_POINT('Ctrl Pts',(-11.6249866141567,33.0192870899849,-3.62744990606199));
#7682=CARTESIAN_POINT('Ctrl Pts',(-11.5374082443903,33.0303955962625,-3.89703674452342));
#7683=CARTESIAN_POINT('Ctrl Pts',(-11.4405453455313,33.0415041025401,-4.16321659859816));
#7684=CARTESIAN_POINT('Ctrl Pts',(-11.3436617578851,33.0526149814652,-4.4294533055898));
#7685=CARTESIAN_POINT('Ctrl Pts',(-11.2374897710976,33.0637258603903,-4.6922813200952));
#7686=CARTESIAN_POINT('Ctrl Pts',(-11.1222997533272,33.0748367393155,-4.95105023678181));
#7687=CARTESIAN_POINT('Ctrl Pts',(-11.067529982669,33.0801196648877,-5.07408793132099));
#7688=CARTESIAN_POINT('Ctrl Pts',(-11.0107221639337,33.0854025904599,-5.19620826044135));
#7689=CARTESIAN_POINT('Ctrl Pts',(-10.9519091180938,33.0906855160321,-5.31734303191104));
#7690=CARTESIAN_POINT('Ctrl Pts',(-10.8278098809659,33.1018328222794,-5.5729450418798));
#7691=CARTESIAN_POINT('Ctrl Pts',(-10.6947401199187,33.1129801285267,-5.82423887901939));
#7692=CARTESIAN_POINT('Ctrl Pts',(-10.5530246517763,33.124127434774,-6.07059477720272));
#7693=CARTESIAN_POINT('Ctrl Pts',(-10.4113332539878,33.1352728476528,-6.31690883186865));
#7694=CARTESIAN_POINT('Ctrl Pts',(-10.2609992138668,33.1464182605315,-6.55828639092668));
#7695=CARTESIAN_POINT('Ctrl Pts',(-10.1023927896335,33.1575636734103,-6.7941232086239));
#7696=CARTESIAN_POINT('Ctrl Pts',(-9.94380397317836,33.168707848975,-7.02993384476881));
#7697=CARTESIAN_POINT('Ctrl Pts',(-9.77694475525955,33.1798520245398,-7.26020474653669));
#7698=CARTESIAN_POINT('Ctrl Pts',(-9.60222881583929,33.1909962001045,-7.48436049494315));
#7699=CARTESIAN_POINT('Ctrl Pts',(-9.42201071655001,33.2024913283972,-7.71557536324092));
#7700=CARTESIAN_POINT('Ctrl Pts',(-9.2334332035449,33.21398645669,-7.94028343973844));
#7701=CARTESIAN_POINT('Ctrl Pts',(-9.03699622097056,33.2254815849827,-8.15788879258377));
#7702=CARTESIAN_POINT('Ctrl Pts',(-8.84654639230963,33.2366263561204,-8.36886180602542));
#7703=CARTESIAN_POINT('Ctrl Pts',(-8.64870928031278,33.2477711272582,-8.57315844163609));
#7704=CARTESIAN_POINT('Ctrl Pts',(-8.44397971682008,33.258915898396,-8.77027119261035));
#7705=CARTESIAN_POINT('Ctrl Pts',(-8.22959605637275,33.2705862052662,-8.97667886697739));
#7706=CARTESIAN_POINT('Ctrl Pts',(-8.00765450035677,33.2822565121364,-9.1752086165817));
#7707=CARTESIAN_POINT('Ctrl Pts',(-7.77876523658056,33.2939268190066,-9.36532229259441));
#7708=CARTESIAN_POINT('Ctrl Pts',(-7.54987597280433,33.3055971258768,-9.55543596860713));
#7709=CARTESIAN_POINT('Ctrl Pts',(-7.31403926496306,33.317267432747,-9.73713336341621));
#7710=CARTESIAN_POINT('Ctrl Pts',(-7.07190449795741,33.3289377396172,-9.90992517740522));
#7711=CARTESIAN_POINT('Ctrl Pts',(-6.8406209138327,33.3400850458639,-10.0749733881227));
#7712=CARTESIAN_POINT('Ctrl Pts',(-6.60352227774398,33.3512323521105,-10.2319459674008));
#7713=CARTESIAN_POINT('Ctrl Pts',(-6.36119516972689,33.3623796583572,-10.3804453788189));
#7714=CARTESIAN_POINT('Ctrl Pts',(-6.1189092209383,33.3735250712353,-10.5289195676309));
#7715=CARTESIAN_POINT('Ctrl Pts',(-5.87139680057618,33.3846704841134,-10.6689233225553));
#7716=CARTESIAN_POINT('Ctrl Pts',(-5.61927217655415,33.3958158969915,-10.8001032613491));
#7717=CARTESIAN_POINT('Ctrl Pts',(-5.36717554228243,33.4069600725556,-10.9312686371318));
#7718=CARTESIAN_POINT('Ctrl Pts',(-5.11046796335894,33.4181042481198,-11.0536120297623));
#7719=CARTESIAN_POINT('Ctrl Pts',(-4.84978803993833,33.4292484236839,-11.1668261479111));
#7720=CARTESIAN_POINT('Ctrl Pts',(-4.58089877613062,33.4407435519771,-11.2836056086468));
#7721=CARTESIAN_POINT('Ctrl Pts',(-4.30778318746436,33.4522386802703,-11.3906713514839));
#7722=CARTESIAN_POINT('Ctrl Pts',(-4.03116543587642,33.4637338085635,-11.4877393545726));
#7723=CARTESIAN_POINT('Ctrl Pts',(-3.76297864793515,33.4748785797007,-11.5818488461391));
#7724=CARTESIAN_POINT('Ctrl Pts',(-3.49150028225666,33.4860233508378,-11.6665609182723));
#7725=CARTESIAN_POINT('Ctrl Pts',(-3.2174076966831,33.497168121975,-11.7416667455402));
#7726=CARTESIAN_POINT('Ctrl Pts',(-2.9303901756055,33.5088384288462,-11.8203142153935));
#7727=CARTESIAN_POINT('Ctrl Pts',(-2.64050625979877,33.5205087357174,-11.8884275851291));
#7728=CARTESIAN_POINT('Ctrl Pts',(-2.34854926057755,33.5321790425887,-11.9458263264054));
#7729=CARTESIAN_POINT('Ctrl Pts',(-2.05659226135631,33.5438493494599,-12.0032250676818));
#7730=CARTESIAN_POINT('Ctrl Pts',(-1.7625625096131,33.5555196563311,-12.0499091243916));
#7731=CARTESIAN_POINT('Ctrl Pts',(-1.46726435779509,33.5671899632023,-12.0857596184247));
#7732=CARTESIAN_POINT('Ctrl Pts',(-1.18519988690535,33.5783372694502,-12.1200034854056));
#7733=CARTESIAN_POINT('Ctrl Pts',(-0.901893961090877,33.5894845756981,-12.1443736781868));
#7734=CARTESIAN_POINT('Ctrl Pts',(-0.618051873482272,33.600631881946,-12.1588018378328));
#7735=CARTESIAN_POINT('Ctrl Pts',(-0.334257996414995,33.6117772948253,-12.1732275468577));
#7736=CARTESIAN_POINT('Ctrl Pts',(-0.0499284056711118,33.6229227077047,
-12.1777145806061));
#7737=CARTESIAN_POINT('Ctrl Pts',(0.234228423541575,33.6340681205841,-12.1722466001805));
#7738=CARTESIAN_POINT('Ctrl Pts',(0.518353706932561,33.6452122961495,-12.1667792267857));
#7739=CARTESIAN_POINT('Ctrl Pts',(0.802306000460723,33.656356471715,-12.1513590511788));
#7740=CARTESIAN_POINT('Ctrl Pts',(1.08537752011688,33.6675006472804,-12.1260218492639));
#7741=CARTESIAN_POINT('Ctrl Pts',(1.37736353695788,33.6789957755727,-12.0998867273907));
#7742=CARTESIAN_POINT('Ctrl Pts',(1.66841210987824,33.6904909038649,-12.0631998598761));
#7743=CARTESIAN_POINT('Ctrl Pts',(1.95775146156407,33.7019860321572,-12.0160583996893));
#7744=CARTESIAN_POINT('Ctrl Pts',(2.23827211117223,33.7131308032956,-11.9703537523331));
#7745=CARTESIAN_POINT('Ctrl Pts',(2.5171859111229,33.7242755744339,-11.91482240613));
#7746=CARTESIAN_POINT('Ctrl Pts',(2.79379816580269,33.7354203455723,-11.84960514358));
#7747=CARTESIAN_POINT('Ctrl Pts',(3.08345417181668,33.7470906524415,-11.7813125373277));
#7748=CARTESIAN_POINT('Ctrl Pts',(3.37058603991502,33.7587609593107,-11.7023986217524));
#7749=CARTESIAN_POINT('Ctrl Pts',(3.65441080124873,33.7704312661799,-11.6130845147065));
#7750=CARTESIAN_POINT('Ctrl Pts',(3.93823556258241,33.782101573049,-11.5237704076606));
#7751=CARTESIAN_POINT('Ctrl Pts',(4.21875289975679,33.7937718799182,-11.4240562182245));
#7752=CARTESIAN_POINT('Ctrl Pts',(4.49519965136699,33.8054421867874,-11.3142224807695));
#7753=CARTESIAN_POINT('Ctrl Pts',(4.75925754080382,33.8165894930335,-11.2093109029254));
#7754=CARTESIAN_POINT('Ctrl Pts',(5.01968053272849,33.8277367992797,-11.0951355152522));
#7755=CARTESIAN_POINT('Ctrl Pts',(5.27581662176582,33.8388841055259,-10.9719738070914));
#7756=CARTESIAN_POINT('Ctrl Pts',(5.53190920612139,33.8500295184035,-10.8488330179308));
#7757=CARTESIAN_POINT('Ctrl Pts',(5.78371610099243,33.8611749312811,-10.7167090711419));
#7758=CARTESIAN_POINT('Ctrl Pts',(6.03060740074508,33.8723203441587,-10.575926655763));
#7759=CARTESIAN_POINT('Ctrl Pts',(6.27747129172809,33.8834645197224,-10.4351598694193));
#7760=CARTESIAN_POINT('Ctrl Pts',(6.51942044562115,33.894608695286,-10.2857366659969));
#7761=CARTESIAN_POINT('Ctrl Pts',(6.75585050286505,33.9057528708497,-10.1280271639119));
#7762=CARTESIAN_POINT('Ctrl Pts',(6.9997262229621,33.9172479991433,-9.96535106919086));
#7763=CARTESIAN_POINT('Ctrl Pts',(7.23772934615604,33.9287431274368,-9.79385847046579));
#7764=CARTESIAN_POINT('Ctrl Pts',(7.46922869419891,33.9402382557304,-9.61400400269085));
#7765=CARTESIAN_POINT('Ctrl Pts',(7.69367223117651,33.951383026867,-9.4396312745173));
#7766=CARTESIAN_POINT('Ctrl Pts',(7.91200235583995,33.9625277980037,-9.25739901926732));
#7767=CARTESIAN_POINT('Ctrl Pts',(8.12367645122317,33.9736725691403,-9.06776329454195));
#7768=CARTESIAN_POINT('Ctrl Pts',(8.3453321155427,33.9853428760124,-8.86918522826218));
#7769=CARTESIAN_POINT('Ctrl Pts',(8.55968867444274,33.9970131828844,-8.66248887742566));
#7770=CARTESIAN_POINT('Ctrl Pts',(8.76616444527815,34.0086834897564,-8.44824308175026));
#7771=CARTESIAN_POINT('Ctrl Pts',(8.97264021611356,34.0203537966285,-8.23399728607487));
#7772=CARTESIAN_POINT('Ctrl Pts',(9.17123497239103,34.0320241035005,-8.01220229322709));
#7773=CARTESIAN_POINT('Ctrl Pts',(9.36141285701635,34.0436944103725,-7.78346963574016));
#7774=CARTESIAN_POINT('Ctrl Pts',(9.54306798782396,34.0548417166199,-7.56498755041451));
#7775=CARTESIAN_POINT('Ctrl Pts',(9.71709831636459,34.0659890228673,-7.34011069825151));
#7776=CARTESIAN_POINT('Ctrl Pts',(9.88306413050669,34.0771363291148,-7.10939474514478));
#7777=CARTESIAN_POINT('Ctrl Pts',(10.049001755376,34.0882817419936,-6.87871797911381));
#7778=CARTESIAN_POINT('Ctrl Pts',(10.2068774448557,34.0994271548725,-6.64220430866783));
#7779=CARTESIAN_POINT('Ctrl Pts',(10.3562934788784,34.1105725677513,-6.40044026839876));
#7780=CARTESIAN_POINT('Ctrl Pts',(10.5056929254003,34.1217167433162,-6.15870306769375));
#7781=CARTESIAN_POINT('Ctrl Pts',(10.6466344516049,34.1328609188811,-5.91171688792114));
#7782=CARTESIAN_POINT('Ctrl Pts',(10.7787645084178,34.1440050944459,-5.66009592869888));
#7783=CARTESIAN_POINT('Ctrl Pts',(10.9150556091398,34.1555002227386,-5.40055091430656));
#7784=CARTESIAN_POINT('Ctrl Pts',(11.04197111863,34.1669953510312,-5.13607473106159));
#7785=CARTESIAN_POINT('Ctrl Pts',(11.1591743840538,34.1784904793238,-4.86736862342257));
#7786=CARTESIAN_POINT('Ctrl Pts',(11.2728054403158,34.1896352504617,-4.60685234237289));
#7787=CARTESIAN_POINT('Ctrl Pts',(11.3773074082572,34.2007800215996,-4.34236042018421));
#7788=CARTESIAN_POINT('Ctrl Pts',(11.4724220783389,34.2119247927375,-4.07455297013576));
#7789=CARTESIAN_POINT('Ctrl Pts',(11.5720219152455,34.2235950996075,-3.79411696248015));
#7790=CARTESIAN_POINT('Ctrl Pts',(11.6613277225691,34.2352654064775,-3.5100455127702));
#7791=CARTESIAN_POINT('Ctrl Pts',(11.7401009596523,34.2469357133476,-3.2231164588285));
#7792=CARTESIAN_POINT('Ctrl Pts',(11.8188741967355,34.2586060202176,-2.93618740488681));
#7793=CARTESIAN_POINT('Ctrl Pts',(11.8871147832217,34.2702763270876,-2.64640107256719));
#7794=CARTESIAN_POINT('Ctrl Pts',(11.9446448465681,34.2819466339576,-2.35455085724545));
#7795=CARTESIAN_POINT('Ctrl Pts',(11.9995967207427,34.2930939402076,-2.07577980473253));
#7796=CARTESIAN_POINT('Ctrl Pts',(12.0447933593859,34.3042412464575,-1.79504252936051));
#7797=CARTESIAN_POINT('Ctrl Pts',(12.0801145768396,34.3153885527074,-1.51303736253506));
#7798=CARTESIAN_POINT('Ctrl Pts',(12.1154297949892,34.3265339655889,-1.23108009425072));
#7799=CARTESIAN_POINT('Ctrl Pts',(12.1408729076176,34.3376793784703,-0.947855629040423));
#7800=CARTESIAN_POINT('Ctrl Pts',(12.1563753727891,34.3488247913517,-0.664069308015263));
#7801=CARTESIAN_POINT('Ctrl Pts',(12.1718761169461,34.3599689669192,-0.380314491679434));
#7802=CARTESIAN_POINT('Ctrl Pts',(12.1774384027462,34.3711131424867,-0.0959982103629502));
#7803=CARTESIAN_POINT('Ctrl Pts',(12.1730457121208,34.3822573180542,0.188171040858175));
#7804=CARTESIAN_POINT('Ctrl Pts',(12.1685146867457,34.3937524463449,0.481289358968064));
#7805=CARTESIAN_POINT('Ctrl Pts',(12.1533915147295,34.4052475746356,0.774250939540593));
#7806=CARTESIAN_POINT('Ctrl Pts',(12.1277161686617,34.4167427029263,1.06627894210765));
#7807=CARTESIAN_POINT('Ctrl Pts',(12.1028233750677,34.4278874740667,1.34940629596561));
#7808=CARTESIAN_POINT('Ctrl Pts',(12.0680121410407,34.4390322452072,1.63165585970076));
#7809=CARTESIAN_POINT('Ctrl Pts',(12.0233716344006,34.4501770163476,1.91232444713011));
#7810=CARTESIAN_POINT('Ctrl Pts',(11.9766260884783,34.4618473232134,2.20622806360036));
#7811=CARTESIAN_POINT('Ctrl Pts',(11.9191020086131,34.4735176300793,2.49839769914427));
#7812=CARTESIAN_POINT('Ctrl Pts',(11.8509621693877,34.4851879369452,2.78803621026358));
#7813=CARTESIAN_POINT('Ctrl Pts',(11.7828223301624,34.496858243811,3.07767472138287));
#7814=CARTESIAN_POINT('Ctrl Pts',(11.7040668169537,34.5085285506769,3.36478178350285));
#7815=CARTESIAN_POINT('Ctrl Pts',(11.6149191198025,34.5201988575427,3.64857562487699));
#7816=CARTESIAN_POINT('Ctrl Pts',(11.5297665448279,34.5313461637786,3.91965134670903));
#7817=CARTESIAN_POINT('Ctrl Pts',(11.4351073244025,34.5424934700145,4.18778524183307));
#7818=CARTESIAN_POINT('Ctrl Pts',(11.3311701091902,34.5536407762504,4.45230661641746));
#7819=CARTESIAN_POINT('Ctrl Pts',(11.2272505477016,34.5647861891177,4.71678306207768));
#7820=CARTESIAN_POINT('Ctrl Pts',(11.1140562351574,34.575931601985,4.97764796404744));
#7821=CARTESIAN_POINT('Ctrl Pts',(10.9918645231726,34.5870770148522,5.2342491872493));
#7822=CARTESIAN_POINT('Ctrl Pts',(10.8696863763659,34.5982211904055,5.49082192372942));
#7823=CARTESIAN_POINT('Ctrl Pts',(10.7385129393202,34.6093653659588,5.743131685842));
#7824=CARTESIAN_POINT('Ctrl Pts',(10.5986687532571,34.6205095415121,5.99054846476783));
#7825=CARTESIAN_POINT('Ctrl Pts',(10.4544205894249,34.6320046698134,6.24575690114288));
#7826=CARTESIAN_POINT('Ctrl Pts',(10.3009468455545,34.6434997981147,6.49575891739394));
#7827=CARTESIAN_POINT('Ctrl Pts',(10.1386543714878,34.6549949264161,6.73989152624218));
#7828=CARTESIAN_POINT('Ctrl Pts',(9.98130836963331,34.6661396975425,6.97658327763416));
#7829=CARTESIAN_POINT('Ctrl Pts',(9.81567339958986,34.6772844686689,7.20775787559392));
#7830=CARTESIAN_POINT('Ctrl Pts',(9.64216426105065,34.6884292397953,7.43284054806221));
#7831=CARTESIAN_POINT('Ctrl Pts',(9.46047323556585,34.7000995466841,7.66853707634841));
#7832=CARTESIAN_POINT('Ctrl Pts',(9.27014774830922,34.7117698535728,7.89755306912699));
#7833=CARTESIAN_POINT('Ctrl Pts',(9.07171219303635,34.7234401604616,8.11926647775005));
#7834=CARTESIAN_POINT('Ctrl Pts',(8.87327663776348,34.7351104673503,8.3409798863731));
#7835=CARTESIAN_POINT('Ctrl Pts',(8.66673124476339,34.7467807742391,8.55539046669953));
#7836=CARTESIAN_POINT('Ctrl Pts',(8.45264636382744,34.7584510811278,8.76191872240749));
#7837=CARTESIAN_POINT('Ctrl Pts',(8.24815561997432,34.769598387403,8.95919148847938));
#7838=CARTESIAN_POINT('Ctrl Pts',(8.03672521997992,34.7807456936781,9.14933180573395));
#7839=CARTESIAN_POINT('Ctrl Pts',(7.81887688946857,34.7918929999533,9.33186018097862));
#7840=CARTESIAN_POINT('Ctrl Pts',(7.60106556046604,34.80303841286,9.514357553804));
#7841=CARTESIAN_POINT('Ctrl Pts',(7.37683868168676,34.8141838257667,9.68924539461946));
#7842=CARTESIAN_POINT('Ctrl Pts',(7.14675186016405,34.8253292386734,9.85608381149641));
#7843=CARTESIAN_POINT('Ctrl Pts',(6.91669058185407,34.8364734142661,10.0229037067164));
#7844=CARTESIAN_POINT('Ctrl Pts',(6.68077087572966,34.8476175898588,10.1816758058499));
#7845=CARTESIAN_POINT('Ctrl Pts',(6.43957919597263,34.8587617654515,10.332002227487));
#7846=CARTESIAN_POINT('Ctrl Pts',(6.19079190131524,34.8702568937233,10.4870627328589));
#7847=CARTESIAN_POINT('Ctrl Pts',(5.93639544874949,34.8817520219951,10.6331368327251));
#7848=CARTESIAN_POINT('Ctrl Pts',(5.67706434630601,34.8932471502669,10.7698370766647));
#7849=CARTESIAN_POINT('Ctrl Pts',(5.4256373309246,34.9043919214323,10.9023708684537));
#7850=CARTESIAN_POINT('Ctrl Pts',(5.16957226213629,34.9155366925976,11.0260936195786));
#7851=CARTESIAN_POINT('Ctrl Pts',(4.90950841371425,34.926681463763,11.1406991425884));
#7852=CARTESIAN_POINT('Ctrl Pts',(4.63718116175636,34.938351770588,11.2607089299149));
#7853=CARTESIAN_POINT('Ctrl Pts',(4.36046921890012,34.950022077413,11.3707208190695));
#7854=CARTESIAN_POINT('Ctrl Pts',(4.08013071339716,34.961692384238,11.4704395561632));
#7855=CARTESIAN_POINT('Ctrl Pts',(3.79979220789422,34.9733626910629,11.5701582932569));
#7856=CARTESIAN_POINT('Ctrl Pts',(3.51582745878504,34.9850329978879,11.6595837741214));
#7857=CARTESIAN_POINT('Ctrl Pts',(3.22901458356905,34.9967033047129,11.7384801004686));
#7858=CARTESIAN_POINT('Ctrl Pts',(2.95505255715356,35.007850715387,11.8138414224685));
#7859=CARTESIAN_POINT('Ctrl Pts',(2.6784101976567,35.0189981260611,11.8796188945309));
#7860=CARTESIAN_POINT('Ctrl Pts',(2.39977509106479,35.0301455367353,11.9356411542198));
#7861=CARTESIAN_POINT('Ctrl Pts',(2.13174790508044,35.040868554199,11.9895305897635));
#7862=CARTESIAN_POINT('Ctrl Pts',(1.86187710718966,35.0515915716628,12.0343936963621));
#7863=CARTESIAN_POINT('Ctrl Pts',(1.59078448392775,35.0623145891265,12.0701224093086));
#7864=CARTESIAN_POINT('Ctrl Pts',(1.59071714630986,32.0622959365534,12.0696162300787));
#7865=CARTESIAN_POINT('Ctrl Pts',(0.955528524672293,32.0874228315995,12.1538996540835));
#7866=CARTESIAN_POINT('Ctrl Pts',(-1.71425060518447,32.1919671345073,12.2972187210211));
#7867=CARTESIAN_POINT('Ctrl Pts',(-6.36996413642198,32.3759288452768,10.9770241092494));
#7868=CARTESIAN_POINT('Ctrl Pts',(-10.8462127664019,32.6141810688619,6.59023292610109));
#7869=CARTESIAN_POINT('Ctrl Pts',(-12.1244826930503,32.7804961191146,2.40607098746999));
#7870=CARTESIAN_POINT('Ctrl Pts',(-12.1754508005637,32.8673937615056,0.190879886591904));
#7871=CARTESIAN_POINT('Ctrl Pts',(-12.175309711376,32.8748739960349,0.000187563072374733));
#7872=CARTESIAN_POINT('',(-12.1744999999831,32.6251260039388,-2.02629457301205E-5));
#7873=CARTESIAN_POINT('Ctrl Pts',(1.59078448392773,31.8125557231064,12.0701224093086));
#7874=CARTESIAN_POINT('Ctrl Pts',(1.30900267453901,31.8237005044403,12.1072599059328));
#7875=CARTESIAN_POINT('Ctrl Pts',(1.02592669881683,31.8348452857743,12.1345247267504));
#7876=CARTESIAN_POINT('Ctrl Pts',(0.742262345110562,31.8459900671082,12.1518515815916));
#7877=CARTESIAN_POINT('Ctrl Pts',(0.458530536541289,31.8571374986507,12.1691825567272));
#7878=CARTESIAN_POINT('Ctrl Pts',(0.174210336700322,31.8682849301933,12.1765708248781));
#7879=CARTESIAN_POINT('Ctrl Pts',(-0.109989332035699,31.8794323617358,12.1740031459187));
#7880=CARTESIAN_POINT('Ctrl Pts',(-0.391949916769597,31.8904919675755,12.1714556965708));
#7881=CARTESIAN_POINT('Ctrl Pts',(-0.673791604467417,31.9015515734153,12.1591086355011));
#7882=CARTESIAN_POINT('Ctrl Pts',(-0.95482342212009,31.912611179255,12.1369997315058));
#7883=CARTESIAN_POINT('Ctrl Pts',(-1.23808376448244,31.9237584855021,12.1147155084335));
#7884=CARTESIAN_POINT('Ctrl Pts',(-1.52060594814084,31.9349057917492,12.0825072854502));
#7885=CARTESIAN_POINT('Ctrl Pts',(-1.80168510862511,31.9460530979963,12.0404477084267));
#7886=CARTESIAN_POINT('Ctrl Pts',(-2.08271652784791,31.9571985108748,11.9983952752174));
#7887=CARTESIAN_POINT('Ctrl Pts',(-2.36230514952321,31.9683439237533,11.9464948680741));
#7888=CARTESIAN_POINT('Ctrl Pts',(-2.63975329031857,31.9794893366318,11.884870753031));
#7889=CARTESIAN_POINT('Ctrl Pts',(-2.91717063006565,31.9906335121966,11.8232534792208));
#7890=CARTESIAN_POINT('Ctrl Pts',(-3.19244770310074,32.0017776877613,11.7519147108885));
#7891=CARTESIAN_POINT('Ctrl Pts',(-3.46489782258198,32.0129218633261,11.6710296601914));
#7892=CARTESIAN_POINT('Ctrl Pts',(-3.74592794981203,32.0244169916189,11.5875973749286));
#7893=CARTESIAN_POINT('Ctrl Pts',(-4.02394989801848,32.0359121199117,11.4940078756693));
#7894=CARTESIAN_POINT('Ctrl Pts',(-4.2982264070027,32.0474072482046,11.3905092074123));
#7895=CARTESIAN_POINT('Ctrl Pts',(-4.56414331051031,32.0585520193422,11.2901650493144));
#7896=CARTESIAN_POINT('Ctrl Pts',(-4.82653944546965,32.0696967904798,11.1805069143616));
#7897=CARTESIAN_POINT('Ctrl Pts',(-5.08476174610048,32.0808415616174,11.0618103507244));
#7898=CARTESIAN_POINT('Ctrl Pts',(-5.35516061315147,32.0925118684879,10.9375166074964));
#7899=CARTESIAN_POINT('Ctrl Pts',(-5.6209822480959,32.1041821753583,10.803311636784));
#7900=CARTESIAN_POINT('Ctrl Pts',(-5.88150296641289,32.1158524822288,10.6595672100736));
#7901=CARTESIAN_POINT('Ctrl Pts',(-6.14202368472985,32.1275227890992,10.5158227833632));
#7902=CARTESIAN_POINT('Ctrl Pts',(-6.39724319690724,32.1391930959697,10.362539070421));
#7903=CARTESIAN_POINT('Ctrl Pts',(-6.64646899845364,32.1508634028401,10.2001421609012));
#7904=CARTESIAN_POINT('Ctrl Pts',(-6.88452583494995,32.1620107090872,10.0450230107282));
#7905=CARTESIAN_POINT('Ctrl Pts',(-7.11718546291348,32.1731580153343,9.88154319117064));
#7906=CARTESIAN_POINT('Ctrl Pts',(-7.3438637301814,32.1843053215814,9.71010379772154));
#7907=CARTESIAN_POINT('Ctrl Pts',(-7.57050349617527,32.19545073446,9.53869352323099));
#7908=CARTESIAN_POINT('Ctrl Pts',(-7.79116371711331,32.2065961473386,9.3593265348274));
#7909=CARTESIAN_POINT('Ctrl Pts',(-8.00529124878566,32.2177415602172,9.17244581734423));
#7910=CARTESIAN_POINT('Ctrl Pts',(-8.2193950089754,32.2288857357819,8.98558584652402));
#7911=CARTESIAN_POINT('Ctrl Pts',(-8.42696732714878,32.2400299113465,8.79121398762406));
#7912=CARTESIAN_POINT('Ctrl Pts',(-8.627489094617,32.2511740869111,8.58981269715847));
#7913=CARTESIAN_POINT('Ctrl Pts',(-8.83432569990824,32.2626692152039,8.3820688709039));
#7914=CARTESIAN_POINT('Ctrl Pts',(-9.03366027000809,32.2741643434968,8.16684589996586));
#7915=CARTESIAN_POINT('Ctrl Pts',(-9.22496414319454,32.2856594717896,7.94471439428599));
#7916=CARTESIAN_POINT('Ctrl Pts',(-9.41043731322679,32.2968042429273,7.72935317950114));
#7917=CARTESIAN_POINT('Ctrl Pts',(-9.58836188649626,32.3079490140649,7.50749853242398));
#7918=CARTESIAN_POINT('Ctrl Pts',(-9.75829629083444,32.3190937852025,7.27970492192416));
#7919=CARTESIAN_POINT('Ctrl Pts',(-9.93624401376104,32.3307640920729,7.04116962094411));
#7920=CARTESIAN_POINT('Ctrl Pts',(-10.1054296870796,32.3424343989434,6.79612202615387));
#7921=CARTESIAN_POINT('Ctrl Pts',(-10.2653957777935,32.3541047058139,6.54523489076284));
#7922=CARTESIAN_POINT('Ctrl Pts',(-10.4253618685074,32.3657750126843,6.2943477553718));
#7923=CARTESIAN_POINT('Ctrl Pts',(-10.576108203647,32.3774453195548,6.03762136698964));
#7924=CARTESIAN_POINT('Ctrl Pts',(-10.7172306218485,32.3891156264253,5.77576125269328));
#7925=CARTESIAN_POINT('Ctrl Pts',(-10.8519688998768,32.4002579882968,5.52574724829742));
#7926=CARTESIAN_POINT('Ctrl Pts',(-10.9779752599429,32.4114003501683,5.27097837052066));
#7927=CARTESIAN_POINT('Ctrl Pts',(-11.0949288753281,32.4225427120399,5.0120857436213));
#7928=CARTESIAN_POINT('Ctrl Pts',(-11.2118624589273,32.4336831654505,4.75323745978609));
#7929=CARTESIAN_POINT('Ctrl Pts',(-11.3197462835136,32.4448236188611,4.49026708040664));
#7930=CARTESIAN_POINT('Ctrl Pts',(-11.418306790496,32.4559640722717,4.22382768210448));
#7931=CARTESIAN_POINT('Ctrl Pts',(-11.5168563332357,32.4671032863762,3.9574179235265));
#7932=CARTESIAN_POINT('Ctrl Pts',(-11.6060845367131,32.4782425004807,3.68754016717926));
#7933=CARTESIAN_POINT('Ctrl Pts',(-11.6857666143717,32.4893817145852,3.41486586624351));
#7934=CARTESIAN_POINT('Ctrl Pts',(-11.7666848528916,32.500693738698,3.13796138822696));
#7935=CARTESIAN_POINT('Ctrl Pts',(-11.8377582625043,32.5120057628108,2.85817315383455));
#7936=CARTESIAN_POINT('Ctrl Pts',(-11.8988041826084,32.5233177869236,2.57621995837733));
#7937=CARTESIAN_POINT('Ctrl Pts',(-11.9589208024357,32.5344576084204,2.29855892826241));
#7938=CARTESIAN_POINT('Ctrl Pts',(-12.009312981119,32.5455974299172,2.01879864552249));
#7939=CARTESIAN_POINT('Ctrl Pts',(-12.0498576548315,32.556737251414,1.73763654090826));
#7940=CARTESIAN_POINT('Ctrl Pts',(-12.0913424556654,32.5681353768348,1.44995500733155));
#7941=CARTESIAN_POINT('Ctrl Pts',(-12.1225175320442,32.5795335022556,1.16080614795246));
#7942=CARTESIAN_POINT('Ctrl Pts',(-12.1433070423736,32.5909316276764,0.870944501468714));
#7943=CARTESIAN_POINT('Ctrl Pts',(-12.1640965527031,32.6023297530972,0.581082854984967));
#7944=CARTESIAN_POINT('Ctrl Pts',(-12.1745004835326,32.613727878518,0.290508720558424));
#7945=CARTESIAN_POINT('Ctrl Pts',(-12.1744999999831,32.6251260039388,-2.02629457920173E-5));
#7946=CARTESIAN_POINT('Ctrl Pts',(-12.1744999999831,32.6251260039651,-2.02636154117562E-5));
#7947=CARTESIAN_POINT('Ctrl Pts',(-12.1744999682797,32.6258732859801,-0.0190678768165046));
#7948=CARTESIAN_POINT('Ctrl Pts',(-12.1744552351083,32.6266205679952,-0.0381154725570181));
#7949=CARTESIAN_POINT('Ctrl Pts',(-12.1743658010439,32.6273678500103,-0.057162858329975));
#7950=CARTESIAN_POINT('Ctrl Pts',(-12.1730317010868,32.6385151562574,-0.341295271704965));
#7951=CARTESIAN_POINT('Ctrl Pts',(-12.1617461874558,32.6496624625045,-0.625423396093907));
#7952=CARTESIAN_POINT('Ctrl Pts',(-12.1405297269587,32.6608097687516,-0.908838928981096));
#7953=CARTESIAN_POINT('Ctrl Pts',(-12.1193168700748,32.6719551816302,-1.19220632377607));
#7954=CARTESIAN_POINT('Ctrl Pts',(-12.0881764538661,32.6831005945087,-1.47486110281071));
#7955=CARTESIAN_POINT('Ctrl Pts',(-12.0471809543266,32.6942460073873,-1.75609831834951));
#7956=CARTESIAN_POINT('Ctrl Pts',(-12.0061900059243,32.7053901829519,-2.03730431218924));
#7957=CARTESIAN_POINT('Ctrl Pts',(-11.9553461973366,32.7165343585165,-2.31709279288919));
#7958=CARTESIAN_POINT('Ctrl Pts',(-11.8947736229075,32.7276785340811,-2.59476602216561));
#7959=CARTESIAN_POINT('Ctrl Pts',(-11.8322934950546,32.739173662374,-2.88118374553293));
#7960=CARTESIAN_POINT('Ctrl Pts',(-11.7594619685466,32.7506687906668,-3.16535053951657));
#7961=CARTESIAN_POINT('Ctrl Pts',(-11.6764720426416,32.7621639189597,-3.44651285902283));
#7962=CARTESIAN_POINT('Ctrl Pts',(-11.5960115460404,32.7733086900973,-3.71910570214559));
#7963=CARTESIAN_POINT('Ctrl Pts',(-11.506002790155,32.7844534612349,-3.98887423638641));
#7964=CARTESIAN_POINT('Ctrl Pts',(-11.4066724115637,32.7955982323725,-4.25514685354945));
#7965=CARTESIAN_POINT('Ctrl Pts',(-11.3026580728741,32.807268539243,-4.53397565273587));
#7966=CARTESIAN_POINT('Ctrl Pts',(-11.1884219401367,32.8189388461134,-4.80897060131908));
#7967=CARTESIAN_POINT('Ctrl Pts',(-11.0642814033507,32.8306091529839,-5.07938256852815));
#7968=CARTESIAN_POINT('Ctrl Pts',(-10.9401408665647,32.8422794598544,-5.34979453573721));
#7969=CARTESIAN_POINT('Ctrl Pts',(-10.8060960736838,32.8539497667249,-5.61562322032863));
#7970=CARTESIAN_POINT('Ctrl Pts',(-10.6625208843845,32.8656200735954,-5.87614658088653));
#7971=CARTESIAN_POINT('Ctrl Pts',(-10.5253799657805,32.8767673798425,-6.12499468033231));
#7972=CARTESIAN_POINT('Ctrl Pts',(-10.3795031187475,32.8879146860897,-6.3690768373752));
#7973=CARTESIAN_POINT('Ctrl Pts',(-10.2252472674586,32.8990619923368,-6.60778091111761));
#7974=CARTESIAN_POINT('Ctrl Pts',(-10.0710176165062,32.9102074052154,-6.84644444100378));
#7975=CARTESIAN_POINT('Ctrl Pts',(-9.9084119473859,32.921352818094,-7.07973148737207));
#7976=CARTESIAN_POINT('Ctrl Pts',(-9.73783124627379,32.9324982309726,-7.30705774365399));
#7977=CARTESIAN_POINT('Ctrl Pts',(-9.56726948226978,32.9436424065372,-7.53435876318956));
#7978=CARTESIAN_POINT('Ctrl Pts',(-9.3887346142411,32.9547865821018,-7.75570010072467));
#7979=CARTESIAN_POINT('Ctrl Pts',(-9.20266950256293,32.9659307576664,-7.97052848163773));
#7980=CARTESIAN_POINT('Ctrl Pts',(-9.01074482252143,32.9774258859592,-8.19212224469573));
#7981=CARTESIAN_POINT('Ctrl Pts',(-8.81080811489427,32.9889210142521,-8.40678596077151));
#7982=CARTESIAN_POINT('Ctrl Pts',(-8.60338944894226,33.0004161425449,-8.6139503272209));
#7983=CARTESIAN_POINT('Ctrl Pts',(-8.40229264490357,33.0115609136825,-8.81480058248823));
#7984=CARTESIAN_POINT('Ctrl Pts',(-8.19416340784828,33.0227056848202,-9.00860166320182));
#7985=CARTESIAN_POINT('Ctrl Pts',(-7.97952213246204,33.0338504559578,-9.19487230947491));
#7986=CARTESIAN_POINT('Ctrl Pts',(-7.75475936973759,33.0455207628282,-9.38992661576092));
#7987=CARTESIAN_POINT('Ctrl Pts',(-7.52285587600274,33.0571910696987,-9.57672298982141));
#7988=CARTESIAN_POINT('Ctrl Pts',(-7.28444883114305,33.0688613765691,-9.75475553135283));
#7989=CARTESIAN_POINT('Ctrl Pts',(-7.04604178628334,33.0805316834396,-9.93278807288427));
#7990=CARTESIAN_POINT('Ctrl Pts',(-6.80113146436942,33.09220199031,-10.1020565881776));
#7991=CARTESIAN_POINT('Ctrl Pts',(-6.55039166588011,33.1038722971805,-10.2621059862763));
#7992=CARTESIAN_POINT('Ctrl Pts',(-6.31088868167215,33.1150196034276,-10.4149828279117));
#7993=CARTESIAN_POINT('Ctrl Pts',(-6.06599569770914,33.1261669096747,-10.5594943509551));
#7994=CARTESIAN_POINT('Ctrl Pts',(-5.81631905191834,33.1373142159218,-10.695273859808));
#7995=CARTESIAN_POINT('Ctrl Pts',(-5.56668481367376,33.1484596288003,-10.8310303065287));
#7996=CARTESIAN_POINT('Ctrl Pts',(-5.31226877001417,33.1596050416789,-10.9580575727416));
#7997=CARTESIAN_POINT('Ctrl Pts',(-5.05370262822269,33.1707504545575,-11.0760344887281));
#7998=CARTESIAN_POINT('Ctrl Pts',(-4.79516519128955,33.1818946301221,-11.1939983074444));
#7999=CARTESIAN_POINT('Ctrl Pts',(-4.53247881883711,33.1930388056867,-11.3029136715195));
#8000=CARTESIAN_POINT('Ctrl Pts',(-4.26629713627511,33.2041829812513,-11.4025066978718));
#8001=CARTESIAN_POINT('Ctrl Pts',(-3.9917328517731,33.2156781095442,-11.5052361109501));
#8002=CARTESIAN_POINT('Ctrl Pts',(-3.71344981544439,33.227173237837,-11.5980463999713));
#8003=CARTESIAN_POINT('Ctrl Pts',(-3.43218589779943,33.2386683661299,-11.6806913413953));
#8004=CARTESIAN_POINT('Ctrl Pts',(-3.15949455312228,33.2498131372675,-11.7608173682115));
#8005=CARTESIAN_POINT('Ctrl Pts',(-2.8840016112494,33.2609579084051,-11.8313884471381));
#8006=CARTESIAN_POINT('Ctrl Pts',(-2.60639431557328,33.2721026795427,-11.8922310321381));
#8007=CARTESIAN_POINT('Ctrl Pts',(-2.31569634698968,33.2837729864132,-11.9559426713433));
#8008=CARTESIAN_POINT('Ctrl Pts',(-2.02268013077371,33.2954432932836,-12.0089861705082));
#8009=CARTESIAN_POINT('Ctrl Pts',(-1.7281472467221,33.3071136001541,-12.0512222344311));
#8010=CARTESIAN_POINT('Ctrl Pts',(-1.43361436267048,33.3187839070246,-12.0934582983541));
#8011=CARTESIAN_POINT('Ctrl Pts',(-1.13756514413288,33.3304542138951,-12.1248868881006));
#8012=CARTESIAN_POINT('Ctrl Pts',(-0.840809011698687,33.3421245207656,-12.1454308468595));
#8013=CARTESIAN_POINT('Ctrl Pts',(-0.557351899073608,33.3532718270128,-12.1650541354633));
#8014=CARTESIAN_POINT('Ctrl Pts',(-0.273165182359102,33.3644191332599,-12.1747527915611));
#8015=CARTESIAN_POINT('Ctrl Pts',(0.0110432552658722,33.375566439507,-12.1744949914365));
#8016=CARTESIAN_POINT('Ctrl Pts',(0.295203420124147,33.3867118523856,-12.1742372350993));
#8017=CARTESIAN_POINT('Ctrl Pts',(0.579385031881237,33.3978572652642,-12.1640263990678));
#8018=CARTESIAN_POINT('Ctrl Pts',(0.862879717510703,33.4090026781428,-12.1438827745951));
#8019=CARTESIAN_POINT('Ctrl Pts',(1.1463429308258,33.4201468537074,-12.1237413863777));
#8020=CARTESIAN_POINT('Ctrl Pts',(1.42911910428315,33.431291029272,-12.0936694305245));
#8021=CARTESIAN_POINT('Ctrl Pts',(1.71050324800708,33.4424352048366,-12.0537392077545));
#8022=CARTESIAN_POINT('Ctrl Pts',(2.00074875005636,33.4539303331295,-12.0125515011501));
#8023=CARTESIAN_POINT('Ctrl Pts',(2.28951283081747,33.4654254614223,-11.9608745844622));
#8024=CARTESIAN_POINT('Ctrl Pts',(2.57602976407282,33.4769205897152,-11.8988453601436));
#8025=CARTESIAN_POINT('Ctrl Pts',(2.85381401900525,33.4880653608528,-11.8387067091201));
#8026=CARTESIAN_POINT('Ctrl Pts',(3.12948580577546,33.4992101319904,-11.7688375157537));
#8027=CARTESIAN_POINT('Ctrl Pts',(3.40235863131859,33.510354903128,-11.689414270779));
#8028=CARTESIAN_POINT('Ctrl Pts',(3.68809887410845,33.5220252099984,-11.6062457938262));
#8029=CARTESIAN_POINT('Ctrl Pts',(3.97076952676866,33.5336955168689,-11.5126006236718));
#8030=CARTESIAN_POINT('Ctrl Pts',(4.24960009200912,33.5453658237393,-11.4087400403373));
#8031=CARTESIAN_POINT('Ctrl Pts',(4.5284306572496,33.5570361306098,-11.3048794570028));
#8032=CARTESIAN_POINT('Ctrl Pts',(4.80342082373608,33.5687064374802,-11.1908035858234));
#8033=CARTESIAN_POINT('Ctrl Pts',(5.07382294533181,33.5803767443507,-11.0668320204756));
#8034=CARTESIAN_POINT('Ctrl Pts',(5.33210709267749,33.5915240505978,-10.9484161964355));
#8035=CARTESIAN_POINT('Ctrl Pts',(5.58628251884841,33.6026713568449,-10.8209367603774));
#8036=CARTESIAN_POINT('Ctrl Pts',(5.83571242790281,33.6138186630921,-10.6847045213623));
#8037=CARTESIAN_POINT('Ctrl Pts',(6.0850999713191,33.6249640759706,-10.5484954213756));
#8038=CARTESIAN_POINT('Ctrl Pts',(6.32974337283193,33.6361094888492,-10.4035366143671));
#8039=CARTESIAN_POINT('Ctrl Pts',(6.56903034562025,33.6472549017278,-10.2501849041039));
#8040=CARTESIAN_POINT('Ctrl Pts',(6.80829075383676,33.6583990772924,-10.0968502182633));
#8041=CARTESIAN_POINT('Ctrl Pts',(7.04219569621666,33.669543252857,-9.93512463360258));
#8042=CARTESIAN_POINT('Ctrl Pts',(7.27016074531316,33.6806874284215,-9.76540900256142));
#8043=CARTESIAN_POINT('Ctrl Pts',(7.50530487692386,33.6921825567144,-9.59034868151615));
#8044=CARTESIAN_POINT('Ctrl Pts',(7.73412869047147,33.7036776850073,-9.40678708310855));
#8045=CARTESIAN_POINT('Ctrl Pts',(7.95602534278516,33.7151728133001,-9.21521084918627));
#8046=CARTESIAN_POINT('Ctrl Pts',(8.17115886224074,33.7263175844377,-9.02947361963365));
#8047=CARTESIAN_POINT('Ctrl Pts',(8.37978101882481,33.7374623555753,-8.83620325463972));
#8048=CARTESIAN_POINT('Ctrl Pts',(8.5813734858511,33.7486071267129,-8.63588324066113));
#8049=CARTESIAN_POINT('Ctrl Pts',(8.79247211891656,33.7602774335834,-8.42611706362923));
#8050=CARTESIAN_POINT('Ctrl Pts',(8.9958619094496,33.7719477404539,-8.20862060647202));
#8051=CARTESIAN_POINT('Ctrl Pts',(9.19099134494893,33.7836180473244,-7.98399200569952));
#8052=CARTESIAN_POINT('Ctrl Pts',(9.38612078044827,33.7952883541949,-7.75936340492701));
#8053=CARTESIAN_POINT('Ctrl Pts',(9.5729896475206,33.8069586610653,-7.52760291957819));
#8054=CARTESIAN_POINT('Ctrl Pts',(9.75109440402037,33.8186289679358,-7.28934895404814));
#8055=CARTESIAN_POINT('Ctrl Pts',(9.92121745963443,33.8297762741829,-7.0617722546679));
#8056=CARTESIAN_POINT('Ctrl Pts',(10.0833954685513,33.8409235804299,-6.82820331985479));
#8057=CARTESIAN_POINT('Ctrl Pts',(10.2372180184085,33.852070886677,-6.58921979399478));
#8058=CARTESIAN_POINT('Ctrl Pts',(10.3910144415251,33.8632162995555,-6.35027685945628));
#8059=CARTESIAN_POINT('Ctrl Pts',(10.5364580946447,33.874361712434,-6.10592139420272));
#8060=CARTESIAN_POINT('Ctrl Pts',(10.6731820964191,33.8855071253125,-5.85675970026768));
#8061=CARTESIAN_POINT('Ctrl Pts',(10.8098909197054,33.8966513008771,-5.60762566715114));
#8062=CARTESIAN_POINT('Ctrl Pts',(10.9378818963315,33.9077954764416,-5.35368670459261));
#8063=CARTESIAN_POINT('Ctrl Pts',(11.0568336864415,33.9189396520062,-5.09557446029115));
#8064=CARTESIAN_POINT('Ctrl Pts',(11.1795315100773,33.9304347802991,-4.82933373705156));
#8065=CARTESIAN_POINT('Ctrl Pts',(11.2926114639304,33.941929908592,-4.55865288790684));
#8066=CARTESIAN_POINT('Ctrl Pts',(11.3957735795933,33.9534250368849,-4.28424961605228));
#8067=CARTESIAN_POINT('Ctrl Pts',(11.4957914427987,33.9645698080224,-4.01820981325158));
#8068=CARTESIAN_POINT('Ctrl Pts',(11.5864869838508,33.97571457916,-3.7486713984846));
#8069=CARTESIAN_POINT('Ctrl Pts',(11.6676364475165,33.9868593502975,-3.47630694539264));
#8070=CARTESIAN_POINT('Ctrl Pts',(11.7526125436312,33.9985296571681,-3.19109904753701));
#8071=CARTESIAN_POINT('Ctrl Pts',(11.8271205113252,34.0101999640387,-2.90279247716342));
#8072=CARTESIAN_POINT('Ctrl Pts',(11.8909623210325,34.0218702709092,-2.61217635885952));
#8073=CARTESIAN_POINT('Ctrl Pts',(11.9548041307399,34.0335405777798,-2.32156024055564));
#8074=CARTESIAN_POINT('Ctrl Pts',(12.0079797190489,34.0452108846504,-2.02863490389215));
#8075=CARTESIAN_POINT('Ctrl Pts',(12.0503524473524,34.056881191521,-1.73420187538456));
#8076=CARTESIAN_POINT('Ctrl Pts',(12.0908262570107,34.0680284977683,-1.45296375761318));
#8077=CARTESIAN_POINT('Ctrl Pts',(12.1214562644126,34.0791758040156,-1.17026611606645));
#8078=CARTESIAN_POINT('Ctrl Pts',(12.142158528628,34.0903231102629,-0.886812559488088));
#8079=CARTESIAN_POINT('Ctrl Pts',(12.1628572765665,34.1014685231416,-0.603407147460176));
#8080=CARTESIAN_POINT('Ctrl Pts',(12.1736316284451,34.1126139360204,-0.319246342673114));
#8081=CARTESIAN_POINT('Ctrl Pts',(12.1744495802706,34.1237593488991,-0.0350380856780686));
#8082=CARTESIAN_POINT('Ctrl Pts',(12.1752674412908,34.1349035244639,0.249138619785386));
#8083=CARTESIAN_POINT('Ctrl Pts',(12.1661311086289,34.1460477000287,0.533362500259884));
#8084=CARTESIAN_POINT('Ctrl Pts',(12.1470606956327,34.1571918755935,0.816925153619469));
#8085=CARTESIAN_POINT('Ctrl Pts',(12.1273897165896,34.1686870038862,1.10941777099075));
#8086=CARTESIAN_POINT('Ctrl Pts',(12.0971488397799,34.1801821321789,1.40120654292002));
#8087=CARTESIAN_POINT('Ctrl Pts',(12.0564181252866,34.1916772604716,1.69151773217481));
#8088=CARTESIAN_POINT('Ctrl Pts',(12.0169288321053,34.2028220316094,1.97298059892988));
#8089=CARTESIAN_POINT('Ctrl Pts',(11.9675797055986,34.2139668027472,2.25305434264466));
#8090=CARTESIAN_POINT('Ctrl Pts',(11.9084961294965,34.225111573885,2.53104132399424));
#8091=CARTESIAN_POINT('Ctrl Pts',(11.8466264458957,34.2367818807552,2.82213688245413));
#8092=CARTESIAN_POINT('Ctrl Pts',(11.7740822255187,34.2484521876253,3.11094382810151));
#8093=CARTESIAN_POINT('Ctrl Pts',(11.6910672154904,34.2601224944955,3.39667449321921));
#8094=CARTESIAN_POINT('Ctrl Pts',(11.608052205462,34.2717928013657,3.68240515833693));
#8095=CARTESIAN_POINT('Ctrl Pts',(11.5145665078164,34.2834631082358,3.96505922319547));
#8096=CARTESIAN_POINT('Ctrl Pts',(11.4108737097382,34.295133415106,4.24386750858299));
#8097=CARTESIAN_POINT('Ctrl Pts',(11.3118278672755,34.3062807213527,4.51018110049645));
#8098=CARTESIAN_POINT('Ctrl Pts',(11.2034400892115,34.3174280275994,4.77306556836597));
#8099=CARTESIAN_POINT('Ctrl Pts',(11.0859733768434,34.3285753338461,5.03186292916634));
#8100=CARTESIAN_POINT('Ctrl Pts',(10.9685266161816,34.3397207467242,5.29061633326782));
#8101=CARTESIAN_POINT('Ctrl Pts',(10.8420041101378,34.3508661596023,5.54528377345437));
#8102=CARTESIAN_POINT('Ctrl Pts',(10.7067165369335,34.3620115724805,5.79522831713764));
#8103=CARTESIAN_POINT('Ctrl Pts',(10.5714439827516,34.3731557480446,6.04514511309366));
#8104=CARTESIAN_POINT('Ctrl Pts',(10.4274084313955,34.3842999236088,6.29033982499244));
#8105=CARTESIAN_POINT('Ctrl Pts',(10.2749665443453,34.395444099173,6.53020005532642));
#8106=CARTESIAN_POINT('Ctrl Pts',(10.117723952571,34.4069392274662,6.77761397161364));
#8107=CARTESIAN_POINT('Ctrl Pts',(9.95153713121388,34.4184343557593,7.01935171891168));
#8108=CARTESIAN_POINT('Ctrl Pts',(9.77684664447996,34.4299294840525,7.25477221836227));
#8109=CARTESIAN_POINT('Ctrl Pts',(9.60748050563951,34.4410742551897,7.48301739496749));
#8110=CARTESIAN_POINT('Ctrl Pts',(9.43012155403504,34.4522190263269,7.7053244809599));
#8111=CARTESIAN_POINT('Ctrl Pts',(9.24521373484962,34.4633637974641,7.92114090563651));
#8112=CARTESIAN_POINT('Ctrl Pts',(9.05158652023803,34.4750341043353,8.14713423226626));
#8113=CARTESIAN_POINT('Ctrl Pts',(8.84968157512732,34.4867044112064,8.36600978804986));
#8114=CARTESIAN_POINT('Ctrl Pts',(8.64005473522879,34.4983747180776,8.5771734517993));
#8115=CARTESIAN_POINT('Ctrl Pts',(8.43042789533026,34.5100450249488,8.78833711554873));
#8116=CARTESIAN_POINT('Ctrl Pts',(8.21307940324054,34.52171533182,8.99178865534857));
#8117=CARTESIAN_POINT('Ctrl Pts',(7.98860879055077,34.5333856386912,9.18697882013097));
#8118=CARTESIAN_POINT('Ctrl Pts',(7.77419774798598,34.5445329449391,9.37342160757606));
#8119=CARTESIAN_POINT('Ctrl Pts',(7.55322486774204,34.5556802511869,9.55238288856828));
#8120=CARTESIAN_POINT('Ctrl Pts',(7.32623595483955,34.5668275574348,9.72341076906742));
#8121=CARTESIAN_POINT('Ctrl Pts',(7.09928559597489,34.5779729703142,9.89440960050293));
#8122=CARTESIAN_POINT('Ctrl Pts',(6.8663214574821,34.5891183831935,10.0574775612436));
#8123=CARTESIAN_POINT('Ctrl Pts',(6.62792113425293,34.6002637960728,10.21220405633));
#8124=CARTESIAN_POINT('Ctrl Pts',(6.38954727716328,34.6114079716382,10.3669133743718));
#8125=CARTESIAN_POINT('Ctrl Pts',(6.14573866412806,34.6225521472035,10.5132829307159));
#8126=CARTESIAN_POINT('Ctrl Pts',(5.89710152521208,34.6336963227689,10.6509456787339));
#8127=CARTESIAN_POINT('Ctrl Pts',(5.64063429770819,34.6451914510612,10.7929437063363));
#8128=CARTESIAN_POINT('Ctrl Pts',(5.37902975093839,34.6566865793535,10.925677496898));
#8129=CARTESIAN_POINT('Ctrl Pts',(5.11298151220474,34.6681817076457,11.0487949707582));
#8130=CARTESIAN_POINT('Ctrl Pts',(4.85504209151608,34.6793264787841,11.1681599777785));
#8131=CARTESIAN_POINT('Ctrl Pts',(4.59292609736622,34.6904712499225,11.2784860573086));
#8132=CARTESIAN_POINT('Ctrl Pts',(4.327287770841,34.7016160210608,11.3795004634795));
#8133=CARTESIAN_POINT('Ctrl Pts',(4.04912317254728,34.7132863279301,11.4852782406623));
#8134=CARTESIAN_POINT('Ctrl Pts',(3.7670963520758,34.7249566347993,11.5808449099814));
#8135=CARTESIAN_POINT('Ctrl Pts',(3.48197968126939,34.7366269416685,11.6659447859669));
#8136=CARTESIAN_POINT('Ctrl Pts',(3.19686301046297,34.7482972485378,11.7510446619523));
#8137=CARTESIAN_POINT('Ctrl Pts',(2.90865681331852,34.759967555407,11.8256776570603));
#8138=CARTESIAN_POINT('Ctrl Pts',(2.61815035720158,34.7716378622762,11.8896483950151));
#8139=CARTESIAN_POINT('Ctrl Pts',(2.34066544362123,34.7827850640849,11.9507517347836));
#8140=CARTESIAN_POINT('Ctrl Pts',(2.06099907596949,34.7939322658936,12.0021458934422));
#8141=CARTESIAN_POINT('Ctrl Pts',(1.77984673713931,34.8050794677023,12.0436952735568));
#8142=CARTESIAN_POINT('Ctrl Pts',(1.71689781304658,34.8075752831859,12.0529980194839));
#8143=CARTESIAN_POINT('Ctrl Pts',(1.65387443840511,34.8100710986695,12.0618074546403));
#8144=CARTESIAN_POINT('Ctrl Pts',(1.59078448392778,34.8125669141531,12.0701224093086));
#8145=CARTESIAN_POINT('Origin',(0.,13.3748739960349,0.));
#8146=CARTESIAN_POINT('',(1.59078448392772,38.0622997972676,12.0701224093087));
#8147=CARTESIAN_POINT('',(1.59078448392769,37.8125509746976,12.0701224093087));
#8148=CARTESIAN_POINT('',(1.59078448392774,13.3748739960349,12.0701224093086));
#8149=CARTESIAN_POINT('',(-12.1744999966649,35.8748739960676,-0.000284967810357368));
#8150=CARTESIAN_POINT('Ctrl Pts',(-12.1744999966649,35.8748739960676,-0.000284967810371163));
#8151=CARTESIAN_POINT('Ctrl Pts',(-12.1744930883501,35.8864472961776,-0.295424542797684));
#8152=CARTESIAN_POINT('Ctrl Pts',(-12.163749488268,35.8980205962875,-0.590512724686085));
#8153=CARTESIAN_POINT('Ctrl Pts',(-12.1423063610032,35.9095938963975,-0.884786124179511));
#8154=CARTESIAN_POINT('Ctrl Pts',(-12.1208567139894,35.9211707153511,-1.17914899703588));
#8155=CARTESIAN_POINT('Ctrl Pts',(-12.0887010545349,35.9327475343047,-1.47269637376915));
#8156=CARTESIAN_POINT('Ctrl Pts',(-12.0459284961632,35.9443243532583,-1.76466906680104));
#8157=CARTESIAN_POINT('Ctrl Pts',(-12.0392930536843,35.9461203018566,-1.80996371560749));
#8158=CARTESIAN_POINT('Ctrl Pts',(-12.0324022028897,35.9479162504549,-1.85522048095315));
#8159=CARTESIAN_POINT('Ctrl Pts',(-12.0252563877582,35.9497121990533,-1.90043654423916));
#8160=CARTESIAN_POINT('Ctrl Pts',(-11.9809028943906,35.9608595059425,-2.18108897173295));
#8161=CARTESIAN_POINT('Ctrl Pts',(-11.9267134419172,35.9720068128318,-2.46022991528048));
#8162=CARTESIAN_POINT('Ctrl Pts',(-11.8628155407781,35.9831541197211,-2.73716234364608));
#8163=CARTESIAN_POINT('Ctrl Pts',(-11.7989284926723,35.9942995332446,-3.01404773514772));
#8164=CARTESIAN_POINT('Ctrl Pts',(-11.7253363480305,36.0054449467682,-3.28872510056579));
#8165=CARTESIAN_POINT('Ctrl Pts',(-11.6422175183502,36.0165903602918,-3.56050860207074));
#8166=CARTESIAN_POINT('Ctrl Pts',(-11.559107916142,36.0277345365026,-3.8322619314151));
#8167=CARTESIAN_POINT('Ctrl Pts',(-11.466473818764,36.0388787127133,-4.10112178333928));
#8168=CARTESIAN_POINT('Ctrl Pts',(-11.3645435686143,36.0500228889241,-4.36641726442477));
#8169=CARTESIAN_POINT('Ctrl Pts',(-11.2594033383302,36.0615180167336,-4.64006741179234));
#8170=CARTESIAN_POINT('Ctrl Pts',(-11.1443720573033,36.0730131445432,-4.90992477220224));
#8171=CARTESIAN_POINT('Ctrl Pts',(-11.0197546303388,36.0845082723527,-5.17527372581657));
#8172=CARTESIAN_POINT('Ctrl Pts',(-10.8989353748965,36.0956530441313,-5.43253520030673));
#8173=CARTESIAN_POINT('Ctrl Pts',(-10.7691057848687,36.1067978159099,-5.68555876622977));
#8174=CARTESIAN_POINT('Ctrl Pts',(-10.6305916042168,36.1179425876886,-5.93371488987754));
#8175=CARTESIAN_POINT('Ctrl Pts',(-10.4855457583789,36.1296128935136,-6.19357286748642));
#8176=CARTESIAN_POINT('Ctrl Pts',(-10.3309767217692,36.1412831993385,-6.44809302920758));
#8177=CARTESIAN_POINT('Ctrl Pts',(-10.1673116861847,36.1529535051635,-6.69658295894055));
#8178=CARTESIAN_POINT('Ctrl Pts',(-10.0036466506002,36.1646238109885,-6.9450728886735));
#8179=CARTESIAN_POINT('Ctrl Pts',(-9.83088580791383,36.1762941168134,-7.18753231105948));
#8180=CARTESIAN_POINT('Ctrl Pts',(-9.64950806513854,36.1879644226384,-7.42330413972284));
#8181=CARTESIAN_POINT('Ctrl Pts',(-9.47625871296853,36.199111727114,-7.6485099226974));
#8182=CARTESIAN_POINT('Ctrl Pts',(-9.29509606919364,36.2102590315895,-7.8676816020831));
#8183=CARTESIAN_POINT('Ctrl Pts',(-9.10646565514324,36.221406336065,-8.0802681590215));
#8184=CARTESIAN_POINT('Ctrl Pts',(-8.91786728005395,36.2325517471659,-8.2928186080371));
#8185=CARTESIAN_POINT('Ctrl Pts',(-8.72180384403198,36.2436971582667,-8.49878596821237));
#8186=CARTESIAN_POINT('Ctrl Pts',(-8.51876020628826,36.2548425693675,-8.69765340754388));
#8187=CARTESIAN_POINT('Ctrl Pts',(-8.31573910957317,36.2659867431529,-8.89649876947028));
#8188=CARTESIAN_POINT('Ctrl Pts',(-8.10573954903184,36.2771309169383,-9.08824559786713));
#8189=CARTESIAN_POINT('Ctrl Pts',(-7.88928307487955,36.2882750907237,-9.27241407694993));
#8190=CARTESIAN_POINT('Ctrl Pts',(-7.66600988509742,36.2997702203486,-9.46238244792694));
#8191=CARTESIAN_POINT('Ctrl Pts',(-7.43586672490532,36.3112653499736,-9.64428721563409));
#8192=CARTESIAN_POINT('Ctrl Pts',(-7.19946377540692,36.3227604795986,-9.81764592947839));
#8193=CARTESIAN_POINT('Ctrl Pts',(-6.97026615536178,36.3339052489754,-9.98572084018279));
#8194=CARTESIAN_POINT('Ctrl Pts',(-6.73518490496334,36.3450500183522,-10.1457627683423));
#8195=CARTESIAN_POINT('Ctrl Pts',(-6.49480730688629,36.3561947877291,-10.2973748254794));
#8196=CARTESIAN_POINT('Ctrl Pts',(-6.24309451396523,36.3678650974781,-10.4561362685081));
#8197=CARTESIAN_POINT('Ctrl Pts',(-5.98557411618706,36.3795354072272,-10.6056535064113));
#8198=CARTESIAN_POINT('Ctrl Pts',(-5.7229525669938,36.3912057169763,-10.7455229824304));
#8199=CARTESIAN_POINT('Ctrl Pts',(-5.46033101780052,36.4028760267254,-10.8853924584494));
#8200=CARTESIAN_POINT('Ctrl Pts',(-5.19260861744099,36.4145463364744,-11.0156140226206));
#8201=CARTESIAN_POINT('Ctrl Pts',(-4.9205203219068,36.4262166462235,-11.1358398880238));
#8202=CARTESIAN_POINT('Ctrl Pts',(-4.66062554473769,36.4373639561281,-11.2506778836736));
#8203=CARTESIAN_POINT('Ctrl Pts',(-4.39666996201338,36.4485112660327,-11.3564306914372));
#8204=CARTESIAN_POINT('Ctrl Pts',(-4.12930845682457,36.4596585759373,-11.4528276822101));
#8205=CARTESIAN_POINT('Ctrl Pts',(-3.86199236269481,36.4708039924835,-11.5492083000596));
#8206=CARTESIAN_POINT('Ctrl Pts',(-3.59127175189979,36.4819494090297,-11.6362361830668));
#8207=CARTESIAN_POINT('Ctrl Pts',(-3.31781968883708,36.4930948255759,-11.7136895452443));
#8208=CARTESIAN_POINT('Ctrl Pts',(-3.04439798317911,36.5042390048086,-11.7911343089017));
#8209=CARTESIAN_POINT('Ctrl Pts',(-2.76824568734694,36.5153831840413,-11.8590066015354));
#8210=CARTESIAN_POINT('Ctrl Pts',(-2.49005036894981,36.526527363274,-11.9171346979923));
#8211=CARTESIAN_POINT('Ctrl Pts',(-2.20309427787332,36.5380224888186,-11.9770933322249));
#8212=CARTESIAN_POINT('Ctrl Pts',(-1.91396469214712,36.5495176143631,-12.0266840376984));
#8213=CARTESIAN_POINT('Ctrl Pts',(-1.62342826198514,36.5610127399077,-12.065775189692));
#8214=CARTESIAN_POINT('Ctrl Pts',(-1.34174686044864,36.5721575146694,-12.1036749135756));
#8215=CARTESIAN_POINT('Ctrl Pts',(-1.05874337738828,36.5833022894311,-12.1317055846882));
#8216=CARTESIAN_POINT('Ctrl Pts',(-0.775123413472737,36.5944470641928,-12.149799749127));
#8217=CARTESIAN_POINT('Ctrl Pts',(-0.478129494697926,36.6061173651288,-12.1687471346687));
#8218=CARTESIAN_POINT('Ctrl Pts',(-0.180459873677726,36.6177876660647,-12.1767983435379));
#8219=CARTESIAN_POINT('Ctrl Pts',(0.11707202117144,36.6294579670007,-12.1739370949524));
#8220=CARTESIAN_POINT('Ctrl Pts',(0.414603916020578,36.6411282679367,-12.1710758463669));
#8221=CARTESIAN_POINT('Ctrl Pts',(0.711997749299544,36.6527985688726,-12.1573021523303));
#8222=CARTESIAN_POINT('Ctrl Pts',(1.00844175372276,36.6644688698086,-12.1326623409435));
#8223=CARTESIAN_POINT('Ctrl Pts',(1.29160072405077,36.6756161703009,-12.1091267540628));
#8224=CARTESIAN_POINT('Ctrl Pts',(1.57397769503675,36.6867634707932,-12.0756705357027));
#8225=CARTESIAN_POINT('Ctrl Pts',(1.85486813075634,36.6979107712855,-12.0323694452716));
#8226=CARTESIAN_POINT('Ctrl Pts',(2.13571085696984,36.7090561783983,-11.9890757095716));
#8227=CARTESIAN_POINT('Ctrl Pts',(2.41506728847831,36.720201585511,-11.9359404808946));
#8228=CARTESIAN_POINT('Ctrl Pts',(2.69224029849889,36.7313469926238,-11.8730911065796));
#8229=CARTESIAN_POINT('Ctrl Pts',(2.96938253809598,36.7424911624267,-11.8102487095019));
#8230=CARTESIAN_POINT('Ctrl Pts',(3.24434158014842,36.7536353322296,-11.7376943791884));
#8231=CARTESIAN_POINT('Ctrl Pts',(3.51643151935759,36.7647795020325,-11.655606360017));
#8232=CARTESIAN_POINT('Ctrl Pts',(3.79709037410433,36.776274634646,-11.5709331467551));
#8233=CARTESIAN_POINT('Ctrl Pts',(4.07469619766536,36.7877697672594,-11.4761161021925));
#8234=CARTESIAN_POINT('Ctrl Pts',(4.34851283179752,36.7992648998728,-11.3714065269734));
#8235=CARTESIAN_POINT('Ctrl Pts',(4.61398364177174,36.8104096653299,-11.2698884587465));
#8236=CARTESIAN_POINT('Ctrl Pts',(4.87589256715123,36.821554430787,-11.159072070423));
#8237=CARTESIAN_POINT('Ctrl Pts',(5.13358776672708,36.8326991962441,-11.039235792903));
#8238=CARTESIAN_POINT('Ctrl Pts',(5.40343503015256,36.8443695124357,-10.9137484279808));
#8239=CARTESIAN_POINT('Ctrl Pts',(5.66866130576691,36.8560398286273,-10.7783701409865));
#8240=CARTESIAN_POINT('Ctrl Pts',(5.92854455678638,36.8677101448189,-10.6334758986983));
#8241=CARTESIAN_POINT('Ctrl Pts',(6.18842780780583,36.8793804610105,-10.4885816564102));
#8242=CARTESIAN_POINT('Ctrl Pts',(6.4429677454689,36.8910507772021,-10.3341716298738));
#8243=CARTESIAN_POINT('Ctrl Pts',(6.69147375292597,36.9027210933937,-10.1706749659943));
#8244=CARTESIAN_POINT('Ctrl Pts',(6.92884298123643,36.9138684051906,-10.0145053935419));
#8245=CARTESIAN_POINT('Ctrl Pts',(7.16077810612801,36.9250157169876,-9.84999907333248));
#8246=CARTESIAN_POINT('Ctrl Pts',(7.38669675289892,36.9361630287846,-9.67755967848882));
#8247=CARTESIAN_POINT('Ctrl Pts',(7.61257702739218,36.9473084472108,-9.50514957247294));
#8248=CARTESIAN_POINT('Ctrl Pts',(7.83244265202763,36.9584538656371,-9.32480924375483));
#8249=CARTESIAN_POINT('Ctrl Pts',(8.0457424448486,36.9695992840634,-9.13698411737493));
#8250=CARTESIAN_POINT('Ctrl Pts',(8.25901855777424,36.9807434651591,-8.94917984277024));
#8251=CARTESIAN_POINT('Ctrl Pts',(8.46573009427768,36.9918876462549,-8.75389260599716));
#8252=CARTESIAN_POINT('Ctrl Pts',(8.66536008199898,37.0030318273506,-8.55160715300338));
#8253=CARTESIAN_POINT('Ctrl Pts',(8.87127664691684,37.0145269514863,-8.34295149916703));
#8254=CARTESIAN_POINT('Ctrl Pts',(9.06965820838166,37.026022075622,-8.12684992765588));
#8255=CARTESIAN_POINT('Ctrl Pts',(9.25997863188271,37.0375171997577,-7.90387537775461));
#8256=CARTESIAN_POINT('Ctrl Pts',(9.44449848305687,37.0486619763178,-7.68769663032144));
#8257=CARTESIAN_POINT('Ctrl Pts',(9.62144111262719,37.0598067528779,-7.46505786145395));
#8258=CARTESIAN_POINT('Ctrl Pts',(9.79036740214472,37.070951529438,-7.23651548613157));
#8259=CARTESIAN_POINT('Ctrl Pts',(9.96725925054946,37.0826218273615,-6.99719641196586));
#8260=CARTESIAN_POINT('Ctrl Pts',(10.1353603737896,37.094292125285,-6.75140383280313));
#8261=CARTESIAN_POINT('Ctrl Pts',(10.2942162169648,37.1059624232084,-6.49981251486365));
#8262=CARTESIAN_POINT('Ctrl Pts',(10.4530720601401,37.1176327211319,-6.24822119692417));
#8263=CARTESIAN_POINT('Ctrl Pts',(10.6026824515541,37.1293030190554,-5.99083142857654));
#8264=CARTESIAN_POINT('Ctrl Pts',(10.742646351938,37.1409733169788,-5.72835051364639));
#8265=CARTESIAN_POINT('Ctrl Pts',(10.8763379661845,37.1521206268483,-5.47763231324153));
#8266=CARTESIAN_POINT('Ctrl Pts',(11.0012686005856,37.1632679367179,-5.22219436487314));
#8267=CARTESIAN_POINT('Ctrl Pts',(11.1171200677777,37.1744152465874,-4.9626698105571));
#8268=CARTESIAN_POINT('Ctrl Pts',(11.2329518581578,37.1855606631402,-4.70318933523264));
#8269=CARTESIAN_POINT('Ctrl Pts',(11.3397074513444,37.196706079693,-4.43962388319863));
#8270=CARTESIAN_POINT('Ctrl Pts',(11.4371160292913,37.2078514962458,-4.17262833026484));
#8271=CARTESIAN_POINT('Ctrl Pts',(11.5345137937413,37.2189956755263,-3.90566241697496));
#8272=CARTESIAN_POINT('Ctrl Pts',(11.6225665235307,37.2301398548069,-3.63526741367178));
#8273=CARTESIAN_POINT('Ctrl Pts',(11.7010522555776,37.2412840340875,-3.3621163516812));
#8274=CARTESIAN_POINT('Ctrl Pts',(11.782009616388,37.2527791596272,-3.08036336926517));
#8275=CARTESIAN_POINT('Ctrl Pts',(11.8527875672035,37.2642742851669,-2.79567821335521));
#8276=CARTESIAN_POINT('Ctrl Pts',(11.9131983041429,37.2757694107066,-2.50881573977965));
#8277=CARTESIAN_POINT('Ctrl Pts',(11.971767831112,37.2869141856162,-2.23069631542371));
#8278=CARTESIAN_POINT('Ctrl Pts',(12.0205926768578,37.2980589605257,-1.95053060259384));
#8279=CARTESIAN_POINT('Ctrl Pts',(12.0595535357516,37.3092037354353,-1.6690173061836));
#8280=CARTESIAN_POINT('Ctrl Pts',(12.1003515732662,37.3208740362901,-1.37422939970866));
#8281=CARTESIAN_POINT('Ctrl Pts',(12.1303329348627,37.3325443371448,-1.07796407739402));
#8282=CARTESIAN_POINT('Ctrl Pts',(12.1494213968046,37.3442146379996,-0.781031352038081));
#8283=CARTESIAN_POINT('Ctrl Pts',(12.1685098587465,37.3558849388544,-0.484098626682174));
#8284=CARTESIAN_POINT('Ctrl Pts',(12.1767054082705,37.3675552397091,-0.186498833656002));
#8285=CARTESIAN_POINT('Ctrl Pts',(12.1739943825377,37.3792255405639,0.110955053691345));
#8286=CARTESIAN_POINT('Ctrl Pts',(12.1714048572777,37.3903728116839,0.395077902726157));
#8287=CARTESIAN_POINT('Ctrl Pts',(12.1588640971083,37.4015200828038,0.679152499465869));
#8288=CARTESIAN_POINT('Ctrl Pts',(12.1363956968827,37.4126673539238,0.962470643026071));
#8289=CARTESIAN_POINT('Ctrl Pts',(12.1139311132748,37.4238127315012,1.24574066046157));
#8290=CARTESIAN_POINT('Ctrl Pts',(12.0815422775253,37.4349581090787,1.52825421544422));
#8291=CARTESIAN_POINT('Ctrl Pts',(12.0393047783483,37.4461034866561,1.80930669153689));
#8292=CARTESIAN_POINT('Ctrl Pts',(11.9970719685101,37.4572476268389,2.09032796430773));
#8293=CARTESIAN_POINT('Ctrl Pts',(11.9449927182814,37.4683917670218,2.36988821838241));
#8294=CARTESIAN_POINT('Ctrl Pts',(11.8831942023772,37.4795359072047,2.64729027471258));
#8295=CARTESIAN_POINT('Ctrl Pts',(11.8194491765883,37.49103106195,2.93342985227278));
#8296=CARTESIAN_POINT('Ctrl Pts',(11.7453627483409,37.5025262166954,3.21727278043161));
#8297=CARTESIAN_POINT('Ctrl Pts',(11.6611312464288,37.5140213714408,3.49806636637472));
#8298=CARTESIAN_POINT('Ctrl Pts',(11.5794674609318,37.525166107437,3.77030022960688));
#8299=CARTESIAN_POINT('Ctrl Pts',(11.4882680468647,37.5363108434333,4.0396676423719));
#8300=CARTESIAN_POINT('Ctrl Pts',(11.387762605013,37.5474555794296,4.30549800857771));
#8301=CARTESIAN_POINT('Ctrl Pts',(11.282516944386,37.5591259435495,4.58386594558306));
#8302=CARTESIAN_POINT('Ctrl Pts',(11.1670664275532,37.5707963076694,4.85835486815289));
#8303=CARTESIAN_POINT('Ctrl Pts',(11.0417317581506,37.5824666717893,5.12821704211602));
#8304=CARTESIAN_POINT('Ctrl Pts',(10.916397088748,37.5941370359092,5.39807921607914));
#8305=CARTESIAN_POINT('Ctrl Pts',(10.7811784160682,37.6058074000291,5.66331434083362));
#8306=CARTESIAN_POINT('Ctrl Pts',(10.6364527948914,37.617477764149,5.92320202188377));
#8307=CARTESIAN_POINT('Ctrl Pts',(10.4982123241924,37.6286251796242,6.171444144219));
#8308=CARTESIAN_POINT('Ctrl Pts',(10.3512569086563,37.6397725950994,6.41488166047602));
#8309=CARTESIAN_POINT('Ctrl Pts',(10.1959461834747,37.6509200105746,6.65290400304169));
#8310=CARTESIAN_POINT('Ctrl Pts',(10.0406618319041,37.6620655330859,6.89088592657842));
#8311=CARTESIAN_POINT('Ctrl Pts',(9.87702514909113,37.6732110555971,7.12345428902473));
#8312=CARTESIAN_POINT('Ctrl Pts',(9.70543970866531,37.6843565781084,7.35002655175222));
#8313=CARTESIAN_POINT('Ctrl Pts',(9.53387331491802,37.6955008634215,7.57657366404129));
#8314=CARTESIAN_POINT('Ctrl Pts',(9.35436008645345,37.7066451487347,7.79712579310566));
#8315=CARTESIAN_POINT('Ctrl Pts',(9.16734533347097,37.7177894340478,8.01113161712426));
#8316=CARTESIAN_POINT('Ctrl Pts',(8.97444438432203,37.7292844801883,8.23187316782137));
#8317=CARTESIAN_POINT('Ctrl Pts',(8.77356223729382,37.7407795263289,8.44564942636432));
#8318=CARTESIAN_POINT('Ctrl Pts',(8.56523145482439,37.7522745724694,8.65189345607578));
#8319=CARTESIAN_POINT('Ctrl Pts',(8.36324692134798,37.7634194522824,8.85185480422498));
#8320=CARTESIAN_POINT('Ctrl Pts',(8.15426104066122,37.7745643320955,9.04473583466634));
#8321=CARTESIAN_POINT('Ctrl Pts',(7.93879633762425,37.7857092119086,9.23005758160391));
#8322=CARTESIAN_POINT('Ctrl Pts',(7.71317695122258,37.7973793412128,9.42411339790049));
#8323=CARTESIAN_POINT('Ctrl Pts',(7.48045361358973,37.8090494705171,9.6098800618625));
#8324=CARTESIAN_POINT('Ctrl Pts',(7.24126569578255,37.8207195998213,9.78685451884735));
#8325=CARTESIAN_POINT('Ctrl Pts',(7.00207777797537,37.8323897291256,9.96382897583221));
#8326=CARTESIAN_POINT('Ctrl Pts',(6.75642555486916,37.8440598584298,10.1320110333703));
#8327=CARTESIAN_POINT('Ctrl Pts',(6.50498479025111,37.8557299877341,10.2909486019804));
#8328=CARTESIAN_POINT('Ctrl Pts',(6.26481566441368,37.8668769660599,10.4427612842787));
#8329=CARTESIAN_POINT('Ctrl Pts',(6.01929383228136,37.8780239443856,10.5861854242557));
#8330=CARTESIAN_POINT('Ctrl Pts',(5.76902720315409,37.8891709227114,10.7208570263421));
#8331=CARTESIAN_POINT('Ctrl Pts',(5.51880378713731,37.9003159763075,10.8555053749135));
#8332=CARTESIAN_POINT('Ctrl Pts',(5.2638374446795,37.9114610299036,10.9814040766123));
#8333=CARTESIAN_POINT('Ctrl Pts',(5.00476124753254,37.9226060834997,11.0982347742872));
#8334=CARTESIAN_POINT('Ctrl Pts',(4.73415303693159,37.9342472263137,11.220265846185));
#8335=CARTESIAN_POINT('Ctrl Pts',(4.45906105304134,37.9458883691277,11.3324031528928));
#8336=CARTESIAN_POINT('Ctrl Pts',(4.18023221178463,37.9575295119417,11.4343390235535));
#8337=CARTESIAN_POINT('Ctrl Pts',(3.91331152914864,37.9686734874808,11.5319214402763));
#8338=CARTESIAN_POINT('Ctrl Pts',(3.64296676375931,37.97981746302,11.6201554471051));
#8339=CARTESIAN_POINT('Ctrl Pts',(3.36987168481286,37.9909614385591,11.6988210977815));
#8340=CARTESIAN_POINT('Ctrl Pts',(3.0967812092452,38.0021052262518,11.7774854224442));
#8341=CARTESIAN_POINT('Ctrl Pts',(2.82094076958306,38.0132490139445,11.8465816411191));
#8342=CARTESIAN_POINT('Ctrl Pts',(2.54303836545634,38.0243928016372,11.90593995121));
#8343=CARTESIAN_POINT('Ctrl Pts',(2.26510329492608,38.0355378992411,11.9653052386514));
#8344=CARTESIAN_POINT('Ctrl Pts',(1.98510603667008,38.0466829968449,12.0149302753719));
#8345=CARTESIAN_POINT('Ctrl Pts',(1.70374521241877,38.0578280944488,12.0546962840695));
#8346=CARTESIAN_POINT('Ctrl Pts',(1.66611545400818,38.0593186620551,12.060014669471));
#8347=CARTESIAN_POINT('Ctrl Pts',(1.62846131738319,38.0608092296613,12.0651567826123));
#8348=CARTESIAN_POINT('Ctrl Pts',(1.59078448392772,38.0622997972676,12.0701224093087));
#8349=CARTESIAN_POINT('Ctrl Pts',(1.59078448392775,35.0623145891265,12.0701224093086));
#8350=CARTESIAN_POINT('Ctrl Pts',(1.30904352310633,35.0734587995694,12.1072545222867));
#8351=CARTESIAN_POINT('Ctrl Pts',(1.0259830707147,35.0846030100123,12.1345202070283));
#8352=CARTESIAN_POINT('Ctrl Pts',(0.742308280011921,35.0957472204552,12.1518487756977));
#8353=CARTESIAN_POINT('Ctrl Pts',(0.447013787609849,35.1073479127754,12.1698871458912));
#8354=CARTESIAN_POINT('Ctrl Pts',(0.15105387917742,35.1189486050956,12.1771572388848));
#8355=CARTESIAN_POINT('Ctrl Pts',(-0.144772198628088,35.1305492974159,12.1736391954298));
#8356=CARTESIAN_POINT('Ctrl Pts',(-0.428971912206157,35.1416940668668,12.1702594158319));
#8357=CARTESIAN_POINT('Ctrl Pts',(-0.713047829445617,35.1528388363178,12.1569231801871));
#8358=CARTESIAN_POINT('Ctrl Pts',(-0.996292022982744,35.1639836057687,12.1336660764561));
#8359=CARTESIAN_POINT('Ctrl Pts',(-1.27954579202879,35.1751287519858,12.1104081864827));
#8360=CARTESIAN_POINT('Ctrl Pts',(-1.56196751558968,35.186273898203,12.0772287831481));
#8361=CARTESIAN_POINT('Ctrl Pts',(-1.84285396305103,35.1974190444201,12.0342153678945));
#8362=CARTESIAN_POINT('Ctrl Pts',(-2.12379262655591,35.2085662624903,11.9911939565613));
#8363=CARTESIAN_POINT('Ctrl Pts',(-2.40319518021695,35.2197134805605,11.9383349222077));
#8364=CARTESIAN_POINT('Ctrl Pts',(-2.68036673719162,35.2308606986307,11.8757772126357));
#8365=CARTESIAN_POINT('Ctrl Pts',(-2.71430555813908,35.2322256418531,11.8681172098301));
#8366=CARTESIAN_POINT('Ctrl Pts',(-2.74821094278368,35.2335905850756,11.8603118549257));
#8367=CARTESIAN_POINT('Ctrl Pts',(-2.78208162737386,35.234955528298,11.8523614553653));
#8368=CARTESIAN_POINT('Ctrl Pts',(-3.05869891833734,35.2461028346214,11.7874316195767));
#8369=CARTESIAN_POINT('Ctrl Pts',(-3.33308347439181,35.2572501409449,11.7128040752968));
#8370=CARTESIAN_POINT('Ctrl Pts',(-3.60454956580541,35.2683974472683,11.628657389297));
#8371=CARTESIAN_POINT('Ctrl Pts',(-3.87596954873944,35.2795428602232,11.5445249956007));
#8372=CARTESIAN_POINT('Ctrl Pts',(-4.14447180200817,35.2906882731782,11.4508767671221));
#8373=CARTESIAN_POINT('Ctrl Pts',(-4.40938551257707,35.3018336861331,11.3479412076145));
#8374=CARTESIAN_POINT('Ctrl Pts',(-4.67426981361024,35.3129778617741,11.2450170755525));
#8375=CARTESIAN_POINT('Ctrl Pts',(-4.93556611887974,35.3241220374151,11.1328077678666));
#8376=CARTESIAN_POINT('Ctrl Pts',(-5.19262220129422,35.3352662130561,11.0115904811533));
#8377=CARTESIAN_POINT('Ctrl Pts',(-5.45777349882183,35.3467613412917,10.8865558173052));
#8378=CARTESIAN_POINT('Ctrl Pts',(-5.71841290697268,35.3582564695273,10.7519367395924));
#8379=CARTESIAN_POINT('Ctrl Pts',(-5.97384924005414,35.3697515977629,10.6080900970488));
#8380=CARTESIAN_POINT('Ctrl Pts',(-6.22150019559629,35.3808963689756,10.4686277188988));
#8381=CARTESIAN_POINT('Ctrl Pts',(-6.46426030265943,35.3920411401884,10.320492072634));
#8382=CARTESIAN_POINT('Ctrl Pts',(-6.70152576426192,35.4031859114012,10.164054441065));
#8383=CARTESIAN_POINT('Ctrl Pts',(-6.94997956062108,35.4148562181482,10.00023993897));
#8384=CARTESIAN_POINT('Ctrl Pts',(-7.19240777343378,35.4265265248952,9.82732182100846));
#8385=CARTESIAN_POINT('Ctrl Pts',(-7.42815137572714,35.4381968316421,9.64577717912264));
#8386=CARTESIAN_POINT('Ctrl Pts',(-7.66389497802051,35.4498671383891,9.4642325372368));
#8387=CARTESIAN_POINT('Ctrl Pts',(-7.89295370933529,35.4615374451361,9.27406158308408));
#8388=CARTESIAN_POINT('Ctrl Pts',(-8.11470759005776,35.4732077518831,9.0757903775847));
#8389=CARTESIAN_POINT('Ctrl Pts',(-8.32652365126632,35.4843550580777,8.88640462404963));
#8390=CARTESIAN_POINT('Ctrl Pts',(-8.53173846022696,35.4955023642722,8.68957211823678));
#8391=CARTESIAN_POINT('Ctrl Pts',(-8.72983535399109,35.5066496704667,8.48577780419729));
#8392=CARTESIAN_POINT('Ctrl Pts',(-8.92789860102508,35.5177950832929,8.28201810459399));
#8393=CARTESIAN_POINT('Ctrl Pts',(-9.11884616072902,35.528940496119,8.07129914875044));
#8394=CARTESIAN_POINT('Ctrl Pts',(-9.30219836495137,35.5400859089451,7.85414259032112));
#8395=CARTESIAN_POINT('Ctrl Pts',(-9.48553021423546,35.5512300844576,7.63701013963763));
#8396=CARTESIAN_POINT('Ctrl Pts',(-9.66126821973614,35.56237425997,7.41344171722012));
#8397=CARTESIAN_POINT('Ctrl Pts',(-9.82897233455958,35.5735184354825,7.18399283800189));
#8398=CARTESIAN_POINT('Ctrl Pts',(-10.0019577940555,35.5850135638146,6.94731814552835));
#8399=CARTESIAN_POINT('Ctrl Pts',(-10.1663949731909,35.5965086921468,6.70438685320291));
#8400=CARTESIAN_POINT('Ctrl Pts',(-10.3218477339838,35.6080038204789,6.45584305931104));
#8401=CARTESIAN_POINT('Ctrl Pts',(-10.4725624875548,35.6191485915657,6.21487457179775));
#8402=CARTESIAN_POINT('Ctrl Pts',(-10.6148322327911,35.6302933626525,5.96863087732274));
#8403=CARTESIAN_POINT('Ctrl Pts',(-10.7483044718205,35.6414381337393,5.71772692868804));
#8404=CARTESIAN_POINT('Ctrl Pts',(-10.8880706444308,35.6531084406941,5.45499151008326));
#8405=CARTESIAN_POINT('Ctrl Pts',(-11.0181894980664,35.6647787476489,5.18714603041487));
#8406=CARTESIAN_POINT('Ctrl Pts',(-11.1383106735327,35.6764490546037,4.91492477967551));
#8407=CARTESIAN_POINT('Ctrl Pts',(-11.2584318489989,35.6881193615585,4.64270352893615));
#8408=CARTESIAN_POINT('Ctrl Pts',(-11.3685552188829,35.6997896685134,4.36610681761556));
#8409=CARTESIAN_POINT('Ctrl Pts',(-11.4683881438355,35.7114599754682,4.08589324778976));
#8410=CARTESIAN_POINT('Ctrl Pts',(-11.5636605180159,35.7225971614369,3.81848034680994));
#8411=CARTESIAN_POINT('Ctrl Pts',(-11.6495908466594,35.7337343474056,3.54769134091233));
#8412=CARTESIAN_POINT('Ctrl Pts',(-11.7259574475739,35.7448715333744,3.27419794570916));
#8413=CARTESIAN_POINT('Ctrl Pts',(-11.8023132777083,35.7560071485493,3.00074312413884));
#8414=CARTESIAN_POINT('Ctrl Pts',(-11.8691079996121,35.7671427637243,2.72458493211118));
#8415=CARTESIAN_POINT('Ctrl Pts',(-11.9261699500892,35.7782783788992,2.44640973093008));
#8416=CARTESIAN_POINT('Ctrl Pts',(-11.9832242232964,35.7894124958583,2.16827195619616));
#8417=CARTESIAN_POINT('Ctrl Pts',(-12.0305482866717,35.8005466128173,1.88811797652426));
#8418=CARTESIAN_POINT('Ctrl Pts',(-12.0680214761787,35.8116807297764,1.60664492047536));
#8419=CARTESIAN_POINT('Ctrl Pts',(-12.1054959778234,35.8228152366007,1.32516200854266));
#8420=CARTESIAN_POINT('Ctrl Pts',(-12.1331188783859,35.833949743425,1.04236019299949));
#8421=CARTESIAN_POINT('Ctrl Pts',(-12.1508211493447,35.8450842502493,0.758943770405247));
#8422=CARTESIAN_POINT('Ctrl Pts',(-12.1666082922634,35.8550141655112,0.506188879272841));
#8423=CARTESIAN_POINT('Ctrl Pts',(-12.1745059239959,35.864944080773,0.252945394476219));
#8424=CARTESIAN_POINT('Ctrl Pts',(-12.1744999966649,35.8748739960349,-0.000284966977105543));
#8425=CARTESIAN_POINT('',(-12.1744999990795,35.6251260039956,-0.000149711562892353));
#8426=CARTESIAN_POINT('Ctrl Pts',(1.59078448392778,34.8125669141531,12.0701224093086));
#8427=CARTESIAN_POINT('Ctrl Pts',(1.3090559178938,34.8237119930029,12.1072528887129));
#8428=CARTESIAN_POINT('Ctrl Pts',(1.02599923070556,34.8348570718527,12.1345189599205));
#8429=CARTESIAN_POINT('Ctrl Pts',(0.742319374086524,34.8460021507025,12.1518480979996));
#8430=CARTESIAN_POINT('Ctrl Pts',(0.45866727424099,34.8571461390574,12.1691755405019));
#8431=CARTESIAN_POINT('Ctrl Pts',(0.174392392915168,34.8682901274123,12.1765679752301));
#8432=CARTESIAN_POINT('Ctrl Pts',(-0.109796879691469,34.8794341157672,12.1740048831603));
#8433=CARTESIAN_POINT('Ctrl Pts',(-0.394010203114441,34.8905790472331,12.1714415741771));
#8434=CARTESIAN_POINT('Ctrl Pts',(-0.678137636520358,34.901723978699,12.1589210539924));
#8435=CARTESIAN_POINT('Ctrl Pts',(-0.96147096144561,34.9128689101649,12.1364749346875));
#8436=CARTESIAN_POINT('Ctrl Pts',(-1.24480084680939,34.9240137063354,12.1140290878701));
#8437=CARTESIAN_POINT('Ctrl Pts',(-1.52733637715058,34.9351585025059,12.0816579059211));
#8438=CARTESIAN_POINT('Ctrl Pts',(-1.80837370794537,34.9463032986765,12.0394449532531));
#8439=CARTESIAN_POINT('Ctrl Pts',(-2.08947599074481,34.957450670579,11.9972222445293));
#8440=CARTESIAN_POINT('Ctrl Pts',(-2.36907911783929,34.9685980424816,11.9451532576149));
#8441=CARTESIAN_POINT('Ctrl Pts',(-2.64648707988667,34.9797454143842,11.8833731064035));
#8442=CARTESIAN_POINT('Ctrl Pts',(-2.89654218866479,34.9897936382099,11.8276845734663));
#8443=CARTESIAN_POINT('Ctrl Pts',(-3.14481365690257,34.9998418620356,11.7641062220393));
#8444=CARTESIAN_POINT('Ctrl Pts',(-3.39080016893301,35.0098900858613,11.6927723173063));
#8445=CARTESIAN_POINT('Ctrl Pts',(-3.66369287414124,35.0210373921087,11.6136358554125));
#8446=CARTESIAN_POINT('Ctrl Pts',(-3.93385472728386,35.0321846983561,11.5249300100742));
#8447=CARTESIAN_POINT('Ctrl Pts',(-4.2006101415968,35.0433320046035,11.4268685425323));
#8448=CARTESIAN_POINT('Ctrl Pts',(-4.46732024753654,35.0544774174824,11.3288237307182));
#8449=CARTESIAN_POINT('Ctrl Pts',(-4.73062481951636,35.0656228303613,11.2214265612428));
#8450=CARTESIAN_POINT('Ctrl Pts',(-4.98986574788541,35.0767682432401,11.1049398948432));
#8451=CARTESIAN_POINT('Ctrl Pts',(-5.24907789648335,35.087912418805,10.9884661602735));
#8452=CARTESIAN_POINT('Ctrl Pts',(-5.50422705905017,35.0990565943698,10.8629050530442));
#8453=CARTESIAN_POINT('Ctrl Pts',(-5.75467620310551,35.1102007699347,10.7285671013147));
#8454=CARTESIAN_POINT('Ctrl Pts',(-6.01301249949139,35.1216958982273,10.5899985745793));
#8455=CARTESIAN_POINT('Ctrl Pts',(-6.26634768811219,35.13319102652,10.4420915758961));
#8456=CARTESIAN_POINT('Ctrl Pts',(-6.51400994570775,35.1446861548126,10.2852381925369));
#8457=CARTESIAN_POINT('Ctrl Pts',(-6.75412376698239,35.1558309259505,10.1331655044178));
#8458=CARTESIAN_POINT('Ctrl Pts',(-6.98890510846411,35.1669756970883,9.97268385469279));
#8459=CARTESIAN_POINT('Ctrl Pts',(-7.21777016470715,35.1781204682262,9.80419522956695));
#8460=CARTESIAN_POINT('Ctrl Pts',(-7.45742743582955,35.1897907750962,9.6277614621073));
#8461=CARTESIAN_POINT('Ctrl Pts',(-7.69059677083969,35.2014610819663,9.44254759390848));
#8462=CARTESIAN_POINT('Ctrl Pts',(-7.9166446754192,35.2131313888363,9.24906413282754));
#8463=CARTESIAN_POINT('Ctrl Pts',(-8.14269257999871,35.2248016957063,9.05558067174661));
#8464=CARTESIAN_POINT('Ctrl Pts',(-8.36161880497301,35.2364720025764,8.85382784261666));
#8465=CARTESIAN_POINT('Ctrl Pts',(-8.57283138154773,35.2481423094464,8.64436303920366));
#8466=CARTESIAN_POINT('Ctrl Pts',(-8.7745785421954,35.2592896156963,8.44428532588983));
#8467=CARTESIAN_POINT('Ctrl Pts',(-8.96934848056512,35.2704369219463,8.23711190810849));
#8468=CARTESIAN_POINT('Ctrl Pts',(-9.15665028193266,35.2815842281962,8.02335377908656));
#8469=CARTESIAN_POINT('Ctrl Pts',(-9.34392027011314,35.2927296410776,7.80963195685556));
#8470=CARTESIAN_POINT('Ctrl Pts',(-9.52372447804811,35.303875053959,7.58932785684307));
#8471=CARTESIAN_POINT('Ctrl Pts',(-9.69561083324766,35.3150204668404,7.36298722124455));
#8472=CARTESIAN_POINT('Ctrl Pts',(-9.8674781063922,35.3261646424078,7.13667171297192));
#8473=CARTESIAN_POINT('Ctrl Pts',(-10.0314291207498,35.3373088179753,6.90432121967417));
#8474=CARTESIAN_POINT('Ctrl Pts',(-10.1870531218382,35.3484529935428,6.66651325228162));
#8475=CARTESIAN_POINT('Ctrl Pts',(-10.3475780388049,35.3599481218335,6.42121622899009));
#8476=CARTESIAN_POINT('Ctrl Pts',(-10.4992428040734,35.3714432501243,6.17011267067247));
#8477=CARTESIAN_POINT('Ctrl Pts',(-10.6416451441391,35.382938378415,5.91386835127568));
#8478=CARTESIAN_POINT('Ctrl Pts',(-10.7797072387721,35.3940831495554,5.6654340386276));
#8479=CARTESIAN_POINT('Ctrl Pts',(-10.9090630261503,35.4052279206958,5.41216793644504));
#8480=CARTESIAN_POINT('Ctrl Pts',(-11.0293922551297,35.4163726918363,5.15470239029231));
#8481=CARTESIAN_POINT('Ctrl Pts',(-11.1553956525465,35.4280429987021,4.8850959629249));
#8482=CARTESIAN_POINT('Ctrl Pts',(-11.2715005718733,35.439713305568,4.61088479720244));
#8483=CARTESIAN_POINT('Ctrl Pts',(-11.3773950641872,35.4513836124339,4.33282030592177));
#8484=CARTESIAN_POINT('Ctrl Pts',(-11.4832895565011,35.4630539192998,4.05475581464107));
#8485=CARTESIAN_POINT('Ctrl Pts',(-11.578973510603,35.4747242261657,3.77283831446075));
#8486=CARTESIAN_POINT('Ctrl Pts',(-11.6641938765588,35.4863945330316,3.48784051528297));
#8487=CARTESIAN_POINT('Ctrl Pts',(-11.7486157263752,35.4979554889427,3.20551314986525));
#8488=CARTESIAN_POINT('Ctrl Pts',(-11.8227942500949,35.5095164448538,2.92007971671269));
#8489=CARTESIAN_POINT('Ctrl Pts',(-11.8865239621894,35.521077400765,2.63229906095355));
#8490=CARTESIAN_POINT('Ctrl Pts',(-11.9482806334632,35.5322804351166,2.35342795401509));
#8491=CARTESIAN_POINT('Ctrl Pts',(-12.0002256656454,35.5434834694682,2.07235304358251));
#8492=CARTESIAN_POINT('Ctrl Pts',(-12.042223537602,35.5546865038198,1.78977722647935));
#8493=CARTESIAN_POINT('Ctrl Pts',(-12.0862340710423,35.5664264205107,1.49365954554348));
#8494=CARTESIAN_POINT('Ctrl Pts',(-12.119320691996,35.5781663372016,1.19589388457444));
#8495=CARTESIAN_POINT('Ctrl Pts',(-12.1413881016093,35.5899062538925,0.897298844366037));
#8496=CARTESIAN_POINT('Ctrl Pts',(-12.1634555112226,35.6016461705834,0.598703804157665));
#8497=CARTESIAN_POINT('Ctrl Pts',(-12.1745036811867,35.6133860872742,0.299279713519359));
#8498=CARTESIAN_POINT('Ctrl Pts',(-12.1744999990795,35.6251260039651,-0.00014971078451594));
#8499=CARTESIAN_POINT('Ctrl Pts',(-12.1744999990795,35.6251260039956,-0.000149711562934393));
#8500=CARTESIAN_POINT('Ctrl Pts',(-12.174496426179,35.6365176701443,-0.290696921273105));
#8501=CARTESIAN_POINT('Ctrl Pts',(-12.1640875501384,35.647909336293,-0.58120652559487));
#8502=CARTESIAN_POINT('Ctrl Pts',(-12.1433074390434,35.6593010024416,-0.870938970808622));
#8503=CARTESIAN_POINT('Ctrl Pts',(-12.1225204619165,35.670696432552,-1.16076714756995));
#8504=CARTESIAN_POINT('Ctrl Pts',(-12.0913554174435,35.6820918626624,-1.44981741179922));
#8505=CARTESIAN_POINT('Ctrl Pts',(-12.0498983619847,35.6934872927729,-1.73735422865857));
#8506=CARTESIAN_POINT('Ctrl Pts',(-12.0121118806754,35.7038737807208,-1.99943276838512));
#8507=CARTESIAN_POINT('Ctrl Pts',(-11.9657758328564,35.7142602686687,-2.26025391982292));
#8508=CARTESIAN_POINT('Ctrl Pts',(-11.9109926366114,35.7246467566166,-2.51926669104116));
#8509=CARTESIAN_POINT('Ctrl Pts',(-11.8521965285982,35.7357940628915,-2.79725234936639));
#8510=CARTESIAN_POINT('Ctrl Pts',(-11.783655703664,35.7469413691664,-3.0732202996823));
#8511=CARTESIAN_POINT('Ctrl Pts',(-11.7055335188614,35.7580886754414,-3.34648103069664));
#8512=CARTESIAN_POINT('Ctrl Pts',(-11.6274246031012,35.7692340883479,-3.61969534841323));
#8513=CARTESIAN_POINT('Ctrl Pts',(-11.5397376498562,35.7803795012544,-3.89020310848564));
#8514=CARTESIAN_POINT('Ctrl Pts',(-11.4426862708534,35.7915249141608,-4.15732860823185));
#8515=CARTESIAN_POINT('Ctrl Pts',(-11.3456456660616,35.8026690897533,-4.42442445289702));
#8516=CARTESIAN_POINT('Ctrl Pts',(-11.2392428024865,35.8138132653458,-4.68813853636811));
#8517=CARTESIAN_POINT('Ctrl Pts',(-11.1237403838462,35.8249574409383,-4.94781266043789));
#8518=CARTESIAN_POINT('Ctrl Pts',(-11.004600559911,35.8364525692102,-5.21566444905335));
#8519=CARTESIAN_POINT('Ctrl Pts',(-10.8757788785789,35.8479476974822,-5.47921742693672));
#8520=CARTESIAN_POINT('Ctrl Pts',(-10.7376168148967,35.8594428257542,-5.73777268514943));
#8521=CARTESIAN_POINT('Ctrl Pts',(-10.6036657578032,35.8705875969194,-5.98844750305287));
#8522=CARTESIAN_POINT('Ctrl Pts',(-10.4609353850308,35.8817323680846,-6.23442449239448));
#8523=CARTESIAN_POINT('Ctrl Pts',(-10.30978353461,35.8928771392499,-6.47509179235978));
#8524=CARTESIAN_POINT('Ctrl Pts',(-10.1515040647607,35.9045474460752,-6.72710784471055));
#8525=CARTESIAN_POINT('Ctrl Pts',(-9.98398994001832,35.9162177529005,-6.97330112872041));
#8526=CARTESIAN_POINT('Ctrl Pts',(-9.80770356017696,35.9278880597258,-7.21300222692966));
#8527=CARTESIAN_POINT('Ctrl Pts',(-9.63141718033562,35.9395583665511,-7.45270332513889));
#8528=CARTESIAN_POINT('Ctrl Pts',(-9.4463587512404,35.9512286733765,-7.68591197247079));
#8529=CARTESIAN_POINT('Ctrl Pts',(-9.25304049328369,35.9628989802018,-7.91199670624631));
#8530=CARTESIAN_POINT('Ctrl Pts',(-9.06838572400005,35.9740462863956,-8.12794953343979));
#8531=CARTESIAN_POINT('Ctrl Pts',(-8.87614002640509,35.9851935925894,-8.33746742022859));
#8532=CARTESIAN_POINT('Ctrl Pts',(-8.67677679908099,35.9963408987832,-8.54002310470703));
#8533=CARTESIAN_POINT('Ctrl Pts',(-8.47744743357855,36.0074863116083,-8.74254438512533));
#8534=CARTESIAN_POINT('Ctrl Pts',(-8.27100313898243,36.0186317244334,-8.93810563411376));
#8535=CARTESIAN_POINT('Ctrl Pts',(-8.05795483269958,36.0297771372585,-9.1262157636215));
#8536=CARTESIAN_POINT('Ctrl Pts',(-7.84493017808824,36.0409213127697,-9.31430500998273));
#8537=CARTESIAN_POINT('Ctrl Pts',(-7.62530317567703,36.0520654882808,-9.49494461212312));
#8538=CARTESIAN_POINT('Ctrl Pts',(-7.39961947215846,36.063209663792,-9.66768234466014));
#8539=CARTESIAN_POINT('Ctrl Pts',(-7.16682852840535,36.0747047921249,-9.84585994079197));
#8540=CARTESIAN_POINT('Ctrl Pts',(-6.9275934559246,36.0861999204578,-10.0156297224767));
#8541=CARTESIAN_POINT('Ctrl Pts',(-6.68254854954543,36.0976950487907,-10.1765414131211));
#8542=CARTESIAN_POINT('Ctrl Pts',(-6.44497230785367,36.1088398198755,-10.3325487150986));
#8543=CARTESIAN_POINT('Ctrl Pts',(-6.2019353743058,36.1199845909603,-10.4802297442823));
#8544=CARTESIAN_POINT('Ctrl Pts',(-5.95404475521485,36.1311293620451,-10.6192184883304));
#8545=CARTESIAN_POINT('Ctrl Pts',(-5.69446476074719,36.1427996690021,-10.7647612988788));
#8546=CARTESIAN_POINT('Ctrl Pts',(-5.429562588848,36.154469975959,-10.9007721676023));
#8547=CARTESIAN_POINT('Ctrl Pts',(-5.16006460113188,36.166140282916,-11.0268845809751));
#8548=CARTESIAN_POINT('Ctrl Pts',(-4.89056661341578,36.1778105898729,-11.1529969943479));
#8549=CARTESIAN_POINT('Ctrl Pts',(-4.61647311747857,36.1894808968299,-11.2692108181213));
#8550=CARTESIAN_POINT('Ctrl Pts',(-4.33853605764074,36.2011512037868,-11.3752167067951));
#8551=CARTESIAN_POINT('Ctrl Pts',(-4.07305464777408,36.2122985101097,-11.4764719794663));
#8552=CARTESIAN_POINT('Ctrl Pts',(-3.80398730860846,36.2234458164327,-11.5684443772484));
#8553=CARTESIAN_POINT('Ctrl Pts',(-3.53200203188287,36.2345931227556,-11.6508974717305));
#8554=CARTESIAN_POINT('Ctrl Pts',(-3.26006295181857,36.2457385357101,-11.7333365615659));
#8555=CARTESIAN_POINT('Ctrl Pts',(-2.98520717886023,36.2568839486646,-11.8062594987885));
#8556=CARTESIAN_POINT('Ctrl Pts',(-2.70811833795219,36.2680293616191,-11.8694795723169));
#8557=CARTESIAN_POINT('Ctrl Pts',(-2.43106025821149,36.2791735372596,-11.9326926274346));
#8558=CARTESIAN_POINT('Ctrl Pts',(-2.1517698655459,36.2903177129001,-11.9862049104721));
#8559=CARTESIAN_POINT('Ctrl Pts',(-1.87094268199846,36.3014618885405,-12.0298804537151));
#8560=CARTESIAN_POINT('Ctrl Pts',(-1.5812716833385,36.3129570167765,-12.0749314280132));
#8561=CARTESIAN_POINT('Ctrl Pts',(-1.28996582371931,36.3244521450124,-12.1095160101662));
#8562=CARTESIAN_POINT('Ctrl Pts',(-0.997797531322615,36.3359472732484,-12.1335423655455));
#8563=CARTESIAN_POINT('Ctrl Pts',(-0.714534160316956,36.3470920444607,-12.1568364278884));
#8564=CARTESIAN_POINT('Ctrl Pts',(-0.430460427915619,36.358236815673,-12.1702063130348));
#8565=CARTESIAN_POINT('Ctrl Pts',(-0.146284477231075,36.3693815868853,-12.1736211170597));
#8566=CARTESIAN_POINT('Ctrl Pts',(0.151291888549954,36.3810518936331,-12.1771969473476));
#8567=CARTESIAN_POINT('Ctrl Pts',(0.448980027019182,36.3927222003809,-12.169856231212));
#8568=CARTESIAN_POINT('Ctrl Pts',(0.745966753667841,36.4043925071286,-12.1516247412608));
#8569=CARTESIAN_POINT('Ctrl Pts',(1.04295348031647,36.4160628138764,-12.1333932513097));
#8570=CARTESIAN_POINT('Ctrl Pts',(1.33923846081193,36.4277331206241,-12.1042710168617));
#8571=CARTESIAN_POINT('Ctrl Pts',(1.63401340472503,36.4394034273719,-12.0643462501363));
#8572=CARTESIAN_POINT('Ctrl Pts',(1.91557811671966,36.4505507335666,-12.0262106973134));
#8573=CARTESIAN_POINT('Ctrl Pts',(2.19584925314808,36.4616980397613,-11.9782081635445));
#8574=CARTESIAN_POINT('Ctrl Pts',(2.47412713324821,36.4728453459559,-11.9204507120547));
#8575=CARTESIAN_POINT('Ctrl Pts',(2.75235774788912,36.4839907587822,-11.8627030706599));
#8576=CARTESIAN_POINT('Ctrl Pts',(3.02859552104343,36.4951361716085,-11.7952038736759));
#8577=CARTESIAN_POINT('Ctrl Pts',(3.30215083685498,36.5062815844348,-11.7181163204953));
#8578=CARTESIAN_POINT('Ctrl Pts',(3.57567578378372,36.5174257599474,-11.6410373252286));
#8579=CARTESIAN_POINT('Ctrl Pts',(3.84651861133585,36.52856993546,-11.5543721716479));
#8580=CARTESIAN_POINT('Ctrl Pts',(4.11400354010584,36.5397141109726,-11.4583343083538));
#8581=CARTESIAN_POINT('Ctrl Pts',(4.38991211491443,36.5512092393046,-11.3592720168407));
#8582=CARTESIAN_POINT('Ctrl Pts',(4.66224758709874,36.5627043676366,-11.250237209273));
#8583=CARTESIAN_POINT('Ctrl Pts',(4.93028776824498,36.5741994959687,-11.1315188888262));
#8584=CARTESIAN_POINT('Ctrl Pts',(5.19015841733053,36.5853442670556,-11.0164189554471));
#8585=CARTESIAN_POINT('Ctrl Pts',(5.44599147331901,36.5964890381425,-10.8922171642219));
#8586=CARTESIAN_POINT('Ctrl Pts',(5.69715035220492,36.6076338092294,-10.7592252562334));
#8587=CARTESIAN_POINT('Ctrl Pts',(5.96015272238509,36.619304116184,-10.6199620648587));
#8588=CARTESIAN_POINT('Ctrl Pts',(6.21802920235262,36.6309744231386,-10.4710599556509));
#8589=CARTESIAN_POINT('Ctrl Pts',(6.47007809708769,36.6426447300932,-10.3129307021615));
#8590=CARTESIAN_POINT('Ctrl Pts',(6.72212699182275,36.6543150370478,-10.1548014486722));
#8591=CARTESIAN_POINT('Ctrl Pts',(6.96834802179005,36.6659853440024,-9.98744523663738));
#8592=CARTESIAN_POINT('Ctrl Pts',(7.20807366931145,36.677655650957,-9.81132632358027));
#8593=CARTESIAN_POINT('Ctrl Pts',(7.43705609365123,36.6888029570834,-9.64310011958052));
#8594=CARTESIAN_POINT('Ctrl Pts',(7.66018090385868,36.6999502632097,-9.46682910328908));
#8595=CARTESIAN_POINT('Ctrl Pts',(7.8768873622909,36.711097569336,-9.2829465005343));
#8596=CARTESIAN_POINT('Ctrl Pts',(8.0935570131396,36.7222429820928,-9.09909513023244));
#8597=CARTESIAN_POINT('Ctrl Pts',(8.3038102853956,36.7333883948497,-8.90763492711705));
#8598=CARTESIAN_POINT('Ctrl Pts',(8.50711974988999,36.7445338076065,-8.70903920137186));
#8599=CARTESIAN_POINT('Ctrl Pts',(8.71040664386375,36.7556779830487,-8.51046552284879));
#8600=CARTESIAN_POINT('Ctrl Pts',(8.9067510786137,36.7668221584909,-8.30475808984803));
#8601=CARTESIAN_POINT('Ctrl Pts',(9.09566182065551,36.7779663339332,-8.09242771325575));
#8602=CARTESIAN_POINT('Ctrl Pts',(9.29052174942825,36.7894614623172,-7.87341061760588));
#8603=CARTESIAN_POINT('Ctrl Pts',(9.47747198957374,36.8009565907013,-7.64734689392032));
#8604=CARTESIAN_POINT('Ctrl Pts',(9.65601671358983,36.8124517190854,-7.41483590357021));
#8605=CARTESIAN_POINT('Ctrl Pts',(9.82911961410876,36.8235964901005,-7.18941156211219));
#8606=CARTESIAN_POINT('Ctrl Pts',(9.99432162080455,36.8347412611157,-6.95792736516624));
#8607=CARTESIAN_POINT('Ctrl Pts',(10.1512129534238,36.8458860321308,-6.72096167406424));
#8608=CARTESIAN_POINT('Ctrl Pts',(10.3155025584388,36.8575563391994,-6.47282177274978));
#8609=CARTESIAN_POINT('Ctrl Pts',(10.4706786683875,36.8692266462679,-6.21867123920136));
#8610=CARTESIAN_POINT('Ctrl Pts',(10.616322201149,36.8808969533365,-5.95920742812246));
#8611=CARTESIAN_POINT('Ctrl Pts',(10.7619657339106,36.892567260405,-5.69974361704354));
#8612=CARTESIAN_POINT('Ctrl Pts',(10.8980765329177,36.9042375674736,-5.43496682529208));
#8613=CARTESIAN_POINT('Ctrl Pts',(11.0242906417777,36.9159078745421,-5.16560413655685));
#8614=CARTESIAN_POINT('Ctrl Pts',(11.1448485153909,36.9270551814265,-4.90831282991925));
#8615=CARTESIAN_POINT('Ctrl Pts',(11.2564132397565,36.9382024883108,-4.64676077901756));
#8616=CARTESIAN_POINT('Ctrl Pts',(11.3586997682256,36.9493497951952,-4.38159672098112));
#8617=CARTESIAN_POINT('Ctrl Pts',(11.4609689233679,36.9604952087139,-4.11647770095597));
#8618=CARTESIAN_POINT('Ctrl Pts',(11.5539629329279,36.9716406222325,-3.84774814742302));
#8619=CARTESIAN_POINT('Ctrl Pts',(11.6374451793146,36.9827860357512,-3.57607605462302));
#8620=CARTESIAN_POINT('Ctrl Pts',(11.7209181578842,36.993930211957,-3.30443412161603));
#8621=CARTESIAN_POINT('Ctrl Pts',(11.7948814035168,37.0050743881628,-3.0298505565593));
#8622=CARTESIAN_POINT('Ctrl Pts',(11.8591480264475,37.0162185643687,-2.75300896053869));
#8623=CARTESIAN_POINT('Ctrl Pts',(11.9254385293134,37.0277136921819,-2.46744908859368));
#8624=CARTESIAN_POINT('Ctrl Pts',(11.9814117057185,37.0392088199951,-2.17948694843925));
#8625=CARTESIAN_POINT('Ctrl Pts',(12.0269190072912,37.0507039478083,-1.88988609234979));
#8626=CARTESIAN_POINT('Ctrl Pts',(12.0710393075008,37.061848719582,-1.60911188095882));
#8627=CARTESIAN_POINT('Ctrl Pts',(12.1053222141113,37.0729934913558,-1.32679764185019));
#8628=CARTESIAN_POINT('Ctrl Pts',(12.129684684297,37.0841382631295,-1.04364731089197));
#8629=CARTESIAN_POINT('Ctrl Pts',(12.1551959718931,37.0958085689624,-0.747144966467611));
#8630=CARTESIAN_POINT('Ctrl Pts',(12.1698286831205,37.1074788747954,-0.44972609738708));
#8631=CARTESIAN_POINT('Ctrl Pts',(12.1735485509352,37.1191491806283,-0.152203574280096));
#8632=CARTESIAN_POINT('Ctrl Pts',(12.1772684187499,37.1308194864613,0.145318948826918));
#8633=CARTESIAN_POINT('Ctrl Pts',(12.170075447735,37.1424897922942,0.442944790376295));
#8634=CARTESIAN_POINT('Ctrl Pts',(12.1519980013252,37.1541600981272,0.73986135578836));
#8635=CARTESIAN_POINT('Ctrl Pts',(12.134730690394,37.1653074026142,1.02347169207873));
#8636=CARTESIAN_POINT('Ctrl Pts',(12.1075278724749,37.1764547071013,1.30651963043172));
#8637=CARTESIAN_POINT('Ctrl Pts',(12.0704497066061,37.1876020115883,1.58829913123846));
#8638=CARTESIAN_POINT('Ctrl Pts',(12.0333778384804,37.1987474227007,1.87003077167098));
#8639=CARTESIAN_POINT('Ctrl Pts',(11.9864340059855,37.2098928338131,2.15049414032514));
#8640=CARTESIAN_POINT('Ctrl Pts',(11.9297301073365,37.2210382449255,2.4289894639765));
#8641=CARTESIAN_POINT('Ctrl Pts',(11.8730325037096,37.2321824187225,2.70745387027918));
#8642=CARTESIAN_POINT('Ctrl Pts',(11.806577050753,37.2433265925194,2.98395040653923));
#8643=CARTESIAN_POINT('Ctrl Pts',(11.730526779452,37.2544707663164,3.25778939260328));
#8644=CARTESIAN_POINT('Ctrl Pts',(11.6520815091351,37.2659658959327,3.5402522019744));
#8645=CARTESIAN_POINT('Ctrl Pts',(11.563427371625,37.277461025549,3.81988707545358));
#8646=CARTESIAN_POINT('Ctrl Pts',(11.4647993244373,37.2889561551654,4.09595247779841));
#8647=CARTESIAN_POINT('Ctrl Pts',(11.3691773629799,37.3001009245536,4.36360367860211));
#8648=CARTESIAN_POINT('Ctrl Pts',(11.2641805724472,37.3112456939418,4.6278995113326));
#8649=CARTESIAN_POINT('Ctrl Pts',(11.1500728991938,37.3223904633301,4.88818213579082));
#8650=CARTESIAN_POINT('Ctrl Pts',(11.0305843891053,37.3340607730604,5.16073859156343));
#8651=CARTESIAN_POINT('Ctrl Pts',(10.9011051867154,37.3457310827908,5.4288939487069));
#8652=CARTESIAN_POINT('Ctrl Pts',(10.7619941971752,37.3574013925212,5.6919180554509));
#8653=CARTESIAN_POINT('Ctrl Pts',(10.622883207635,37.3690717022515,5.95494216219492));
#8654=CARTESIAN_POINT('Ctrl Pts',(10.4741405955607,37.3807420119819,6.21283472606724));
#8655=CARTESIAN_POINT('Ctrl Pts',(10.3161801276997,37.3924123217123,6.46489580912594));
#8656=CARTESIAN_POINT('Ctrl Pts',(10.1652985893882,37.4035596315964,6.70566088456128));
#8657=CARTESIAN_POINT('Ctrl Pts',(10.0059621610874,37.4147069414806,6.94117756831538));
#8658=CARTESIAN_POINT('Ctrl Pts',(9.83856153689548,37.4258542513647,7.17085470043292));
#8659=CARTESIAN_POINT('Ctrl Pts',(9.67118934551754,37.4369996678904,7.40049282213932));
#8660=CARTESIAN_POINT('Ctrl Pts',(9.49575584989997,37.448145084416,7.62429315693641));
#8661=CARTESIAN_POINT('Ctrl Pts',(9.31269417572409,37.4592905009417,7.84169480657305));
#8662=CARTESIAN_POINT('Ctrl Pts',(9.12965282422266,37.4704346801539,8.05907232126735));
#8663=CARTESIAN_POINT('Ctrl Pts',(8.93898515694895,37.4815788593662,8.27005236527153));
#8664=CARTESIAN_POINT('Ctrl Pts',(8.74116436747306,37.4927230385784,8.47410737191944));
#8665=CARTESIAN_POINT('Ctrl Pts',(8.53711391475835,37.5042181641383,8.68458836633626));
#8666=CARTESIAN_POINT('Ctrl Pts',(8.32545271468949,37.5157132896982,8.88770087711788));
#8667=CARTESIAN_POINT('Ctrl Pts',(8.10674193044595,37.5272084152581,9.08290622670682));
#8668=CARTESIAN_POINT('Ctrl Pts',(7.89469705879945,37.5383531899996,9.27216206720623));
#8669=CARTESIAN_POINT('Ctrl Pts',(7.67602616543322,37.549497964741,9.45398541568647));
#8670=CARTESIAN_POINT('Ctrl Pts',(7.45127581728952,37.5606427394824,9.62792495528899));
#8671=CARTESIAN_POINT('Ctrl Pts',(7.21592747991899,37.5723130404516,9.81006652608769));
#8672=CARTESIAN_POINT('Ctrl Pts',(6.9739127963806,37.5839833414207,9.98356268944996));
#8673=CARTESIAN_POINT('Ctrl Pts',(6.72589631532788,37.5956536423899,10.1479440777657));
#8674=CARTESIAN_POINT('Ctrl Pts',(6.47787983427515,37.6073239433591,10.3123254660813));
#8675=CARTESIAN_POINT('Ctrl Pts',(6.22386184020968,37.6189942443282,10.4675919013181));
#8676=CARTESIAN_POINT('Ctrl Pts',(5.96454059505376,37.6306645452974,10.6133267988862));
#8677=CARTESIAN_POINT('Ctrl Pts',(5.71684316802239,37.6418117365775,10.7525292739267));
#8678=CARTESIAN_POINT('Ctrl Pts',(5.46423348683355,37.6529589278576,10.8830774824776));
#8679=CARTESIAN_POINT('Ctrl Pts',(5.20733748166243,37.6641061191377,11.0046393217621));
#8680=CARTESIAN_POINT('Ctrl Pts',(4.95048636431727,37.6752513626523,11.1261799203634));
#8681=CARTESIAN_POINT('Ctrl Pts',(4.68935065937322,37.6863966061668,11.2387371707387));
#8682=CARTESIAN_POINT('Ctrl Pts',(4.42457906275146,37.6975418496814,11.3420258493561));
#8683=CARTESIAN_POINT('Ctrl Pts',(4.15982285196366,37.7086864455477,11.4453085258853));
#8684=CARTESIAN_POINT('Ctrl Pts',(3.89143141911817,37.719831041414,11.5393236073228));
#8685=CARTESIAN_POINT('Ctrl Pts',(3.62007279718327,37.7309756372803,11.6238342724375));
#8686=CARTESIAN_POINT('Ctrl Pts',(3.34873426985421,37.7421194078688,11.7083386793819));
#8687=CARTESIAN_POINT('Ctrl Pts',(3.07442924725578,37.7532631784572,11.7833399974053));
#8688=CARTESIAN_POINT('Ctrl Pts',(2.79784129946167,37.7644069490457,11.8486511600699));
#8689=CARTESIAN_POINT('Ctrl Pts',(2.52123406790476,37.7755514965798,11.9139668762409));
#8690=CARTESIAN_POINT('Ctrl Pts',(2.24234385257215,37.786696044114,11.9695910250927));
#8691=CARTESIAN_POINT('Ctrl Pts',(1.96186619748412,37.7978405916482,12.0153872710441));
#8692=CARTESIAN_POINT('Ctrl Pts',(1.83845955010879,37.8027440526647,12.035537044378));
#8693=CARTESIAN_POINT('Ctrl Pts',(1.71474572240879,37.8076475136811,12.0537849101436));
#8694=CARTESIAN_POINT('Ctrl Pts',(1.59078448392769,37.8125509746976,12.0701224093087));
#8695=CARTESIAN_POINT('Origin',(0.,20.,0.));
#8696=CARTESIAN_POINT('',(-9.83900047314216,22.8294636018362,-3.67173622267202));
#8697=CARTESIAN_POINT('',(-9.83826089695889,22.011121265682,-3.67146067980712));
#8698=CARTESIAN_POINT('',(-9.83826089695937,20.,-3.67146067980583));
#8699=CARTESIAN_POINT('',(-10.5009999965284,22.6589303284762,0.000270018945713324));
#8700=CARTESIAN_POINT('Ctrl Pts',(-10.5010864010386,22.6589303319738,0.000269944245985663));
#8701=CARTESIAN_POINT('Ctrl Pts',(-10.4997937395166,22.7157747552614,-1.24986959862917));
#8702=CARTESIAN_POINT('Ctrl Pts',(-10.2752983162086,22.7726191785488,-2.50045949815336));
#8703=CARTESIAN_POINT('Ctrl Pts',(-9.8390004731412,22.8294636018363,-3.6717362226746));
#8704=CARTESIAN_POINT('',(-7.93387242656103,20.0000000365693,-6.87929279207206));
#8705=CARTESIAN_POINT('Ctrl Pts',(-7.93387242656103,20.0000000365693,-6.87929279207206));
#8706=CARTESIAN_POINT('Ctrl Pts',(-7.76761933943708,20.0115427600485,-7.07103209197269));
#8707=CARTESIAN_POINT('Ctrl Pts',(-7.59438520903055,20.0230854835278,-7.25677295860134));
#8708=CARTESIAN_POINT('Ctrl Pts',(-7.41462834869705,20.034628207007,-7.4360128732203));
#8709=CARTESIAN_POINT('Ctrl Pts',(-7.23490292970705,20.0461689115439,-7.61522143691495));
#8710=CARTESIAN_POINT('Ctrl Pts',(-7.04865725581925,20.0577096160809,-7.78793112142728));
#8711=CARTESIAN_POINT('Ctrl Pts',(-6.85638681915036,20.0692503206178,-7.95367592916516));
#8712=CARTESIAN_POINT('Ctrl Pts',(-6.66413668086264,20.080789806779,-8.11940323888648));
#8713=CARTESIAN_POINT('Ctrl Pts',(-6.46586326115029,20.0923292929403,-8.27816695779237));
#8714=CARTESIAN_POINT('Ctrl Pts',(-6.26209628867734,20.1038687791016,-8.42954038316049));
#8715=CARTESIAN_POINT('Ctrl Pts',(-6.05831348529575,20.1154091617798,-8.58092556891764));
#8716=CARTESIAN_POINT('Ctrl Pts',(-5.84903649881054,20.126949544458,-8.72491914519595));
#8717=CARTESIAN_POINT('Ctrl Pts',(-5.63482633728949,20.1384899271363,-8.86113610935916));
#8718=CARTESIAN_POINT('Ctrl Pts',(-5.42061577914819,20.1500303311821,-8.99735332573452));
#8719=CARTESIAN_POINT('Ctrl Pts',(-5.20147226469043,20.1615707352279,-9.12579375361984));
#8720=CARTESIAN_POINT('Ctrl Pts',(-4.97798450545638,20.1731111392737,-9.24611655039218));
#8721=CARTESIAN_POINT('Ctrl Pts',(-4.75444854472634,20.1846540323361,-9.36646529820017));
#8722=CARTESIAN_POINT('Ctrl Pts',(-4.52656671290687,20.1961969253985,-9.47869278418477));
#8723=CARTESIAN_POINT('Ctrl Pts',(-4.29495217795627,20.2077398184608,-9.58250420240288));
#8724=CARTESIAN_POINT('Ctrl Pts',(-4.17906943469033,20.2135150264528,-9.63444374034253));
#8725=CARTESIAN_POINT('Ctrl Pts',(-4.06225265218799,20.2192902344447,-9.6842772535272));
#8726=CARTESIAN_POINT('Ctrl Pts',(-3.94458058590528,20.2250654424367,-9.73197230787774));
#8727=CARTESIAN_POINT('Ctrl Pts',(-3.70889539637858,20.236632597099,-9.8275006544021));
#8728=CARTESIAN_POINT('Ctrl Pts',(-3.46970190359019,20.2481997517614,-9.91447815568018));
#8729=CARTESIAN_POINT('Ctrl Pts',(-3.227639342775,20.2597669064238,-9.99266457322425));
#8730=CARTESIAN_POINT('Ctrl Pts',(-2.98561909575511,20.2713320390874,-10.0708373233757));
#8731=CARTESIAN_POINT('Ctrl Pts',(-2.74073104518588,20.282897171751,-10.1402219724847));
#8732=CARTESIAN_POINT('Ctrl Pts',(-2.49363094408252,20.2944623044145,-10.2006277117986));
#8733=CARTESIAN_POINT('Ctrl Pts',(-2.24655838679567,20.306026147933,-10.2610267177903));
#8734=CARTESIAN_POINT('Ctrl Pts',(-1.99727454010465,20.3175899914514,-10.3124487466889));
#8735=CARTESIAN_POINT('Ctrl Pts',(-1.74644781609206,20.3291538349698,-10.3547535473167));
#8736=CARTESIAN_POINT('Ctrl Pts',(-1.49560122773008,20.3407185942927,-10.3970616982946));
#8737=CARTESIAN_POINT('Ctrl Pts',(-1.24321179031955,20.3522833536156,-10.4302511288727));
#8738=CARTESIAN_POINT('Ctrl Pts',(-0.989956899476713,20.3638481129385,-10.4542329387277));
#8739=CARTESIAN_POINT('Ctrl Pts',(-0.736706570407378,20.3754126639502,-10.4782143166084));
#8740=CARTESIAN_POINT('Ctrl Pts',(-0.482591094877707,20.386977214962,-10.4929883812208));
#8741=CARTESIAN_POINT('Ctrl Pts',(-0.228292540303652,20.3985417659737,-10.4985181581041));
#8742=CARTESIAN_POINT('Ctrl Pts',(0.0260656621990141,20.4101090295511,-10.5040492320444));
#8743=CARTESIAN_POINT('Ctrl Pts',(0.280606752688652,20.4216762931284,-10.5003316777243));
#8744=CARTESIAN_POINT('Ctrl Pts',(0.534647621022751,20.4332435567058,-10.4873806511128));
#8745=CARTESIAN_POINT('Ctrl Pts',(0.754810692836675,20.4432682598111,-10.4761567176542));
#8746=CARTESIAN_POINT('Ctrl Pts',(0.974597946320386,20.4532929629165,-10.4579986016713));
#8747=CARTESIAN_POINT('Ctrl Pts',(1.19356681527101,20.4633176660218,-10.4329477741185));
#8748=CARTESIAN_POINT('Ctrl Pts',(1.44621574302689,20.4748842896372,-10.4040438264891));
#8749=CARTESIAN_POINT('Ctrl Pts',(1.69785355141683,20.4864509132526,-10.3659536780285));
#8750=CARTESIAN_POINT('Ctrl Pts',(1.94780404330222,20.4980175368679,-10.3187722335991));
#8751=CARTESIAN_POINT('Ctrl Pts',(2.19771061531791,20.5095821280624,-10.271599079623));
#8752=CARTESIAN_POINT('Ctrl Pts',(2.44593019076294,20.5211467192569,-10.2153378699943));
#8753=CARTESIAN_POINT('Ctrl Pts',(2.69179571929448,20.5327113104513,-10.1501348171139));
#8754=CARTESIAN_POINT('Ctrl Pts',(2.93763365212993,20.5442746036479,-10.0849390825577));
#8755=CARTESIAN_POINT('Ctrl Pts',(3.18111779808646,20.5558378968444,-10.0108035796106));
#8756=CARTESIAN_POINT('Ctrl Pts',(3.42159418211181,20.567401190041,-9.92792497216506));
#8757=CARTESIAN_POINT('Ctrl Pts',(3.66208940860482,20.5789653892765,-9.84503987078675));
#8758=CARTESIAN_POINT('Ctrl Pts',(3.89957613936932,20.5905295885121,-9.7534103830688));
#8759=CARTESIAN_POINT('Ctrl Pts',(4.13341708260761,20.6020937877476,-9.65328256196863));
#8760=CARTESIAN_POINT('Ctrl Pts',(4.36725372089671,20.6136577740893,-9.55315658419485));
#8761=CARTESIAN_POINT('Ctrl Pts',(4.59744445206855,20.6252217604311,-9.44453269662927));
#8762=CARTESIAN_POINT('Ctrl Pts',(4.82337272867542,20.6367857467728,-9.32770478307875));
#8763=CARTESIAN_POINT('Ctrl Pts',(5.049353932526,20.6483524421598,-9.21084950075641));
#8764=CARTESIAN_POINT('Ctrl Pts',(5.27107043963594,20.6599191375467,-9.08578647774354));
#8765=CARTESIAN_POINT('Ctrl Pts',(5.48792973200312,20.6714858329337,-8.95285587154156));
#8766=CARTESIAN_POINT('Ctrl Pts',(5.67594100123841,20.6815138518248,-8.83760855278735));
#8767=CARTESIAN_POINT('Ctrl Pts',(5.86030167021098,20.6915418707158,-8.71644839631923));
#8768=CARTESIAN_POINT('Ctrl Pts',(6.04064259344008,20.7015698896069,-8.58962386011853));
#8769=CARTESIAN_POINT('Ctrl Pts',(6.24866971656362,20.7131374244913,-8.44332903731897));
#8770=CARTESIAN_POINT('Ctrl Pts',(6.45141193053673,20.7247049593757,-8.2894509307573));
#8771=CARTESIAN_POINT('Ctrl Pts',(6.64832085415769,20.7362724942601,-8.1283965712908));
#8772=CARTESIAN_POINT('Ctrl Pts',(6.84519539190618,20.7478380091254,-7.96737033647484));
#8773=CARTESIAN_POINT('Ctrl Pts',(7.03623845868885,20.7594035239908,-7.79917052559365));
#8774=CARTESIAN_POINT('Ctrl Pts',(7.22093426151812,20.7709690388561,-7.624244840693));
#8775=CARTESIAN_POINT('Ctrl Pts',(7.4056094914013,20.7825332654588,-7.4493386404619));
#8776=CARTESIAN_POINT('Ctrl Pts',(7.58393866813121,20.7940974920614,-7.26770825235433));
#8777=CARTESIAN_POINT('Ctrl Pts',(7.75544162581868,20.805661718664,-7.07983941827206));
#8778=CARTESIAN_POINT('Ctrl Pts',(7.92695814427787,20.8172268596523,-6.89195572936509));
#8779=CARTESIAN_POINT('Ctrl Pts',(8.09164717607218,20.8287920006405,-6.69783281100001));
#8780=CARTESIAN_POINT('Ctrl Pts',(8.24906684102578,20.8403571416288,-6.49799178610508));
#8781=CARTESIAN_POINT('Ctrl Pts',(8.40648365211932,20.8519220729527,-6.29815438412675));
#8782=CARTESIAN_POINT('Ctrl Pts',(8.55663119010718,20.8634870042766,-6.09259930154301));
#8783=CARTESIAN_POINT('Ctrl Pts',(8.69910868029778,20.8750519356005,-5.88187973086563));
#8784=CARTESIAN_POINT('Ctrl Pts',(8.84161952783095,20.8866195745477,-5.67111082576427));
#8785=CARTESIAN_POINT('Ctrl Pts',(8.97645658274871,20.8981872134949,-5.45517524491679));
#8786=CARTESIAN_POINT('Ctrl Pts',(9.10326231471628,20.9097548524421,-5.23465531142849));
#8787=CARTESIAN_POINT('Ctrl Pts',(9.21312918916514,20.9197772726921,-5.04359268775918));
#8788=CARTESIAN_POINT('Ctrl Pts',(9.31696772742072,20.929799692942,-4.84908921829048));
#8789=CARTESIAN_POINT('Ctrl Pts',(9.41457305225478,20.939822113192,-4.65153901883646));
#8790=CARTESIAN_POINT('Ctrl Pts',(9.52721930290881,20.9513889827819,-4.42354644443252));
#8791=CARTESIAN_POINT('Ctrl Pts',(9.63159720442441,20.9629558523718,-4.19142462929393));
#8792=CARTESIAN_POINT('Ctrl Pts',(9.7274200224257,20.9745227219618,-3.9557933094781));
#8793=CARTESIAN_POINT('Ctrl Pts',(9.82322603763168,20.9860875632692,-3.72020330826378));
#8794=CARTESIAN_POINT('Ctrl Pts',(9.91047985981083,20.9976524045767,-3.48110528720773));
#8795=CARTESIAN_POINT('Ctrl Pts',(9.98894283068399,21.0092172458841,-3.23913910249729));
#8796=CARTESIAN_POINT('Ctrl Pts',(10.0673970183146,21.0207807926089,-2.99720000378267));
#8797=CARTESIAN_POINT('Ctrl Pts',(10.1370622341291,21.0323443393336,-2.75239364572893));
#8798=CARTESIAN_POINT('Ctrl Pts',(10.1977493055541,21.0439078860583,-2.50537623942409));
#8799=CARTESIAN_POINT('Ctrl Pts',(10.2584411501937,21.0554723422896,-2.25833940448208));
#8800=CARTESIAN_POINT('Ctrl Pts',(10.3101533700907,21.0670367985209,-2.00909144186784));
#8801=CARTESIAN_POINT('Ctrl Pts',(10.3527473408365,21.0786012547522,-1.75830131001571));
#8802=CARTESIAN_POINT('Ctrl Pts',(10.3953405331328,21.0901654996309,-1.50751576161625));
#8803=CARTESIAN_POINT('Ctrl Pts',(10.428815765027,21.1017297445096,-1.25518837362866));
#8804=CARTESIAN_POINT('Ctrl Pts',(10.453085851784,21.1132939893884,-1.00199659442159));
#8805=CARTESIAN_POINT('Ctrl Pts',(10.4773616255209,21.1248609440072,-0.748745487179122));
#8806=CARTESIAN_POINT('Ctrl Pts',(10.492427915911,21.1364278986261,-0.494629859558551));
#8807=CARTESIAN_POINT('Ctrl Pts',(10.4982494496924,21.147994853245,-0.240332045374405));
#8808=CARTESIAN_POINT('Ctrl Pts',(10.5032956851473,21.1580213477557,-0.0199010225155619));
#8809=CARTESIAN_POINT('Ctrl Pts',(10.5013963984425,21.1680478422664,0.200666716014741));
#8810=CARTESIAN_POINT('Ctrl Pts',(10.4925603111451,21.1780743367771,0.420926498313265));
#8811=CARTESIAN_POINT('Ctrl Pts',(10.4823664180197,21.1896415621819,0.675032711280474));
#8812=CARTESIAN_POINT('Ctrl Pts',(10.4629357848001,21.2012087875866,0.928807784217113));
#8813=CARTESIAN_POINT('Ctrl Pts',(10.4343132327989,21.2127760129914,1.18157029407343));
#8814=CARTESIAN_POINT('Ctrl Pts',(10.405695689421,21.2243412142624,1.4342885733465));
#8815=CARTESIAN_POINT('Ctrl Pts',(10.3678894693691,21.2359064155334,1.6859943683356));
#8816=CARTESIAN_POINT('Ctrl Pts',(10.3209912360567,21.2474716168044,1.9360115973934));
#8817=CARTESIAN_POINT('Ctrl Pts',(10.2740982398118,21.2590355266038,2.18600090733733));
#8818=CARTESIAN_POINT('Ctrl Pts',(10.2181153085458,21.2705994364031,2.43430175588062));
#8819=CARTESIAN_POINT('Ctrl Pts',(10.1531903835915,21.2821633462024,2.68024738308711));
#8820=CARTESIAN_POINT('Ctrl Pts',(10.0882603399369,21.2937281677038,2.92621240071936));
#8821=CARTESIAN_POINT('Ctrl Pts',(10.0143869613077,21.3052929892052,3.16982155745538));
#8822=CARTESIAN_POINT('Ctrl Pts',(9.93176867348247,21.3168578107066,3.4104210907793));
#8823=CARTESIAN_POINT('Ctrl Pts',(9.84915189072215,21.3284224215306,3.65101624107944));
#8824=CARTESIAN_POINT('Ctrl Pts',(9.75779060903818,21.3399870323546,3.88860161638269));
#8825=CARTESIAN_POINT('Ctrl Pts',(9.65793248410276,21.3515516431785,4.12254061623566));
#8826=CARTESIAN_POINT('Ctrl Pts',(9.55805097403558,21.3631189622443,4.35653440075777));
#8827=CARTESIAN_POINT('Ctrl Pts',(9.44966875177061,21.3746862813101,4.58687984810717));
#8828=CARTESIAN_POINT('Ctrl Pts',(9.33308139224463,21.3862536003759,4.81296091047258));
#8829=CARTESIAN_POINT('Ctrl Pts',(9.23204596712439,21.3962779203713,5.00888434797557));
#8830=CARTESIAN_POINT('Ctrl Pts',(9.12484921800875,21.4063022403668,5.20160543394834));
#8831=CARTESIAN_POINT('Ctrl Pts',(9.01171144400528,21.4163265603622,5.3907381544631));
#8832=CARTESIAN_POINT('Ctrl Pts',(8.88116158188506,21.4278936395697,5.60897870942459));
#8833=CARTESIAN_POINT('Ctrl Pts',(8.74265991882837,21.4394607187771,5.82250848322717));
#8834=CARTESIAN_POINT('Ctrl Pts',(8.59657188523117,21.4510277979846,6.0307506018781));
#8835=CARTESIAN_POINT('Ctrl Pts',(8.45050943566692,21.4625928514783,6.23895625160618));
#8836=CARTESIAN_POINT('Ctrl Pts',(8.29686342668251,21.474157904972,6.44187586825196));
#8837=CARTESIAN_POINT('Ctrl Pts',(8.1360422536485,21.4857229584658,6.63896207602109));
#8838=CARTESIAN_POINT('Ctrl Pts',(7.97523905559414,21.4972867193337,6.83602625546828));
#8839=CARTESIAN_POINT('Ctrl Pts',(7.80726246971827,21.5088504802016,7.02725811347687));
#8840=CARTESIAN_POINT('Ctrl Pts',(7.63256145618762,21.5204142410695,7.21214299757839));
#8841=CARTESIAN_POINT('Ctrl Pts',(7.45784667973596,21.5319789129288,7.39704244688481));
#8842=CARTESIAN_POINT('Ctrl Pts',(7.27640660479359,21.5435435847882,7.57559371963131));
#8843=CARTESIAN_POINT('Ctrl Pts',(7.08872830055373,21.5551082566475,7.74731773460523));
#8844=CARTESIAN_POINT('Ctrl Pts',(6.90105341809982,21.5666727176576,7.91903861867477));
#8845=CARTESIAN_POINT('Ctrl Pts',(6.70714073932691,21.5782371786677,8.08393230839132));
#8846=CARTESIAN_POINT('Ctrl Pts',(6.50751234785372,21.5898016396778,8.24155835036866));
#8847=CARTESIAN_POINT('Ctrl Pts',(6.30783719252306,21.6013688097154,8.39922131696232));
#8848=CARTESIAN_POINT('Ctrl Pts',(6.10244386533014,21.612935979753,8.54961306089783));
#8849=CARTESIAN_POINT('Ctrl Pts',(5.89188669093872,21.6245031497906,8.69233410662172));
#8850=CARTESIAN_POINT('Ctrl Pts',(5.70939778698386,21.6345283611761,8.8160297597417));
#8851=CARTESIAN_POINT('Ctrl Pts',(5.52303059208186,21.6445535725617,8.93396407346112));
#8852=CARTESIAN_POINT('Ctrl Pts',(5.3331633740482,21.6545787839473,9.04590346099885));
#8853=CARTESIAN_POINT('Ctrl Pts',(5.11409401130845,21.6661459027596,9.17505946037215));
#8854=CARTESIAN_POINT('Ctrl Pts',(4.89029674129765,21.677713021572,9.29627375453589));
#8855=CARTESIAN_POINT('Ctrl Pts',(4.66236849914987,21.6892801403843,9.40921468445348));
#8856=CARTESIAN_POINT('Ctrl Pts',(4.4344801664234,21.7008452338355,9.52213583881753));
#8857=CARTESIAN_POINT('Ctrl Pts',(4.20246255342235,21.7124103272867,9.62678639796797));
#8858=CARTESIAN_POINT('Ctrl Pts',(3.96693620500328,21.7239754207378,9.72288116483145));
#8859=CARTESIAN_POINT('Ctrl Pts',(3.73143617643087,21.7355392218007,9.81896519319563));
#8860=CARTESIAN_POINT('Ctrl Pts',(3.49242845155076,21.7471030228636,9.90649523377258));
#8861=CARTESIAN_POINT('Ctrl Pts',(3.25055353409967,21.7586668239265,9.98523423470637));
#8862=CARTESIAN_POINT('Ctrl Pts',(3.00865956023713,21.7702315360576,10.0639794391887));
#8863=CARTESIAN_POINT('Ctrl Pts',(2.76389820463271,21.7817962481888,10.1339321311693));
#8864=CARTESIAN_POINT('Ctrl Pts',(2.51692641074983,21.7933609603199,10.1949047294651));
#8865=CARTESIAN_POINT('Ctrl Pts',(2.26995912005407,21.8049254615846,10.2558762160104));
#8866=CARTESIAN_POINT('Ctrl Pts',(2.02078174091657,21.8164899628492,10.3078678717852));
#8867=CARTESIAN_POINT('Ctrl Pts',(1.77006347660718,21.8280544641139,10.3507427892293));
#8868=CARTESIAN_POINT('Ctrl Pts',(1.51928648744899,21.8396216740907,10.3936277491129));
#8869=CARTESIAN_POINT('Ctrl Pts',(1.26696816464985,21.8511888840674,10.4273916553262));
#8870=CARTESIAN_POINT('Ctrl Pts',(1.01378641150786,21.8627560940442,10.451949010201));
#8871=CARTESIAN_POINT('Ctrl Pts',(0.794361003023756,21.8727810652069,10.4732321696619));
#8872=CARTESIAN_POINT('Ctrl Pts',(0.574287290355624,21.8828060363696,10.4876009062648));
#8873=CARTESIAN_POINT('Ctrl Pts',(0.354009164658848,21.8928310075323,10.4950311343672));
#8874=CARTESIAN_POINT('Ctrl Pts',(0.0998454799983954,21.9043981279682,10.5036043603578));
#8875=CARTESIAN_POINT('Ctrl Pts',(-0.154669164764553,21.9159652484041,10.5029417501122));
#8876=CARTESIAN_POINT('Ctrl Pts',(-0.408851908986821,21.92753236884,10.4930377449296));
#8877=CARTESIAN_POINT('Ctrl Pts',(-0.662990148560078,21.9390974639982,10.4831354738312));
#8878=CARTESIAN_POINT('Ctrl Pts',(-0.916796327124914,21.9506625591565,10.4639950486802));
#8879=CARTESIAN_POINT('Ctrl Pts',(-1.16958908724468,21.9622276543147,10.4356630056263));
#8880=CARTESIAN_POINT('Ctrl Pts',(-1.42235359973181,21.9737914571631,10.4073341284589));
#8881=CARTESIAN_POINT('Ctrl Pts',(-1.67410464488521,21.9853552600116,10.3698157149898));
#8882=CARTESIAN_POINT('Ctrl Pts',(-1.9241663796562,21.99691906286,10.323206127139));
#8883=CARTESIAN_POINT('Ctrl Pts',(-2.17424781820299,22.0084837768858,10.2765928666557));
#8884=CARTESIAN_POINT('Ctrl Pts',(-2.42263940761389,22.0200484909115,10.220887047828));
#8885=CARTESIAN_POINT('Ctrl Pts',(-2.66867454355026,22.0316132049373,10.1562383381155));
#8886=CARTESIAN_POINT('Ctrl Pts',(-2.91470519460546,22.0431777081542,10.0915908068597));
#8887=CARTESIAN_POINT('Ctrl Pts',(-3.15837921079943,22.0547422113712,10.0180007828975));
#8888=CARTESIAN_POINT('Ctrl Pts',(-3.39904347241097,22.0663067145882,9.93566829522103));
#8889=CARTESIAN_POINT('Ctrl Pts',(-3.6397641056346,22.0778739265982,9.85331652252478));
#8890=CARTESIAN_POINT('Ctrl Pts',(-3.87747331294342,22.0894411386083,9.76221828223451));
#8891=CARTESIAN_POINT('Ctrl Pts',(-4.11153493727735,22.1010083506183,9.66262290786243));
#8892=CARTESIAN_POINT('Ctrl Pts',(-4.31438921697679,22.1110333107847,9.57630654572003));
#8893=CARTESIAN_POINT('Ctrl Pts',(-4.51450390802682,22.1210582709511,9.48360864941968));
#8894=CARTESIAN_POINT('Ctrl Pts',(-4.71147772092378,22.1310832311175,9.38472049052282));
#8895=CARTESIAN_POINT('Ctrl Pts',(-4.93875220021531,22.1426503403095,9.27062027338817));
#8896=CARTESIAN_POINT('Ctrl Pts',(-5.16191511449861,22.1542174495014,9.14824246401068));
#8897=CARTESIAN_POINT('Ctrl Pts',(-5.38036420898964,22.1657845586934,9.01790895821328));
#8898=CARTESIAN_POINT('Ctrl Pts',(-5.59877505233851,22.1773496424472,8.88759827423379));
#8899=CARTESIAN_POINT('Ctrl Pts',(-5.81247348602248,22.1889147262009,8.74933481654849));
#8900=CARTESIAN_POINT('Ctrl Pts',(-6.02088350472526,22.2004798099547,8.60348550428995));
#8901=CARTESIAN_POINT('Ctrl Pts',(-6.22927023290093,22.2120436012711,8.45765249118719));
#8902=CARTESIAN_POINT('Ctrl Pts',(-6.43236949941675,22.2236073925875,8.30423547485258));
#8903=CARTESIAN_POINT('Ctrl Pts',(-6.62963494174465,22.2351711839039,8.14364424193484));
#8904=CARTESIAN_POINT('Ctrl Pts',(-6.82691592579408,22.2467358862832,7.98304035670358));
#8905=CARTESIAN_POINT('Ctrl Pts',(-7.01836195042591,22.2583005886625,7.81526129764087));
#8906=CARTESIAN_POINT('Ctrl Pts',(-7.20345931715591,22.2698652910418,7.64075747986283));
#8907=CARTESIAN_POINT('Ctrl Pts',(-7.38855330907376,22.2814297825661,7.46625684374865));
#8908=CARTESIAN_POINT('Ctrl Pts',(-7.56729867441535,22.2929942740905,7.28503188540077));
#8909=CARTESIAN_POINT('Ctrl Pts',(-7.73921765517788,22.3045587656148,7.09757078765566));
#8910=CARTESIAN_POINT('Ctrl Pts',(-7.91117690526097,22.3161259659396,6.91006578009324));
#8911=CARTESIAN_POINT('Ctrl Pts',(-8.07630638719474,22.3276931662644,6.71632191726792));
#8912=CARTESIAN_POINT('Ctrl Pts',(-8.23416683158492,22.3392603665892,6.51686255721469));
#8913=CARTESIAN_POINT('Ctrl Pts',(-8.37098088745965,22.3492853959603,6.34399566749777));
#8914=CARTESIAN_POINT('Ctrl Pts',(-8.50233549758968,22.3593104253315,6.16683632915167));
#8915=CARTESIAN_POINT('Ctrl Pts',(-8.6279698299386,22.3693354547026,5.98574453294403));
#8916=CARTESIAN_POINT('Ctrl Pts',(-8.7729297269788,22.3809025733261,5.776796487913));
#8917=CARTESIAN_POINT('Ctrl Pts',(-8.91031820995912,22.3924696919496,5.56254773761589));
#8918=CARTESIAN_POINT('Ctrl Pts',(-9.03976050121706,22.4040368105731,5.343569133139));
#8919=CARTESIAN_POINT('Ctrl Pts',(-9.16918012806939,22.4156019038781,5.12462887022624));
#8920=CARTESIAN_POINT('Ctrl Pts',(-9.29065619986459,22.4271669971831,4.9009606445605));
#8921=CARTESIAN_POINT('Ctrl Pts',(-9.40385853326217,22.4387320904881,4.67316227905604));
#8922=CARTESIAN_POINT('Ctrl Pts',(-9.51704821682695,22.4502958914479,4.44538936895653));
#8923=CARTESIAN_POINT('Ctrl Pts',(-9.62196588488816,22.4618596924076,4.2134874883438));
#8924=CARTESIAN_POINT('Ctrl Pts',(-9.71832789633379,22.4734234933674,3.97807791519226));
#8925=CARTESIAN_POINT('Ctrl Pts',(-9.81469750034251,22.484988205463,3.74264979363137));
#8926=CARTESIAN_POINT('Ctrl Pts',(-9.90250999273814,22.4965529175587,3.50371368221689));
#8927=CARTESIAN_POINT('Ctrl Pts',(-9.98152985600637,22.5081176296544,3.26191090216357));
#8928=CARTESIAN_POINT('Ctrl Pts',(-10.060548278714,22.5196821309211,3.02011253026216));
#8929=CARTESIAN_POINT('Ctrl Pts',(-10.1307743086362,22.5312466321879,2.77544785797645));
#8930=CARTESIAN_POINT('Ctrl Pts',(-10.1920220597857,22.5428111334547,2.52857416993089));
#8931=CARTESIAN_POINT('Ctrl Pts',(-10.253284157106,22.5543783434954,2.28164265621764));
#8932=CARTESIAN_POINT('Ctrl Pts',(-10.3055637050415,22.5659455535361,2.03250136123242));
#8933=CARTESIAN_POINT('Ctrl Pts',(-10.3487254459157,22.5775127635768,1.78182003722534));
#8934=CARTESIAN_POINT('Ctrl Pts',(-10.3861324977168,22.5875377351471,1.56456167176555));
#8935=CARTESIAN_POINT('Ctrl Pts',(-10.4166917642207,22.5975627067174,1.34614685374224));
#8936=CARTESIAN_POINT('Ctrl Pts',(-10.4403464900633,22.6075876782877,1.12701648941934));
#8937=CARTESIAN_POINT('Ctrl Pts',(-10.4692474892472,22.6198360424031,0.859286204883308));
#8938=CARTESIAN_POINT('Ctrl Pts',(-10.4878466242685,22.6320844065186,0.590435506072792));
#8939=CARTESIAN_POINT('Ctrl Pts',(-10.496085593371,22.644332770634,0.32122922754471));
#8940=CARTESIAN_POINT('Ctrl Pts',(-10.4993586516315,22.6491986232481,0.214282858074387));
#8941=CARTESIAN_POINT('Ctrl Pts',(-10.5009972449014,22.6540644758621,0.107280420198263));
#8942=CARTESIAN_POINT('Ctrl Pts',(-10.5009999965284,22.6589303284762,0.000270018945713879));
#8943=CARTESIAN_POINT('',(7.93381306740072,20.,-6.87936125025729));
#8944=CARTESIAN_POINT('Origin',(0.,20.,0.));
#8945=CARTESIAN_POINT('Ctrl Pts',(7.93381306740072,20.,-6.87936125025729));
#8946=CARTESIAN_POINT('Ctrl Pts',(8.33170850771912,20.0276160927694,-6.42047736132949));
#8947=CARTESIAN_POINT('Ctrl Pts',(8.6890477220574,20.054661105705,-5.9279313429));
#8948=CARTESIAN_POINT('Ctrl Pts',(9.25327381718263,20.1041280035438,-4.98862816615476));
#8949=CARTESIAN_POINT('Ctrl Pts',(9.47522497451872,20.126344404341,-4.55297499331653));
#8950=CARTESIAN_POINT('Ctrl Pts',(9.79836691632613,20.1643589694833,-3.79178851112153));
#8951=CARTESIAN_POINT('Ctrl Pts',(9.91553003773292,20.1800057244298,-3.47389058038225));
#8952=CARTESIAN_POINT('Ctrl Pts',(10.0952999382063,20.2076664306373,-2.90237669961849));
#8953=CARTESIAN_POINT('Ctrl Pts',(10.1641960235044,20.219674611679,-2.65103624009131));
#8954=CARTESIAN_POINT('Ctrl Pts',(10.3094356532406,20.2487563952025,-2.03166213315775));
#8955=CARTESIAN_POINT('Ctrl Pts',(10.3755099682223,20.2656411687531,-1.66159912157421));
#8956=CARTESIAN_POINT('Ctrl Pts',(10.4777552458961,20.303032596406,-0.834802718256054));
#8957=CARTESIAN_POINT('Ctrl Pts',(10.5041720493136,20.3235132528092,-0.377643834044697));
#8958=CARTESIAN_POINT('Ctrl Pts',(10.496453767424,20.3695127093978,0.638301907748669));
#8959=CARTESIAN_POINT('Ctrl Pts',(10.4476558813244,20.395092943157,1.1955885646722));
#8960=CARTESIAN_POINT('Ctrl Pts',(10.3016966979839,20.4355285424765,2.06104547614693));
#8961=CARTESIAN_POINT('Ctrl Pts',(10.2342996985265,20.4502475425874,2.37317831113298));
#8962=CARTESIAN_POINT('Ctrl Pts',(10.0570313419514,20.4820093583924,3.04429371137263));
#8963=CARTESIAN_POINT('Ctrl Pts',(9.94192385891823,20.4989006904602,3.40143468374545));
#8964=CARTESIAN_POINT('Ctrl Pts',(9.63986791337795,20.5368593837045,4.1910983082916));
#8965=CARTESIAN_POINT('Ctrl Pts',(9.44243741772192,20.5579055054931,4.61873680006114));
#8966=CARTESIAN_POINT('Ctrl Pts',(8.91191104245967,20.6079994043206,5.5905496196773));
#8967=CARTESIAN_POINT('Ctrl Pts',(8.55663196483671,20.6371917674026,6.12049147995457));
#8968=CARTESIAN_POINT('Ctrl Pts',(7.97378386342717,20.6798218120091,6.83908192755249));
#8969=CARTESIAN_POINT('Ctrl Pts',(7.78284407418771,20.6931119818567,7.05560850752202));
#8970=CARTESIAN_POINT('Ctrl Pts',(7.32890788282693,20.7230916506436,7.52949384767635));
#8971=CARTESIAN_POINT('Ctrl Pts',(7.0608247281153,20.7396254506821,7.78144756106601));
#8972=CARTESIAN_POINT('Ctrl Pts',(6.42926161537202,20.7767429292833,8.31544629874953));
#8973=CARTESIAN_POINT('Ctrl Pts',(6.0593663925618,20.7973022681417,8.58872086019017));
#8974=CARTESIAN_POINT('Ctrl Pts',(5.12991785590839,20.8472877075065,9.18537263375261));
#8975=CARTESIAN_POINT('Ctrl Pts',(4.55612010371929,20.876887788323,9.48308275207275));
#8976=CARTESIAN_POINT('Ctrl Pts',(3.69901264028119,20.9195379465733,9.8319322831093));
#8977=CARTESIAN_POINT('Ctrl Pts',(3.43523340515425,20.9324494287245,9.9271728580165));
#8978=CARTESIAN_POINT('Ctrl Pts',(2.83021902392823,20.9614404354452,10.1186140352906));
#8979=CARTESIAN_POINT('Ctrl Pts',(2.48729389099104,20.9773789866624,10.2083231847577));
#8980=CARTESIAN_POINT('Ctrl Pts',(1.68420993801496,21.0142008888276,10.3755311924679));
#8981=CARTESIAN_POINT('Ctrl Pts',(1.22212278455807,21.0350511105719,10.4400489434024));
#8982=CARTESIAN_POINT('Ctrl Pts',(0.125954152230296,21.0847779393699,10.5193059252721));
#8983=CARTESIAN_POINT('Ctrl Pts',(-0.508197190164823,21.1138006461458,10.5077762010507));
#8984=CARTESIAN_POINT('Ctrl Pts',(-1.42441616088062,21.1562675912602,10.4079480717021));
#8985=CARTESIAN_POINT('Ctrl Pts',(-1.71000102798903,21.1695651291613,10.3648561741657));
#8986=CARTESIAN_POINT('Ctrl Pts',(-2.34296255588236,21.1990213357113,10.2424730595806));
#8987=CARTESIAN_POINT('Ctrl Pts',(-2.68880852581115,21.2150413230804,10.157166930549));
#8988=CARTESIAN_POINT('Ctrl Pts',(-3.47516177481196,21.2519075549319,9.92021883200492));
#8989=CARTESIAN_POINT('Ctrl Pts',(-3.91124289030554,21.2727226706814,9.75651913122846));
#8990=CARTESIAN_POINT('Ctrl Pts',(-4.92738186256186,21.3231991359801,9.29596026407012));
#8991=CARTESIAN_POINT('Ctrl Pts',(-5.49350364275742,21.353033187985,8.97303445559977));
#8992=CARTESIAN_POINT('Ctrl Pts',(-6.25637932893135,21.3959611522619,8.4384707840874));
#8993=CARTESIAN_POINT('Ctrl Pts',(-6.48009235505487,21.4089110064311,8.26791854861376));
#8994=CARTESIAN_POINT('Ctrl Pts',(-6.98250597371194,21.4387064996792,7.85196125438404));
#8995=CARTESIAN_POINT('Ctrl Pts',(-7.25557334748587,21.455387295951,7.60035159506074));
#8996=CARTESIAN_POINT('Ctrl Pts',(-7.83567546319084,21.4926580291033,7.00601774921797));
#8997=CARTESIAN_POINT('Ctrl Pts',(-8.13466751077909,21.5132236303013,6.65652115756698));
#8998=CARTESIAN_POINT('Ctrl Pts',(-8.75160441519402,21.5598569737943,5.8314816379862));
#8999=CARTESIAN_POINT('Ctrl Pts',(-9.05555988987851,21.5859980332283,5.34729517612323));
#9000=CARTESIAN_POINT('Ctrl Pts',(-9.4650561751063,21.6269275040984,4.55900940410054));
#9001=CARTESIAN_POINT('Ctrl Pts',(-9.5985956070701,21.6415732678217,4.27069313825337));
#9002=CARTESIAN_POINT('Ctrl Pts',(-9.86078218491834,21.6732509339197,3.62993266846404));
#9003=CARTESIAN_POINT('Ctrl Pts',(-9.9840306246657,21.6901303635167,3.27575537037389));
#9004=CARTESIAN_POINT('Ctrl Pts',(-10.2178516872492,21.7279344349071,2.46676406607352));
#9005=CARTESIAN_POINT('Ctrl Pts',(-10.3174994780433,21.7488388005139,2.00963136933526));
#9006=CARTESIAN_POINT('Ctrl Pts',(-10.4824452607786,21.7994776004841,0.902482616465333));
#9007=CARTESIAN_POINT('Ctrl Pts',(-10.5182494478197,21.8293840331909,0.250044238442422));
#9008=CARTESIAN_POINT('Ctrl Pts',(-10.4825538342925,21.8724086802026,-0.682940267238052));
#9009=CARTESIAN_POINT('Ctrl Pts',(-10.4604640690836,21.8853803065603,-0.963865308085334));
#9010=CARTESIAN_POINT('Ctrl Pts',(-10.3823265404302,21.9155202319846,-1.619037524658));
#9011=CARTESIAN_POINT('Ctrl Pts',(-10.3172996736249,21.9325133938148,-1.99181280326991));
#9012=CARTESIAN_POINT('Ctrl Pts',(-10.1296190864295,21.9699826338174,-2.80544831621959));
#9013=CARTESIAN_POINT('Ctrl Pts',(-9.99799076945949,21.9904370961928,-3.24343916582445));
#9014=CARTESIAN_POINT('Ctrl Pts',(-9.83826089695888,22.011121265682,-3.67146067980712));
#9015=CARTESIAN_POINT('Origin',(0.,20.,0.));
#9016=CARTESIAN_POINT('',(-9.83826089696967,25.8299813406324,-3.67146067977821));
#9017=CARTESIAN_POINT('',(-9.83826089299223,25.0121157186286,-3.67146069043641));
#9018=CARTESIAN_POINT('',(-9.83826089695937,20.,-3.67146067980583));
#9019=CARTESIAN_POINT('',(-10.5012121264633,25.6589303284762,-0.000261163433911081));
#9020=CARTESIAN_POINT('Ctrl Pts',(-9.83826089696967,25.8299813406324,-3.67146067977821));
#9021=CARTESIAN_POINT('Ctrl Pts',(-9.89045159809829,25.8232071459156,-3.53160742275631));
#9022=CARTESIAN_POINT('Ctrl Pts',(-9.939673531474,25.8164106538706,-3.3906056865579));
#9023=CARTESIAN_POINT('Ctrl Pts',(-10.1287223228633,25.7885121074398,-2.80947855419518));
#9024=CARTESIAN_POINT('Ctrl Pts',(-10.2424427334057,25.767240589704,-2.3614703355705));
#9025=CARTESIAN_POINT('Ctrl Pts',(-10.3824353262031,25.7317358521643,-1.6035935839193));
#9026=CARTESIAN_POINT('Ctrl Pts',(-10.4251238890136,25.717526202749,-1.29741018819776));
#9027=CARTESIAN_POINT('Ctrl Pts',(-10.4853901420833,25.6884582855822,-0.66087079578811));
#9028=CARTESIAN_POINT('Ctrl Pts',(-10.500991607173,25.6736315998779,-0.330663241303831));
#9029=CARTESIAN_POINT('Ctrl Pts',(-10.5009999966147,25.6588081038301,-0.000266641749689656));
#9030=CARTESIAN_POINT('Ctrl Pts',(-9.8390004731412,22.8294636018363,-3.6717362226746));
#9031=CARTESIAN_POINT('Ctrl Pts',(-9.79710281651912,22.8349223685151,-3.78421385875093));
#9032=CARTESIAN_POINT('Ctrl Pts',(-9.11528360003952,22.9197985430557,-5.52171118454613));
#9033=CARTESIAN_POINT('Ctrl Pts',(-6.8861881181333,23.0840921254579,-8.50962861104461));
#9034=CARTESIAN_POINT('Ctrl Pts',(-1.97429514280339,23.322344349043,-10.7673360139992));
#9035=CARTESIAN_POINT('Ctrl Pts',(3.41907203483483,23.5605965726281,-10.3991976830994));
#9036=CARTESIAN_POINT('Ctrl Pts',(7.9786251950841,23.7988487962132,-7.49499206591381));
#9037=CARTESIAN_POINT('Ctrl Pts',(10.5924195565847,24.0371010197983,-2.76297195119323));
#9038=CARTESIAN_POINT('Ctrl Pts',(10.6230253270481,24.2753532433834,2.64285810476577));
#9039=CARTESIAN_POINT('Ctrl Pts',(8.06297863443841,24.5136054669685,7.40417055498215));
#9040=CARTESIAN_POINT('Ctrl Pts',(3.53660174667682,24.7518576905536,10.3598172835396));
#9041=CARTESIAN_POINT('Ctrl Pts',(-1.852251294932,24.9901099141387,10.7890004729458));
#9042=CARTESIAN_POINT('Ctrl Pts',(-6.78939314957438,25.2283621377238,8.58705460123571));
#9043=CARTESIAN_POINT('Ctrl Pts',(-9.85990547775721,25.4513022758363,4.5670737028351));
#9044=CARTESIAN_POINT('Ctrl Pts',(-10.4997645278665,25.5948250060871,1.40951361517464));
#9045=CARTESIAN_POINT('Ctrl Pts',(-10.5012121264633,25.6589303284762,-0.000261163433911081));
#9046=CARTESIAN_POINT('Ctrl Pts',(-9.83826089695889,22.011121265682,-3.67146067980712));
#9047=CARTESIAN_POINT('Ctrl Pts',(-9.83815902016989,22.0111344581847,-3.6717336748129));
#9048=CARTESIAN_POINT('Ctrl Pts',(-9.83805713194903,22.0111476507706,-3.67200666576359));
#9049=CARTESIAN_POINT('Ctrl Pts',(-9.64434668302772,22.0362268124193,-4.19095263523416));
#9050=CARTESIAN_POINT('Ctrl Pts',(-9.41002738239786,22.0615788385252,-4.69349193767824));
#9051=CARTESIAN_POINT('Ctrl Pts',(-8.97712264262286,22.102049618576,-5.45781687901402));
#9052=CARTESIAN_POINT('Ctrl Pts',(-8.80402489973173,22.1170322616488,-5.73285651885139));
#9053=CARTESIAN_POINT('Ctrl Pts',(-8.41440599084763,22.1482450050358,-6.29256191692831));
#9054=CARTESIAN_POINT('Ctrl Pts',(-8.19553555048529,22.1643533526806,-6.57508668780649));
#9055=CARTESIAN_POINT('Ctrl Pts',(-7.65258308910481,22.2017570499126,-7.20661073322297));
#9056=CARTESIAN_POINT('Ctrl Pts',(-7.31832987445934,22.2230196512501,-7.54581411621333));
#9057=CARTESIAN_POINT('Ctrl Pts',(-6.46898209784905,22.2743175656941,-8.29803651587865));
#9058=CARTESIAN_POINT('Ctrl Pts',(-5.9357161480937,22.3045223522079,-8.68748361885374));
#9059=CARTESIAN_POINT('Ctrl Pts',(-5.12394153632778,22.3480516497147,-9.17048920874733));
#9060=CARTESIAN_POINT('Ctrl Pts',(-4.8725168794026,22.3612130171386,-9.3065155146438));
#9061=CARTESIAN_POINT('Ctrl Pts',(-4.29763489393,22.3904554879768,-9.5878491972953));
#9062=CARTESIAN_POINT('Ctrl Pts',(-3.97174141558032,22.4063986100488,-9.72737330635653));
#9063=CARTESIAN_POINT('Ctrl Pts',(-3.20245155002429,22.4432131272224,-10.0116084584261));
#9064=CARTESIAN_POINT('Ctrl Pts',(-2.75523686219245,22.4640520645159,-10.143799346496));
#9065=CARTESIAN_POINT('Ctrl Pts',(-1.66473884588458,22.5146184762881,-10.3886728584124));
#9066=CARTESIAN_POINT('Ctrl Pts',(-1.01684588705719,22.5445200078446,-10.4719560635979));
#9067=CARTESIAN_POINT('Ctrl Pts',(-0.0853416228904833,22.5874704913377,
-10.5043929161344));
#9068=CARTESIAN_POINT('Ctrl Pts',(0.195041786972363,22.6003765838329,-10.502928877526));
#9069=CARTESIAN_POINT('Ctrl Pts',(0.81655748248041,22.6287938592871,-10.4747846598895));
#9070=CARTESIAN_POINT('Ctrl Pts',(1.15711873060623,22.6441823048351,-10.4426509660506));
#9071=CARTESIAN_POINT('Ctrl Pts',(1.95922851258783,22.6805636350815,-10.3272410399013));
#9072=CARTESIAN_POINT('Ctrl Pts',(2.41795474048663,22.701516826454,-10.2295637506253));
#9073=CARTESIAN_POINT('Ctrl Pts',(3.49635554825474,22.7522269050209,-9.92332238117599));
#9074=CARTESIAN_POINT('Ctrl Pts',(4.10609480486743,22.7821548408593,-9.68693834709733));
#9075=CARTESIAN_POINT('Ctrl Pts',(4.94269625392056,22.8252426909853,-9.26933483375999));
#9076=CARTESIAN_POINT('Ctrl Pts',(5.19027498506561,22.8382533542126,-9.13300950794298));
#9077=CARTESIAN_POINT('Ctrl Pts',(5.75040850746558,22.8681520763889,-8.79444022394108));
#9078=CARTESIAN_POINT('Ctrl Pts',(6.05830627436546,22.88487469136,-8.5852376614528));
#9079=CARTESIAN_POINT('Ctrl Pts',(6.72007094510577,22.9221775871373,-8.08223637358721));
#9080=CARTESIAN_POINT('Ctrl Pts',(7.06705417455174,22.9427340794435,-7.78065796364311));
#9081=CARTESIAN_POINT('Ctrl Pts',(7.79751885398652,22.9892960837487,-7.05647798906836));
#9082=CARTESIAN_POINT('Ctrl Pts',(8.16857886507436,23.0153735169989,-6.62340351151992));
#9083=CARTESIAN_POINT('Ctrl Pts',(8.68951133169902,23.0562752807112,-5.9046370081607));
#9084=CARTESIAN_POINT('Ctrl Pts',(8.86451243462568,23.0709572450441,-5.63850751838844));
#9085=CARTESIAN_POINT('Ctrl Pts',(9.33304683409507,23.1129214453884,-4.85012744194704));
#9086=CARTESIAN_POINT('Ctrl Pts',(9.59435339042549,23.1396021008703,-4.31020770155439));
#9087=CARTESIAN_POINT('Ctrl Pts',(9.99983374349218,23.1905863083567,-3.24993259678776));
#9088=CARTESIAN_POINT('Ctrl Pts',(10.1527641376387,23.2148085179695,-2.73497656755786));
#9089=CARTESIAN_POINT('Ctrl Pts',(10.4007629878409,23.2687159474576,-1.58331140976642));
#9090=CARTESIAN_POINT('Ctrl Pts',(10.4780616286908,23.2984558210026,-0.944963989157477));
#9091=CARTESIAN_POINT('Ctrl Pts',(10.5075671360965,23.3450782235732,0.0752577520063168));
#9092=CARTESIAN_POINT('Ctrl Pts',(10.4980074689732,23.3621089064779,0.454394046262921));
#9093=CARTESIAN_POINT('Ctrl Pts',(10.4317614492728,23.3996192632603,1.2876886456361));
#9094=CARTESIAN_POINT('Ctrl Pts',(10.3658589018376,23.4200775574763,1.74033120298424));
#9095=CARTESIAN_POINT('Ctrl Pts',(10.1550289049611,23.4659069337931,2.73033316573101));
#9096=CARTESIAN_POINT('Ctrl Pts',(9.99647915889097,23.4913361835439,3.26338941403484));
#9097=CARTESIAN_POINT('Ctrl Pts',(9.68006758582109,23.5318202650046,4.08312365456022));
#9098=CARTESIAN_POINT('Ctrl Pts',(9.54972305405631,23.5467390083196,4.37931491553579));
#9099=CARTESIAN_POINT('Ctrl Pts',(9.24577669894103,23.5780250103329,4.99162647250862));
#9100=CARTESIAN_POINT('Ctrl Pts',(9.06914863390172,23.5942652616466,5.305776938101));
#9101=CARTESIAN_POINT('Ctrl Pts',(8.62340797158104,23.6317323780177,6.01104391268322));
#9102=CARTESIAN_POINT('Ctrl Pts',(8.34323953991837,23.6529290018979,6.39422899165451));
#9103=CARTESIAN_POINT('Ctrl Pts',(7.61514676227132,23.7040929453002,7.2603481875249));
#9104=CARTESIAN_POINT('Ctrl Pts',(7.1458480924517,23.7342297904803,7.72268928596635));
#9105=CARTESIAN_POINT('Ctrl Pts',(6.41536461271097,23.777665886549,8.31838137924427));
#9106=CARTESIAN_POINT('Ctrl Pts',(6.18704025795914,23.7908046197879,8.4895763911214));
#9107=CARTESIAN_POINT('Ctrl Pts',(5.65868170174971,23.8201057109058,8.85308455988577));
#9108=CARTESIAN_POINT('Ctrl Pts',(5.35526513543522,23.8361272906311,9.03985196730476));
#9109=CARTESIAN_POINT('Ctrl Pts',(4.63496995130448,23.8729884528147,9.43421355827906));
#9110=CARTESIAN_POINT('Ctrl Pts',(4.21261409007777,23.8937966225121,9.63022376952958));
#9111=CARTESIAN_POINT('Ctrl Pts',(3.21948087009429,23.9419578780391,10.0132479869728));
#9112=CARTESIAN_POINT('Ctrl Pts',(2.64287647158049,23.9694124821907,10.1806367538641));
#9113=CARTESIAN_POINT('Ctrl Pts',(1.75287456069259,24.0112332109821,10.3582552497805));
#9114=CARTESIAN_POINT('Ctrl Pts',(1.44807074470326,24.0254447667837,10.4052445727814));
#9115=CARTESIAN_POINT('Ctrl Pts',(0.555767135274358,24.0665008850491,10.5028318669704));
#9116=CARTESIAN_POINT('Ctrl Pts',(-0.0344499151844701,24.092764140141,10.5174700191434));
#9117=CARTESIAN_POINT('Ctrl Pts',(-1.15924631420159,24.1433699730843,10.4506437241561));
#9118=CARTESIAN_POINT('Ctrl Pts',(-1.69245673400647,24.1676350826749,10.377638272027));
#9119=CARTESIAN_POINT('Ctrl Pts',(-2.8435682224278,24.2215227181855,10.1289233613513));
#9120=CARTESIAN_POINT('Ctrl Pts',(-3.45572680846813,24.2511967049917,9.93674531730604));
#9121=CARTESIAN_POINT('Ctrl Pts',(-4.3790713293582,24.2969111099058,9.55115615584327));
#9122=CARTESIAN_POINT('Ctrl Pts',(-4.7042142993661,24.313121006967,9.39527652413933));
#9123=CARTESIAN_POINT('Ctrl Pts',(-5.4277437100935,24.3500962416154,9.00140953445909));
#9124=CARTESIAN_POINT('Ctrl Pts',(-5.81966103042136,24.3708325236976,8.75313178819298));
#9125=CARTESIAN_POINT('Ctrl Pts',(-6.67746466046599,24.418901899173,8.12656570111863));
#9126=CARTESIAN_POINT('Ctrl Pts',(-7.12992670676351,24.446338259833,7.73263979066241));
#9127=CARTESIAN_POINT('Ctrl Pts',(-7.75954682546717,24.4880610182181,7.08198012569272));
#9128=CARTESIAN_POINT('Ctrl Pts',(-7.96300872057675,24.5021958701584,6.85240862926559));
#9129=CARTESIAN_POINT('Ctrl Pts',(-8.52488338439856,24.54299408193,6.15955360840909));
#9130=CARTESIAN_POINT('Ctrl Pts',(-8.85495584636693,24.5690851036403,5.67481298086184));
#9131=CARTESIAN_POINT('Ctrl Pts',(-9.40791733758965,24.6195732197068,4.69599439798748));
#9132=CARTESIAN_POINT('Ctrl Pts',(-9.63641966303246,24.6438970363864,4.20721614263459));
#9133=CARTESIAN_POINT('Ctrl Pts',(-10.0522541068766,24.6978520280123,3.10376689292687));
#9134=CARTESIAN_POINT('Ctrl Pts',(-10.2228003983249,24.7275331235944,2.48505934808134));
#9135=CARTESIAN_POINT('Ctrl Pts',(-10.3984690151572,24.772976314344,1.50608121476103));
#9136=CARTESIAN_POINT('Ctrl Pts',(-10.4433459744648,24.7889144646162,1.15454178886592));
#9137=CARTESIAN_POINT('Ctrl Pts',(-10.505929849523,24.8257262803297,0.336875177503686));
#9138=CARTESIAN_POINT('Ctrl Pts',(-10.5105315440466,24.8465674105374,-0.12949535687918));
#9139=CARTESIAN_POINT('Ctrl Pts',(-10.4472377535106,24.8971385399517,-1.245462253474));
#9140=CARTESIAN_POINT('Ctrl Pts',(-10.349801139714,24.9270426025443,-1.89143581293053));
#9141=CARTESIAN_POINT('Ctrl Pts',(-10.1257429083098,24.9699953718586,-2.79622626179373));
#9142=CARTESIAN_POINT('Ctrl Pts',(-10.0475087846972,24.9829011928103,-3.06547232081995));
#9143=CARTESIAN_POINT('Ctrl Pts',(-9.92043121505545,25.0011979718126,-3.44536206030048));
#9144=CARTESIAN_POINT('Ctrl Pts',(-9.88031276594183,25.0066686769615,-3.55877603111409));
#9145=CARTESIAN_POINT('Ctrl Pts',(-9.83826089299223,25.0121157186286,-3.67146069043641));
#9146=CARTESIAN_POINT('Origin',(0.,20.,0.));
#9147=CARTESIAN_POINT('',(-9.83826091084007,28.8291247138027,-3.67146064261029));
#9148=CARTESIAN_POINT('',(-9.83826088292329,28.0112119827727,-3.67146071741772));
#9149=CARTESIAN_POINT('',(-9.83826089695937,20.,-3.67146067980583));
#9150=CARTESIAN_POINT('Ctrl Pts',(-9.83826091084007,28.8291247138027,-3.67146064261029));
#9151=CARTESIAN_POINT('Ctrl Pts',(-9.87865592041323,28.8238131018187,-3.56321580973253));
#9152=CARTESIAN_POINT('Ctrl Pts',(-9.91726649557972,28.8185104352702,-3.45429895222306));
#9153=CARTESIAN_POINT('Ctrl Pts',(-10.1463566686194,28.7856088690282,-2.77252060102908));
#9154=CARTESIAN_POINT('Ctrl Pts',(-10.2889335781495,28.7587218828267,-2.18478333336485));
#9155=CARTESIAN_POINT('Ctrl Pts',(-10.460636635831,28.7077180821375,-1.06244929267068));
#9156=CARTESIAN_POINT('Ctrl Pts',(-10.5010088482604,28.6836978808386,-0.531517047903976));
#9157=CARTESIAN_POINT('Ctrl Pts',(-10.5009915652785,28.6361742225104,0.506848100517199));
#9158=CARTESIAN_POINT('Ctrl Pts',(-10.4643124591535,28.6127661383962,1.012854700152));
#9159=CARTESIAN_POINT('Ctrl Pts',(-10.349077464141,28.5760384018781,1.80364652905196));
#9160=CARTESIAN_POINT('Ctrl Pts',(-10.2948284982149,28.5626854573338,2.09118625213222));
#9161=CARTESIAN_POINT('Ctrl Pts',(-10.1524018818668,28.5342484550003,2.70430645000063));
#9162=CARTESIAN_POINT('Ctrl Pts',(-10.0604050604299,28.5191670709985,3.02866161267971));
#9163=CARTESIAN_POINT('Ctrl Pts',(-9.78078089020341,28.4798136980383,3.8599232156621));
#9164=CARTESIAN_POINT('Ctrl Pts',(-9.56935865845635,28.4555078685281,4.35775621233012));
#9165=CARTESIAN_POINT('Ctrl Pts',(-9.10866277396772,28.4098552854066,5.24546805337249));
#9166=CARTESIAN_POINT('Ctrl Pts',(-8.87012987032504,28.3886625424817,5.63945549867554));
#9167=CARTESIAN_POINT('Ctrl Pts',(-8.39481116936552,28.3504421612671,6.31939104680849));
#9168=CARTESIAN_POINT('Ctrl Pts',(-8.16724069797434,28.333462568094,6.61088141490322));
#9169=CARTESIAN_POINT('Ctrl Pts',(-7.73920684218572,28.3039186601339,7.10321544846201));
#9170=CARTESIAN_POINT('Ctrl Pts',(-7.54509277020654,28.2912278366045,7.30907454270442));
#9171=CARTESIAN_POINT('Ctrl Pts',(-6.87626451667295,28.249253774505,7.96329609522314));
#9172=CARTESIAN_POINT('Ctrl Pts',(-6.36809015951772,28.2199823966844,8.37523151930707));
#9173=CARTESIAN_POINT('Ctrl Pts',(-5.43481699171802,28.1687475870897,8.99742455172715));
#9174=CARTESIAN_POINT('Ctrl Pts',(-5.02767534204249,28.1471316927054,9.23110799371259));
#9175=CARTESIAN_POINT('Ctrl Pts',(-4.29994499453645,28.1098356133824,9.58632782094374));
#9176=CARTESIAN_POINT('Ctrl Pts',(-3.98649222318385,28.0941873969082,9.72085906386877));
#9177=CARTESIAN_POINT('Ctrl Pts',(-3.40413257847277,28.0660391936369,9.93788732317606));
#9178=CARTESIAN_POINT('Ctrl Pts',(-3.13739759613245,28.0534477669827,10.0252911521772));
#9179=CARTESIAN_POINT('Ctrl Pts',(-2.24047447567557,28.0116178341672,10.2798875697885));
#9180=CARTESIAN_POINT('Ctrl Pts',(-1.59827124573953,27.9823970318907,10.3991019236625));
#9181=CARTESIAN_POINT('Ctrl Pts',(-0.484954907263053,27.931344590157,10.5001475895433));
#9182=CARTESIAN_POINT('Ctrl Pts',(-0.0184444661739987,27.9098617345736,
10.5113239048773));
#9183=CARTESIAN_POINT('Ctrl Pts',(0.80045003192573,27.8721083103663,10.4764142106946));
#9184=CARTESIAN_POINT('Ctrl Pts',(1.15267038956768,27.8558777032382,10.4435310354543));
#9185=CARTESIAN_POINT('Ctrl Pts',(1.78542266794532,27.8269296983462,10.3520502820949));
#9186=CARTESIAN_POINT('Ctrl Pts',(2.06649138533566,27.8141079633993,10.2996260059725));
#9187=CARTESIAN_POINT('Ctrl Pts',(2.98725169581614,27.77173041069,10.0886752059421));
#9188=CARTESIAN_POINT('Ctrl Pts',(3.61414735214316,27.7421777932464,9.88144496242516));
#9189=CARTESIAN_POINT('Ctrl Pts',(4.65307470562964,27.6903362940943,9.42582279508626));
#9190=CARTESIAN_POINT('Ctrl Pts',(5.07518644878895,27.6683996593876,9.20541754112403));
#9191=CARTESIAN_POINT('Ctrl Pts',(5.78555358165188,27.630055308456,8.77074345285593));
#9192=CARTESIAN_POINT('Ctrl Pts',(6.08051194093631,27.6136918223141,8.56889497459747));
#9193=CARTESIAN_POINT('Ctrl Pts',(6.62300614190321,27.5828647896981,8.15550868870517));
#9194=CARTESIAN_POINT('Ctrl Pts',(6.87212015002063,27.5683179981145,7.94672893050593));
#9195=CARTESIAN_POINT('Ctrl Pts',(7.51850943189882,27.5289058692825,7.35183672079408));
#9196=CARTESIAN_POINT('Ctrl Pts',(7.89557003381352,27.5040110994093,6.94531806600125));
#9197=CARTESIAN_POINT('Ctrl Pts',(8.52232467977584,27.4578818150736,6.15223976145366));
#9198=CARTESIAN_POINT('Ctrl Pts',(8.78209427500418,27.4368254140924,5.7753685342449));
#9199=CARTESIAN_POINT('Ctrl Pts',(9.21023571901058,27.3983421045552,5.05820620088779));
#9200=CARTESIAN_POINT('Ctrl Pts',(9.38634076996834,27.3809665043756,4.72340085038933));
#9201=CARTESIAN_POINT('Ctrl Pts',(9.66153206116036,27.3510852179623,4.12373496024748));
#9202=CARTESIAN_POINT('Ctrl Pts',(9.76869846150711,27.3384413218305,3.86302025304477));
#9203=CARTESIAN_POINT('Ctrl Pts',(10.0886555350229,27.2965501609103,2.98581479684692));
#9204=CARTESIAN_POINT('Ctrl Pts',(10.2545304733166,27.267317565445,2.35385693556927));
#9205=CARTESIAN_POINT('Ctrl Pts',(10.4368743717964,27.2161934001995,1.24945043154621));
#9206=CARTESIAN_POINT('Ctrl Pts',(10.4821394408103,27.1946494940426,0.783719067757864));
#9207=CARTESIAN_POINT('Ctrl Pts',(10.5075148188313,27.1558757564564,-0.0577294557712837));
#9208=CARTESIAN_POINT('Ctrl Pts',(10.4987761814546,27.1387016418583,-0.432338556765475));
#9209=CARTESIAN_POINT('Ctrl Pts',(10.4457119065858,27.1074326089507,-1.12191544444419));
#9210=CARTESIAN_POINT('Ctrl Pts',(10.4070636928996,27.0932258532195,-1.43687872092839));
#9211=CARTESIAN_POINT('Ctrl Pts',(10.2589372280531,27.0533422556544,-2.31349282487628));
#9212=CARTESIAN_POINT('Ctrl Pts',(10.1177536861628,27.0276377850881,-2.8686378727547));
#9213=CARTESIAN_POINT('Ctrl Pts',(9.78290341033973,26.9805648681496,-3.84407294962027));
#9214=CARTESIAN_POINT('Ctrl Pts',(9.60536923028663,26.9594022522756,-4.26836825030155));
#9215=CARTESIAN_POINT('Ctrl Pts',(9.23513606089142,26.9211264220879,-5.01210178079168));
#9216=CARTESIAN_POINT('Ctrl Pts',(9.05212486952971,26.904062007347,-5.33553687625689));
#9217=CARTESIAN_POINT('Ctrl Pts',(8.70035963719141,26.874446936582,-5.88681505644243));
#9218=CARTESIAN_POINT('Ctrl Pts',(8.5388048770834,26.8617672673773,-6.11879595360297));
#9219=CARTESIAN_POINT('Ctrl Pts',(7.97388556503127,26.8198155424908,-6.86395833918171));
#9220=CARTESIAN_POINT('Ctrl Pts',(7.53208180673409,26.7905560253361,-7.34605306975006));
#9221=CARTESIAN_POINT('Ctrl Pts',(6.70111001494593,26.7393519240148,-8.09849614544494));
#9222=CARTESIAN_POINT('Ctrl Pts',(6.33315604796249,26.717754826784,-8.38937658895251));
#9223=CARTESIAN_POINT('Ctrl Pts',(5.66531986722898,26.6804348274477,-8.84827516267339));
#9224=CARTESIAN_POINT('Ctrl Pts',(5.37433179608604,26.6647445071336,-9.02797837314898));
#9225=CARTESIAN_POINT('Ctrl Pts',(4.51347728910668,26.6202075278006,-9.50321302013761));
#9226=CARTESIAN_POINT('Ctrl Pts',(3.92462964793251,26.5917225675874,-9.76113912543414));
#9227=CARTESIAN_POINT('Ctrl Pts',(2.80818579361606,26.5385947654838,-10.1326921208555));
#9228=CARTESIAN_POINT('Ctrl Pts',(2.28828057551133,26.5141910295174,-10.2626071530311));
#9229=CARTESIAN_POINT('Ctrl Pts',(1.16810232698847,26.4619090371942,-10.4531304803375));
#9230=CARTESIAN_POINT('Ctrl Pts',(0.567868246511755,26.4341067707607,-10.5028553427611));
#9231=CARTESIAN_POINT('Ctrl Pts',(-0.351408512689415,26.3925461627676,-10.4999375061956));
#9232=CARTESIAN_POINT('Ctrl Pts',(-0.669279215390337,26.3782987851555,-10.484476361876));
#9233=CARTESIAN_POINT('Ctrl Pts',(-1.55313663816918,26.3384715239668,-10.4011210371498));
#9234=CARTESIAN_POINT('Ctrl Pts',(-2.1150097324725,26.3128636795486,-10.3015662406973));
#9235=CARTESIAN_POINT('Ctrl Pts',(-3.11016169909518,26.2659035284779,-10.0403558899959));
#9236=CARTESIAN_POINT('Ctrl Pts',(-3.54617229251944,26.2447536668076,-9.89477154102883));
#9237=CARTESIAN_POINT('Ctrl Pts',(-4.31573647487857,26.2064539224273,-9.58039139671548));
#9238=CARTESIAN_POINT('Ctrl Pts',(-4.65251401597445,26.1893531532413,-9.42144416325672));
#9239=CARTESIAN_POINT('Ctrl Pts',(-5.22883403661191,26.1597073858888,-9.11098706163269));
#9240=CARTESIAN_POINT('Ctrl Pts',(-5.47201374754287,26.1470323010079,-8.96704296246385));
#9241=CARTESIAN_POINT('Ctrl Pts',(-6.25667282360332,26.1050892662708,-8.45876478369332));
#9242=CARTESIAN_POINT('Ctrl Pts',(-6.76999237242064,26.0758341315137,-8.05380883545692));
#9243=CARTESIAN_POINT('Ctrl Pts',(-7.58155294914752,26.0246418254573,-7.28082583311357));
#9244=CARTESIAN_POINT('Ctrl Pts',(-7.89870727803254,26.003052135242,-6.93547280967408));
#9245=CARTESIAN_POINT('Ctrl Pts',(-8.4074952058364,25.9655987617559,-6.30110611875553));
#9246=CARTESIAN_POINT('Ctrl Pts',(-8.60987269290143,25.9497695737279,-6.02162932995481));
#9247=CARTESIAN_POINT('Ctrl Pts',(-8.95277371293878,25.9213253381718,-5.49536895439635));
#9248=CARTESIAN_POINT('Ctrl Pts',(-9.09774629233561,25.9086154292961,-5.25188088533478));
#9249=CARTESIAN_POINT('Ctrl Pts',(-9.46534003125153,25.8739996172454,-4.57348815313626));
#9250=CARTESIAN_POINT('Ctrl Pts',(-9.66766124650532,25.8521246578494,-4.12860948690843));
#9251=CARTESIAN_POINT('Ctrl Pts',(-9.83826089696969,25.8299813406324,-3.67146067977821));
#9252=CARTESIAN_POINT('Ctrl Pts',(-9.83826089299223,25.0121157186286,-3.67146069043641));
#9253=CARTESIAN_POINT('Ctrl Pts',(-9.76075300064936,25.0221554312385,-3.87915537395064));
#9254=CARTESIAN_POINT('Ctrl Pts',(-9.67667706671879,25.0321241213543,-4.08437205702527));
#9255=CARTESIAN_POINT('Ctrl Pts',(-9.39493386590707,25.0631086038194,-4.71440637966613));
#9256=CARTESIAN_POINT('Ctrl Pts',(-9.17532054386728,25.0840583919932,-5.12873264663993));
#9257=CARTESIAN_POINT('Ctrl Pts',(-8.5853534378316,25.134762535786,-6.0818138649344));
#9258=CARTESIAN_POINT('Ctrl Pts',(-8.19096716067736,25.1646879750445,-6.60339082686781));
#9259=CARTESIAN_POINT('Ctrl Pts',(-7.56016458876944,25.207771580521,-7.29347011223664));
#9260=CARTESIAN_POINT('Ctrl Pts',(-7.36124113141074,25.2207806331471,-7.49419284956908));
#9261=CARTESIAN_POINT('Ctrl Pts',(-6.88210665288705,25.2506818667835,-7.94015441478219));
#9262=CARTESIAN_POINT('Ctrl Pts',(-6.59647108555561,25.2674084493627,-8.17899853859639));
#9263=CARTESIAN_POINT('Ctrl Pts',(-5.93133099321032,25.304713920329,-8.67762534715816));
#9264=CARTESIAN_POINT('Ctrl Pts',(-5.54623931221407,25.3252690517141,-8.92866693588708));
#9265=CARTESIAN_POINT('Ctrl Pts',(-4.6494360944431,25.3718403495577,-9.43282527750661));
#9266=CARTESIAN_POINT('Ctrl Pts',(-4.1310365331164,25.3979287662914,-9.67108880676581));
#9267=CARTESIAN_POINT('Ctrl Pts',(-3.29696622650543,25.4388329004323,-9.97508104006006));
#9268=CARTESIAN_POINT('Ctrl Pts',(-2.99324090409898,25.4535062711629,-10.0703892329591));
#9269=CARTESIAN_POINT('Ctrl Pts',(-2.10506466790359,25.4955449089419,-10.3053569839323));
#9270=CARTESIAN_POINT('Ctrl Pts',(-1.51237793076189,25.5223041541911,-10.4088616502049));
#9271=CARTESIAN_POINT('Ctrl Pts',(-0.380666846091074,25.5733287540954,-10.5077496005324));
#9272=CARTESIAN_POINT('Ctrl Pts',(0.155523981271924,25.5975096870528,-10.5134913766237));
#9273=CARTESIAN_POINT('Ctrl Pts',(1.32917141982183,25.651333161507,-10.4362288265948));
#9274=CARTESIAN_POINT('Ctrl Pts',(1.96334113481097,25.6810303074909,-10.3357073884281));
#9275=CARTESIAN_POINT('Ctrl Pts',(2.95246986269504,25.7276465117983,-10.0845500377189));
#9276=CARTESIAN_POINT('Ctrl Pts',(3.3152140893724,25.7447118335475,-9.97118785461763));
#9277=CARTESIAN_POINT('Ctrl Pts',(4.09889665007971,25.7822459427528,-9.67877093641956));
#9278=CARTESIAN_POINT('Ctrl Pts',(4.51589019677931,25.802693588194,-9.49137981413581));
#9279=CARTESIAN_POINT('Ctrl Pts',(5.41111758709042,25.8485735132144,-9.01668622542121));
#9280=CARTESIAN_POINT('Ctrl Pts',(5.88135822648925,25.874065878704,-8.71724865256425));
#9281=CARTESIAN_POINT('Ctrl Pts',(6.58287739329119,25.9145592424325,-8.18783165650493));
#9282=CARTESIAN_POINT('Ctrl Pts',(6.83104727622634,25.9294242228729,-7.98195824528117));
#9283=CARTESIAN_POINT('Ctrl Pts',(7.33765945003296,25.960778306039,-7.52073180747464));
#9284=CARTESIAN_POINT('Ctrl Pts',(7.5931174670888,25.977135738209,-7.26272844811498));
#9285=CARTESIAN_POINT('Ctrl Pts',(8.14956108161896,26.014662332474,-6.63922026589004));
#9286=CARTESIAN_POINT('Ctrl Pts',(8.44021647823084,26.0358033303613,-6.2655673058368));
#9287=CARTESIAN_POINT('Ctrl Pts',(9.07168109751893,26.0868563765776,-5.32973469143728));
#9288=CARTESIAN_POINT('Ctrl Pts',(9.38687688222927,26.1169380608015,-4.75268042787667));
#9289=CARTESIAN_POINT('Ctrl Pts',(9.75869492583654,26.1602934449843,-3.88843960106565));
#9290=CARTESIAN_POINT('Ctrl Pts',(9.86054699868495,26.173409025586,-3.6223893556622));
#9291=CARTESIAN_POINT('Ctrl Pts',(10.0658754506011,26.2027922734766,-3.01290350970603));
#9292=CARTESIAN_POINT('Ctrl Pts',(10.1628282762837,26.218915593411,-2.66765084903357));
#9293=CARTESIAN_POINT('Ctrl Pts',(10.3444142603852,26.2558379303364,-1.86536188076883));
#9294=CARTESIAN_POINT('Ctrl Pts',(10.4167525674532,26.2766068380195,-1.40632236420041));
#9295=CARTESIAN_POINT('Ctrl Pts',(10.5123409898598,26.3247205777358,-0.34731705689704));
#9296=CARTESIAN_POINT('Ctrl Pts',(10.5150351460995,26.3521679604852,0.252876673934817));
#9297=CARTESIAN_POINT('Ctrl Pts',(10.4416651182508,26.3939367716773,1.15632261822086));
#9298=CARTESIAN_POINT('Ctrl Pts',(10.4033527110059,26.4081052652601,1.46140592339454));
#9299=CARTESIAN_POINT('Ctrl Pts',(10.2530593062309,26.4490169093351,2.34319045607481));
#9300=CARTESIAN_POINT('Ctrl Pts',(10.1060337161021,26.4751837781094,2.91270616932516));
#9301=CARTESIAN_POINT('Ctrl Pts',(9.73449756649101,26.5257235690258,3.97494396375965));
#9302=CARTESIAN_POINT('Ctrl Pts',(9.51803608469693,26.5500213790414,4.46851105848206));
#9303=CARTESIAN_POINT('Ctrl Pts',(8.96315700599671,26.6039555873216,5.50846234220355));
#9304=CARTESIAN_POINT('Ctrl Pts',(8.610530850104,26.6336428646415,6.04483960405354));
#9305=CARTESIAN_POINT('Ctrl Pts',(7.98821598006915,26.6792547471245,6.82549740762069));
#9306=CARTESIAN_POINT('Ctrl Pts',(7.75104619252017,26.6953518367844,7.09367998963111));
#9307=CARTESIAN_POINT('Ctrl Pts',(7.17560663216171,26.7322582971608,7.68097440837005));
#9308=CARTESIAN_POINT('Ctrl Pts',(6.82892181902772,26.7530372293412,7.99077721654748));
#9309=CARTESIAN_POINT('Ctrl Pts',(5.9906111882726,26.8011637342064,8.645380300992));
#9310=CARTESIAN_POINT('Ctrl Pts',(5.48766322039095,26.8286136123418,8.97304540426886));
#9311=CARTESIAN_POINT('Ctrl Pts',(4.68844432601075,26.8703960538427,9.40128095225348));
#9312=CARTESIAN_POINT('Ctrl Pts',(4.41109611238629,26.8845752610326,9.53455962749087));
#9313=CARTESIAN_POINT('Ctrl Pts',(3.58790307356012,26.9255229314759,9.8865243228236));
#9314=CARTESIAN_POINT('Ctrl Pts',(3.02907594088133,26.9517138599482,10.0717981834828));
#9315=CARTESIAN_POINT('Ctrl Pts',(1.93464259117908,27.0022700979017,10.335258862224));
#9316=CARTESIAN_POINT('Ctrl Pts',(1.40271844505116,27.0265597097168,10.4207858762804));
#9317=CARTESIAN_POINT('Ctrl Pts',(0.228369115918427,27.0804780387298,10.5180310647503));
#9318=CARTESIAN_POINT('Ctrl Pts',(-0.413348270803016,27.1101576545282,10.5123860107341));
#9319=CARTESIAN_POINT('Ctrl Pts',(-1.40663598019266,27.1557670161011,10.4125147720544));
#9320=CARTESIAN_POINT('Ctrl Pts',(-1.76066499763962,27.171868980435,10.3585303443809));
#9321=CARTESIAN_POINT('Ctrl Pts',(-2.56616123710465,27.2087783859612,10.1932072701764));
#9322=CARTESIAN_POINT('Ctrl Pts',(-3.01436912110219,27.2295554501554,10.0697682236358));
#9323=CARTESIAN_POINT('Ctrl Pts',(-4.01878417821638,27.2776796084062,9.72005053985172));
#9324=CARTESIAN_POINT('Ctrl Pts',(-4.56672628561487,27.3051290545453,9.47496640068579));
#9325=CARTESIAN_POINT('Ctrl Pts',(-5.359722030793,27.3469089750363,9.0354273261699));
#9326=CARTESIAN_POINT('Ctrl Pts',(-5.6220087946756,27.3610861715226,8.87460347217745));
#9327=CARTESIAN_POINT('Ctrl Pts',(-6.36383353765463,27.4020270840498,8.37364397057684));
#9328=CARTESIAN_POINT('Ctrl Pts',(-6.82233664236446,27.4282135003865,8.0045000738226));
#9329=CARTESIAN_POINT('Ctrl Pts',(-7.63688730562669,27.4787666518605,7.22761428973073));
#9330=CARTESIAN_POINT('Ctrl Pts',(-7.99709220919185,27.5030577992767,6.82692843427301));
#9331=CARTESIAN_POINT('Ctrl Pts',(-8.71535856676066,27.5569793595116,5.89268204537063));
#9332=CARTESIAN_POINT('Ctrl Pts',(-9.05844354768592,27.5866606750433,5.35030500272587));
#9333=CARTESIAN_POINT('Ctrl Pts',(-9.51288968886619,27.6322721271269,4.46139273755004));
#9334=CARTESIAN_POINT('Ctrl Pts',(-9.65940689536713,27.6483745054719,4.13460485312264));
#9335=CARTESIAN_POINT('Ctrl Pts',(-9.95704584452271,27.6852841612461,3.36806956048787));
#9336=CARTESIAN_POINT('Ctrl Pts',(-10.0962334208425,27.7060610668963,2.92450347137084));
#9337=CARTESIAN_POINT('Ctrl Pts',(-10.3467201885116,27.7541850252979,1.89086987561539));
#9338=CARTESIAN_POINT('Ctrl Pts',(-10.4377356413369,27.7816344340699,1.29755567173516));
#9339=CARTESIAN_POINT('Ctrl Pts',(-10.4981514713004,27.8234141401926,0.392913033911138));
#9340=CARTESIAN_POINT('Ctrl Pts',(-10.5051552215293,27.8375911663282,0.0853299485340096));
#9341=CARTESIAN_POINT('Ctrl Pts',(-10.4862215596595,27.8785315062419,-0.809591124987056));
#9342=CARTESIAN_POINT('Ctrl Pts',(-10.4245064953328,27.9047175402339,-1.39497411059982));
#9343=CARTESIAN_POINT('Ctrl Pts',(-10.2131096014756,27.9552704302117,-2.50057024650288));
#9344=CARTESIAN_POINT('Ctrl Pts',(-10.0716088916502,27.9795617077902,-3.02045248795448));
#9345=CARTESIAN_POINT('Ctrl Pts',(-9.87370387496888,28.0065212948858,-3.57541525405906));
#9346=CARTESIAN_POINT('Ctrl Pts',(-9.85615642006742,28.0088658143616,-3.62350678937248));
#9347=CARTESIAN_POINT('Ctrl Pts',(-9.83826088292329,28.0112119827727,-3.67146071741772));
#9348=CARTESIAN_POINT('Origin',(0.,20.,0.));
#9349=CARTESIAN_POINT('',(-9.83826093350753,31.8296488111843,-3.67146058186924));
#9350=CARTESIAN_POINT('',(-9.83826089557905,31.0116616139852,-3.67146068350461));
#9351=CARTESIAN_POINT('',(-9.83826089695937,20.,-3.67146067980583));
#9352=CARTESIAN_POINT('',(-10.5010003051392,31.6584104925326,-4.11482518479439E-5));
#9353=CARTESIAN_POINT('Ctrl Pts',(-9.83826093350753,31.8296488111843,-3.67146058186924));
#9354=CARTESIAN_POINT('Ctrl Pts',(-10.0094795081984,31.8076523557889,-3.21265325521828));
#9355=CARTESIAN_POINT('Ctrl Pts',(-10.1484321693502,31.7855438356587,-2.74232807173823));
#9356=CARTESIAN_POINT('Ctrl Pts',(-10.4181972024547,31.7283755090288,-1.520467410793));
#9357=CARTESIAN_POINT('Ctrl Pts',(-10.5009970189966,31.6929958703928,-0.761382904710808));
#9358=CARTESIAN_POINT('Ctrl Pts',(-10.5009999999195,31.6584099621222,-4.11151364069526E-5));
#9359=CARTESIAN_POINT('Ctrl Pts',(-10.5009999999193,31.6584099647158,-4.11722280356519E-5));
#9360=CARTESIAN_POINT('Ctrl Pts',(-10.5010029719109,31.623975496371,0.757966959591466));
#9361=CARTESIAN_POINT('Ctrl Pts',(-10.4189324737747,31.5904413899423,1.51376024549679));
#9362=CARTESIAN_POINT('Ctrl Pts',(-10.1312166813896,31.5297580311426,2.82285787600405));
#9363=CARTESIAN_POINT('Ctrl Pts',(-9.9591335994681,31.5030737741803,3.38019336946323));
#9364=CARTESIAN_POINT('Ctrl Pts',(-9.62657157092227,31.4620254817805,4.2065783101474));
#9365=CARTESIAN_POINT('Ctrl Pts',(-9.49883576393913,31.4478018133524,4.48757204654972));
#9366=CARTESIAN_POINT('Ctrl Pts',(-9.19329425687296,31.4169876093467,5.08799528102228));
#9367=CARTESIAN_POINT('Ctrl Pts',(-9.01081404737691,31.4005399667176,5.40458965930672));
#9368=CARTESIAN_POINT('Ctrl Pts',(-8.5574470493751,31.3631151825095,6.1041403530954));
#9369=CARTESIAN_POINT('Ctrl Pts',(-8.27667154015362,31.3421644954908,6.47974794710526));
#9370=CARTESIAN_POINT('Ctrl Pts',(-7.54702729141367,31.2914589448984,7.33069901596518));
#9371=CARTESIAN_POINT('Ctrl Pts',(-7.07705673809412,31.2615330123196,7.78537069265081));
#9372=CARTESIAN_POINT('Ctrl Pts',(-6.34753993713335,31.2184481879107,8.37015769482052));
#9373=CARTESIAN_POINT('Ctrl Pts',(-6.12008149546854,31.2054384573527,8.53788077642229));
#9374=CARTESIAN_POINT('Ctrl Pts',(-5.57809952373071,31.1755417669533,8.90472709394489));
#9375=CARTESIAN_POINT('Ctrl Pts',(-5.25920760678224,31.1588202271627,9.09670808727943));
#9376=CARTESIAN_POINT('Ctrl Pts',(-4.52532749965072,31.1215181078612,9.48700771984015));
#9377=CARTESIAN_POINT('Ctrl Pts',(-4.10615558996647,31.1009613292202,9.67581446052378));
#9378=CARTESIAN_POINT('Ctrl Pts',(-3.1426498840517,31.0543998783173,10.0358812627618));
#9379=CARTESIAN_POINT('Ctrl Pts',(-2.59400862506019,31.0283233163457,10.1914794378608));
#9380=CARTESIAN_POINT('Ctrl Pts',(-1.72315646797506,30.9874217168502,10.3635460562461));
#9381=CARTESIAN_POINT('Ctrl Pts',(-1.40818649056257,30.9727390482237,10.4110214790555));
#9382=CARTESIAN_POINT('Ctrl Pts',(-0.496105447267984,30.9307770581461,10.5063458167437));
#9383=CARTESIAN_POINT('Ctrl Pts',(0.103554571297619,30.9040991535197,10.5175428444798));
#9384=CARTESIAN_POINT('Ctrl Pts',(1.23615810814353,30.853116318168,10.4417760482636));
#9385=CARTESIAN_POINT('Ctrl Pts',(1.76786438535313,30.8288926177573,10.3650088809611));
#9386=CARTESIAN_POINT('Ctrl Pts',(2.91882883017579,30.7749248798937,10.1076621676343));
#9387=CARTESIAN_POINT('Ctrl Pts',(3.53207512909303,30.7451244531409,9.91003673895346));
#9388=CARTESIAN_POINT('Ctrl Pts',(4.43795670876226,30.7001341715368,9.52326297092287));
#9389=CARTESIAN_POINT('Ctrl Pts',(4.74577646543308,30.6847381374973,9.37366557264447));
#9390=CARTESIAN_POINT('Ctrl Pts',(5.45655018352348,30.6483526025346,8.98423469998865));
#9391=CARTESIAN_POINT('Ctrl Pts',(5.85182343138215,30.6274026682853,8.73192827296279));
#9392=CARTESIAN_POINT('Ctrl Pts',(6.75423761367047,30.5766983083303,8.06703353008391));
#9393=CARTESIAN_POINT('Ctrl Pts',(7.2423188522358,30.5467728018786,7.63187612968911));
#9394=CARTESIAN_POINT('Ctrl Pts',(7.87929346817327,30.503688992417,6.94748378035463));
#9395=CARTESIAN_POINT('Ctrl Pts',(8.06332541754961,30.4906798117367,6.73302177484321));
#9396=CARTESIAN_POINT('Ctrl Pts',(8.46918835254721,30.4607796181574,6.21950751259473));
#9397=CARTESIAN_POINT('Ctrl Pts',(8.68421041660464,30.4440541640326,5.91556575944822));
#9398=CARTESIAN_POINT('Ctrl Pts',(9.12757966406785,30.4067494562523,5.21240502546104));
#9399=CARTESIAN_POINT('Ctrl Pts',(9.3467605432577,30.3861939693831,4.80831974446729));
#9400=CARTESIAN_POINT('Ctrl Pts',(9.77695256372727,30.3396249280172,3.87383297196255));
#9401=CARTESIAN_POINT('Ctrl Pts',(9.97262920115203,30.3135392046698,3.337966894007));
#9402=CARTESIAN_POINT('Ctrl Pts',(10.2083958280231,30.2726356587073,2.48211832055813));
#9403=CARTESIAN_POINT('Ctrl Pts',(10.2789190544463,30.257960187701,2.17165424717177));
#9404=CARTESIAN_POINT('Ctrl Pts',(10.4414565501759,30.215936859755,1.26775671570833));
#9405=CARTESIAN_POINT('Ctrl Pts',(10.4968383957213,30.1891940897518,0.669039387544863));
#9406=CARTESIAN_POINT('Ctrl Pts',(10.5042868157778,30.1381779524306,-0.466779564517998));
#9407=CARTESIAN_POINT('Ctrl Pts',(10.4668101813873,30.1139883520765,-1.00189271282337));
#9408=CARTESIAN_POINT('Ctrl Pts',(10.2951847713318,30.0601486322426,-2.1658595525262));
#9409=CARTESIAN_POINT('Ctrl Pts',(10.1438419931816,30.030443939003,-2.79002392599146));
#9410=CARTESIAN_POINT('Ctrl Pts',(9.81388306759422,29.9838446633388,-3.75533219169576));
#9411=CARTESIAN_POINT('Ctrl Pts',(9.67187482201498,29.9668029547496,-4.10726941975931));
#9412=CARTESIAN_POINT('Ctrl Pts',(9.31750355162947,29.9292850872525,-4.8645496016262));
#9413=CARTESIAN_POINT('Ctrl Pts',(9.09707562871007,29.9088302317151,-5.26525637970499));
#9414=CARTESIAN_POINT('Ctrl Pts',(8.55224960660479,29.8629849568965,-6.11872774650409));
#9415=CARTESIAN_POINT('Ctrl Pts',(8.21653890499678,29.8375357624051,-6.56264167301637));
#9416=CARTESIAN_POINT('Ctrl Pts',(7.63261845744045,29.7970488080632,-7.21931479187445));
#9417=CARTESIAN_POINT('Ctrl Pts',(7.40691609965493,29.7821471167866,-7.45070243484553));
#9418=CARTESIAN_POINT('Ctrl Pts',(6.90719511346969,29.750840913549,-7.91782586000983));
#9419=CARTESIAN_POINT('Ctrl Pts',(6.63095358837488,29.7345648394487,-8.15056865789208));
#9420=CARTESIAN_POINT('Ctrl Pts',(5.96572279077559,29.6970797713222,-8.65480137096482));
#9421=CARTESIAN_POINT('Ctrl Pts',(5.56924809301941,29.6759003705688,-8.91509435014499));
#9422=CARTESIAN_POINT('Ctrl Pts',(4.58426022019142,29.624770997779,-9.47033038367636));
#9423=CARTESIAN_POINT('Ctrl Pts',(3.98296225200876,29.5946514738936,-9.73850963354644));
#9424=CARTESIAN_POINT('Ctrl Pts',(3.09046721182634,29.5512403602524,-10.0399850438766));
#9425=CARTESIAN_POINT('Ctrl Pts',(2.81674775674761,29.5381085529275,-10.1201888279556));
#9426=CARTESIAN_POINT('Ctrl Pts',(2.19395682337431,29.5087837409927,-10.2754473268974));
#9427=CARTESIAN_POINT('Ctrl Pts',(1.84364424209252,29.4927325531931,-10.3440438740099));
#9428=CARTESIAN_POINT('Ctrl Pts',(1.03037329502299,29.4558537217162,-10.4606602287176));
#9429=CARTESIAN_POINT('Ctrl Pts',(0.566365628337865,29.4350571039316,-10.4960138577852));
#9430=CARTESIAN_POINT('Ctrl Pts',(-0.497703865727678,29.3869091447435,-10.5063041963415));
#9431=CARTESIAN_POINT('Ctrl Pts',(-1.09633936813621,29.3594559615501,-10.4607908615899));
#9432=CARTESIAN_POINT('Ctrl Pts',(-1.99177299762381,29.3176500776683,-10.3149740767657));
#9433=CARTESIAN_POINT('Ctrl Pts',(-2.29342159521646,29.3034514706996,-10.2521251320501));
#9434=CARTESIAN_POINT('Ctrl Pts',(-3.16236749142982,29.2624386300888,-10.030803123064));
#9435=CARTESIAN_POINT('Ctrl Pts',(-3.71962300240937,29.2362041996979,-9.83778390824362));
#9436=CARTESIAN_POINT('Ctrl Pts',(-4.74922988451164,29.185618179249,-9.38109078280864));
#9437=CARTESIAN_POINT('Ctrl Pts',(-5.22320775861405,29.1613433504691,-9.12568513083327));
#9438=CARTESIAN_POINT('Ctrl Pts',(-6.21475465024609,29.1074181253387,-8.4887318811753));
#9439=CARTESIAN_POINT('Ctrl Pts',(-6.72112662152996,29.0777157234547,-8.09371285533201));
#9440=CARTESIAN_POINT('Ctrl Pts',(-7.45270245699273,29.0318680506219,-7.40673776204664));
#9441=CARTESIAN_POINT('Ctrl Pts',(-7.70404562399735,29.0155553325848,-7.14494386101737));
#9442=CARTESIAN_POINT('Ctrl Pts',(-8.24398863608406,28.9785163329944,-6.52085947837628));
#9443=CARTESIAN_POINT('Ctrl Pts',(-8.52318560181982,28.95781791939,-6.15144367501544));
#9444=CARTESIAN_POINT('Ctrl Pts',(-9.10012422392409,28.9102582503829,-5.27303831661512));
#9445=CARTESIAN_POINT('Ctrl Pts',(-9.38122216741048,28.883305981918,-4.75497999426468));
#9446=CARTESIAN_POINT('Ctrl Pts',(-9.69612696169593,28.847164576079,-4.03664795901804));
#9447=CARTESIAN_POINT('Ctrl Pts',(-9.76975967869846,28.8381320632105,-3.85502055516978));
#9448=CARTESIAN_POINT('Ctrl Pts',(-9.83826091084007,28.8291247138027,-3.67146064261029));
#9449=CARTESIAN_POINT('Ctrl Pts',(-9.83826088292329,28.0112119827727,-3.67146071741772));
#9450=CARTESIAN_POINT('Ctrl Pts',(-9.63233473390102,28.0382096315146,-4.22327247100276));
#9451=CARTESIAN_POINT('Ctrl Pts',(-9.38031912188069,28.065496103614,-4.75686020923467));
#9452=CARTESIAN_POINT('Ctrl Pts',(-8.90557621356885,28.1087433876724,-5.575793418109));
#9453=CARTESIAN_POINT('Ctrl Pts',(-8.71064440008901,28.1248251234884,-5.87566485887207));
#9454=CARTESIAN_POINT('Ctrl Pts',(-8.22805239493337,28.1617223235901,-6.54109929211968));
#9455=CARTESIAN_POINT('Ctrl Pts',(-7.93065471161723,28.1825071544524,-6.89866199759931));
#9456=CARTESIAN_POINT('Ctrl Pts',(-7.19919120869614,28.230542420745,-7.66805748594574));
#9457=CARTESIAN_POINT('Ctrl Pts',(-6.75167554745295,28.257892170752,-8.06488101351353));
#9458=CARTESIAN_POINT('Ctrl Pts',(-6.02512532181003,28.2996390276788,-8.60606232885609));
#9459=CARTESIAN_POINT('Ctrl Pts',(-5.76934019205613,28.3138825271891,-8.77958769818982));
#9460=CARTESIAN_POINT('Ctrl Pts',(-5.00304875173894,28.3550454604036,-9.25147415735185));
#9461=CARTESIAN_POINT('Ctrl Pts',(-4.47456880442693,28.3813798654994,-9.51832511468678));
#9462=CARTESIAN_POINT('Ctrl Pts',(-3.42852853096244,28.43203473232,-9.94004039354387));
#9463=CARTESIAN_POINT('Ctrl Pts',(-2.91596786447846,28.4562759682461,-10.1022929073331));
#9464=CARTESIAN_POINT('Ctrl Pts',(-1.76698463174089,28.5102728697067,-10.37123329394));
#9465=CARTESIAN_POINT('Ctrl Pts',(-1.12856998007311,28.5400847485167,-10.4599728064787));
#9466=CARTESIAN_POINT('Ctrl Pts',(-0.145070787777347,28.5850553676003,-10.5055452732829));
#9467=CARTESIAN_POINT('Ctrl Pts',(0.196484823710329,28.6004210999214,-10.5047096051333));
#9468=CARTESIAN_POINT('Ctrl Pts',(1.00550151449112,28.636789730861,-10.4632528868762));
#9469=CARTESIAN_POINT('Ctrl Pts',(1.47146700094931,28.6577525681422,-10.407952486264));
#9470=CARTESIAN_POINT('Ctrl Pts',(2.57371132310845,28.7084776633949,-10.2016176558495));
#9471=CARTESIAN_POINT('Ctrl Pts',(3.20264201786382,28.7384108117788,-10.0219776853927));
#9472=CARTESIAN_POINT('Ctrl Pts',(4.0742069902033,28.7815121233764,-9.68254848628005));
#9473=CARTESIAN_POINT('Ctrl Pts',(4.33336691402994,28.7945305032246,-9.56936996621349));
#9474=CARTESIAN_POINT('Ctrl Pts',(4.92101182835283,28.8243737855602,-9.28396417582688));
#9475=CARTESIAN_POINT('Ctrl Pts',(5.2455679906417,28.8410353906497,-9.10452461256677));
#9476=CARTESIAN_POINT('Ctrl Pts',(5.94995049113592,28.8782980508488,-8.6648959961835));
#9477=CARTESIAN_POINT('Ctrl Pts',(6.32352711746613,28.8988747719579,-8.39614989546143));
#9478=CARTESIAN_POINT('Ctrl Pts',(7.1209088982611,28.9456457421507,-7.73903235280749));
#9479=CARTESIAN_POINT('Ctrl Pts',(7.53289270146961,28.9719163864062,-7.33862828664188));
#9480=CARTESIAN_POINT('Ctrl Pts',(8.11829189114373,29.0129279808974,-6.66817273702931));
#9481=CARTESIAN_POINT('Ctrl Pts',(8.31558950329078,29.0275252066665,-6.42044893059705));
#9482=CARTESIAN_POINT('Ctrl Pts',(8.72201361299088,29.0592038169341,-5.85992567878681));
#9483=CARTESIAN_POINT('Ctrl Pts',(8.92613363015351,29.0761303892718,-5.5440412265667));
#9484=CARTESIAN_POINT('Ctrl Pts',(9.34482163716742,29.1139560856039,-4.81281480529713));
#9485=CARTESIAN_POINT('Ctrl Pts',(9.54949020363153,29.1348354722129,-4.39273379914329));
#9486=CARTESIAN_POINT('Ctrl Pts',(9.97137368278544,29.1854419308279,-3.3567262459062));
#9487=CARTESIAN_POINT('Ctrl Pts',(10.1604649521668,29.2153416361926,-2.73144948306346));
#9488=CARTESIAN_POINT('Ctrl Pts',(10.3464009860724,29.2583356301675,-1.81715629618003));
#9489=CARTESIAN_POINT('Ctrl Pts',(10.3913488019078,29.271284666685,-1.53946192602653));
#9490=CARTESIAN_POINT('Ctrl Pts',(10.4657500100949,29.2996015140777,-0.924019887580983));
#9491=CARTESIAN_POINT('Ctrl Pts',(10.4901081552804,29.3148513170999,-0.585977830003707));
#9492=CARTESIAN_POINT('Ctrl Pts',(10.5091543523551,29.3511563112881,0.222412656326963));
#9493=CARTESIAN_POINT('Ctrl Pts',(10.4886797662731,29.3721694805039,0.692376564799234));
#9494=CARTESIAN_POINT('Ctrl Pts',(10.3646502019633,29.4229807083489,1.80889330690969));
#9495=CARTESIAN_POINT('Ctrl Pts',(10.2320267467071,29.4529490877228,2.4502361318087));
#9496=CARTESIAN_POINT('Ctrl Pts',(9.95768563518145,29.4961204860435,3.34601210296476));
#9497=CARTESIAN_POINT('Ctrl Pts',(9.86377048821956,29.5091712328104,3.61349339708788));
#9498=CARTESIAN_POINT('Ctrl Pts',(9.62403962161938,29.5388356072155,4.21696526542007));
#9499=CARTESIAN_POINT('Ctrl Pts',(9.47124289687231,29.5552931414798,4.54977980898371));
#9500=CARTESIAN_POINT('Ctrl Pts',(9.08724967436104,29.5924236753195,5.28258781618324));
#9501=CARTESIAN_POINT('Ctrl Pts',(8.84642545296598,29.6130703647793,5.67667088795452));
#9502=CARTESIAN_POINT('Ctrl Pts',(8.23595657122771,29.6609979484473,6.54195421661666));
#9503=CARTESIAN_POINT('Ctrl Pts',(7.85039218358787,29.6883834983227,6.99996121813689));
#9504=CARTESIAN_POINT('Ctrl Pts',(7.21253448019393,29.7299672068082,7.63827535937103));
#9505=CARTESIAN_POINT('Ctrl Pts',(6.98779898455277,29.7440177658395,7.84439748659218));
#9506=CARTESIAN_POINT('Ctrl Pts',(6.29098588322203,29.7856360743679,8.4297581958081));
#9507=CARTESIAN_POINT('Ctrl Pts',(5.79477555917899,29.8125842367786,8.7782635753352));
#9508=CARTESIAN_POINT('Ctrl Pts',(4.81399661231949,29.863532448144,9.34751391886051));
#9509=CARTESIAN_POINT('Ctrl Pts',(4.33730619892938,29.8874258788524,9.57801309186884));
#9510=CARTESIAN_POINT('Ctrl Pts',(3.24498406131828,29.9411576434858,10.0078599991292));
#9511=CARTESIAN_POINT('Ctrl Pts',(2.62418553411607,29.9710647030443,10.1882688167627));
#9512=CARTESIAN_POINT('Ctrl Pts',(1.58923252694129,30.0191758100296,10.3880982672269));
#9513=CARTESIAN_POINT('Ctrl Pts',(1.18351196804469,30.037513931895,10.4421046784482));
#9514=CARTESIAN_POINT('Ctrl Pts',(0.144862686981982,30.0842356954535,10.5190357669806));
#9515=CARTESIAN_POINT('Ctrl Pts',(-0.4888616783407,30.1126184177228,10.5086673993383));
#9516=CARTESIAN_POINT('Ctrl Pts',(-1.5818551808535,30.1628211623336,10.391658493651));
#9517=CARTESIAN_POINT('Ctrl Pts',(-2.0420945023228,30.1843322759007,10.3110946018329));
#9518=CARTESIAN_POINT('Ctrl Pts',(-2.86060133256157,30.2231445594523,10.1108499331129));
#9519=CARTESIAN_POINT('Ctrl Pts',(-3.22071534644785,30.2403892234578,10.0019666444908));
#9520=CARTESIAN_POINT('Ctrl Pts',(-3.8718038180859,30.2716960682434,9.76628349993863));
#9521=CARTESIAN_POINT('Ctrl Pts',(-4.16436479706541,30.2858726134789,9.64516602787594));
#9522=CARTESIAN_POINT('Ctrl Pts',(-4.9706455322075,30.3258082299518,9.26783910065944));
#9523=CARTESIAN_POINT('Ctrl Pts',(-5.46946745949984,30.3515947339942,8.98248657036646));
#9524=CARTESIAN_POINT('Ctrl Pts',(-6.32152632643401,30.398766799773,8.39765887737398));
#9525=CARTESIAN_POINT('Ctrl Pts',(-6.68307917688397,30.4199437237763,8.11287939219596));
#9526=CARTESIAN_POINT('Ctrl Pts',(-7.30017914791703,30.4581930889483,7.55748934682719));
#9527=CARTESIAN_POINT('Ctrl Pts',(-7.56225810640208,30.4752170860831,7.29524017171136));
#9528=CARTESIAN_POINT('Ctrl Pts',(-7.99890840640804,30.5047981949374,6.80943323918421));
#9529=CARTESIAN_POINT('Ctrl Pts',(-8.17931770227583,30.5174831260515,6.5916372765147));
#9530=CARTESIAN_POINT('Ctrl Pts',(-8.74641206874221,30.5594452052333,5.84783705291626));
#9531=CARTESIAN_POINT('Ctrl Pts',(-9.09285357153411,30.5887101334723,5.29310052074037));
#9532=CARTESIAN_POINT('Ctrl Pts',(-9.59577594160372,30.6399284224677,4.29089399154537));
#9533=CARTESIAN_POINT('Ctrl Pts',(-9.77771090054328,30.6615342781933,3.8583735624167));
#9534=CARTESIAN_POINT('Ctrl Pts',(-10.0411628828821,30.6988431170465,3.09234276004025));
#9535=CARTESIAN_POINT('Ctrl Pts',(-10.1363803408675,30.7145138031143,2.76429783978361));
#9536=CARTESIAN_POINT('Ctrl Pts',(-10.3639128066613,30.7590076115742,1.80863771144074));
#9537=CARTESIAN_POINT('Ctrl Pts',(-10.4549714258374,30.7874695772116,1.17279641167473));
#9538=CARTESIAN_POINT('Ctrl Pts',(-10.5146055243684,30.840554819351,-0.00141240276887271));
#9539=CARTESIAN_POINT('Ctrl Pts',(-10.5008966525229,30.8649396524933,-0.536728397122199));
#9540=CARTESIAN_POINT('Ctrl Pts',(-10.3852276138976,30.9172365074931,-1.66743429855176));
#9541=CARTESIAN_POINT('Ctrl Pts',(-10.2726032240514,30.9450737385028,-2.25985786975737));
#9542=CARTESIAN_POINT('Ctrl Pts',(-10.0309173198126,30.9854842527832,-3.1204009893133));
#9543=CARTESIAN_POINT('Ctrl Pts',(-9.94031035515241,30.9985682311324,-3.3980029798592));
#9544=CARTESIAN_POINT('Ctrl Pts',(-9.83826089557905,31.0116616139851,-3.67146068350461));
#9545=CARTESIAN_POINT('Origin',(0.,20.,0.));
#9546=CARTESIAN_POINT('',(-9.83826090449497,34.8296849384879,-3.671460659613));
#9547=CARTESIAN_POINT('',(-9.83826088462892,34.0117278664922,-3.67146071284722));
#9548=CARTESIAN_POINT('',(-9.83826089695937,20.,-3.67146067980583));
#9549=CARTESIAN_POINT('Ctrl Pts',(-9.83826090449497,34.8296849384879,-3.67146065961299));
#9550=CARTESIAN_POINT('Ctrl Pts',(-9.87013633268989,34.8254908533905,-3.58604539628911));
#9551=CARTESIAN_POINT('Ctrl Pts',(-9.90090469256612,34.8212920122283,-3.5002008550201));
#9552=CARTESIAN_POINT('Ctrl Pts',(-10.0381989019327,34.8018370504582,-3.10083688152188));
#9553=CARTESIAN_POINT('Ctrl Pts',(-10.1309726508253,34.7865611629162,-2.78280827432138));
#9554=CARTESIAN_POINT('Ctrl Pts',(-10.2898789181953,34.7555197163493,-2.12362392381044));
#9555=CARTESIAN_POINT('Ctrl Pts',(-10.3544230567936,34.7398574003433,-1.78250223045051));
#9556=CARTESIAN_POINT('Ctrl Pts',(-10.4679052283791,34.7026484492834,-0.962071396842471));
#9557=CARTESIAN_POINT('Ctrl Pts',(-10.5009950583733,34.6811443202572,-0.481374431363444));
#9558=CARTESIAN_POINT('Ctrl Pts',(-10.5010059971665,34.6329869416597,0.584074227527096));
#9559=CARTESIAN_POINT('Ctrl Pts',(-10.4522641003492,34.6062739922244,1.1672253169037));
#9560=CARTESIAN_POINT('Ctrl Pts',(-10.2712639095788,34.556047637444,2.24239017538735));
#9561=CARTESIAN_POINT('Ctrl Pts',(-10.1512619301906,34.5326917969161,2.73479225064487));
#9562=CARTESIAN_POINT('Ctrl Pts',(-9.79660557440828,34.480295246905,3.83694637694141));
#9563=CARTESIAN_POINT('Ctrl Pts',(-9.5396883845809,34.4513608581882,4.43734175670019));
#9564=CARTESIAN_POINT('Ctrl Pts',(-8.95746364100407,34.3962142269396,5.50983150560361));
#9565=CARTESIAN_POINT('Ctrl Pts',(-8.64600107367251,34.3702280086654,5.98673832377566));
#9566=CARTESIAN_POINT('Ctrl Pts',(-7.98461654538339,34.3205292275213,6.83940487991358));
#9567=CARTESIAN_POINT('Ctrl Pts',(-7.64276005766471,34.296951349283,7.21940490641383));
#9568=CARTESIAN_POINT('Ctrl Pts',(-7.07530876290363,34.2613049116018,7.7644951896326));
#9569=CARTESIAN_POINT('Ctrl Pts',(-6.86851775670562,34.2488991110006,7.94800897823506));
#9570=CARTESIAN_POINT('Ctrl Pts',(-6.14770234010226,34.2070910557485,8.53852227459741));
#9571=CARTESIAN_POINT('Ctrl Pts',(-5.60291145794244,34.1777169263762,8.90550211149995));
#9572=CARTESIAN_POINT('Ctrl Pts',(-4.62018427710503,34.12660652522,9.44140473596752));
#9573=CARTESIAN_POINT('Ctrl Pts',(-4.19861787549921,34.1052293693084,9.63627644832546));
#9574=CARTESIAN_POINT('Ctrl Pts',(-3.43035923345287,34.0673184054502,9.93139337493067));
#9575=CARTESIAN_POINT('Ctrl Pts',(-3.08876700801998,34.0508276702708,10.042881669787));
#9576=CARTESIAN_POINT('Ctrl Pts',(-2.46738715424225,34.021679306244,10.2109748284553));
#9577=CARTESIAN_POINT('Ctrl Pts',(-2.18973698849106,34.008909624726,10.2740966311617));
#9578=CARTESIAN_POINT('Ctrl Pts',(-1.26512575620733,33.9667255212829,10.4451120393492));
#9579=CARTESIAN_POINT('Ctrl Pts',(-0.610648105926783,33.9373179263997,10.5037133309675));
#9580=CARTESIAN_POINT('Ctrl Pts',(0.517447316625793,33.8857764482132,10.4988789282049));
#9581=CARTESIAN_POINT('Ctrl Pts',(0.989214235355772,33.8639920030632,10.4649727950989));
#9582=CARTESIAN_POINT('Ctrl Pts',(1.81725123890417,33.8254891572408,10.3489548272268));
#9583=CARTESIAN_POINT('Ctrl Pts',(2.17456437111616,33.8088198402017,10.2798129469653));
#9584=CARTESIAN_POINT('Ctrl Pts',(2.84004022142136,33.777827180874,10.1147816930769));
#9585=CARTESIAN_POINT('Ctrl Pts',(3.1487755355104,33.7634098659188,10.0229663018507));
#9586=CARTESIAN_POINT('Ctrl Pts',(3.97884962762206,33.7239776381315,9.73396229696878));
#9587=CARTESIAN_POINT('Ctrl Pts',(4.48947632726099,33.6989348997777,9.50925078789113));
#9588=CARTESIAN_POINT('Ctrl Pts',(5.38185766584579,33.6526821209184,9.02857129310746));
#9589=CARTESIAN_POINT('Ctrl Pts',(5.76930053070901,33.6316563254727,8.78604873819855));
#9590=CARTESIAN_POINT('Ctrl Pts',(6.44800700312271,33.5931095733654,8.29690377244693));
#9591=CARTESIAN_POINT('Ctrl Pts',(6.74401474077003,33.5756406005176,8.05814423722092));
#9592=CARTESIAN_POINT('Ctrl Pts',(7.23567168159055,33.5456780391768,7.61546636469039));
#9593=CARTESIAN_POINT('Ctrl Pts',(7.43724914870386,33.5330434761281,7.41873311618829));
#9594=CARTESIAN_POINT('Ctrl Pts',(8.07851750994854,33.4911654907862,6.74043805931232));
#9595=CARTESIAN_POINT('Ctrl Pts',(8.48126699105468,33.4619372844473,6.22607724549495));
#9596=CARTESIAN_POINT('Ctrl Pts',(9.08630087861113,33.4108296182019,5.28472989311774));
#9597=CARTESIAN_POINT('Ctrl Pts',(9.31237542967223,33.3892979492435,4.87533458854948));
#9598=CARTESIAN_POINT('Ctrl Pts',(9.66942584208554,33.3505099838225,4.11264165144949));
#9599=CARTESIAN_POINT('Ctrl Pts',(9.81011440460812,33.3333097001856,3.76474308258486));
#9600=CARTESIAN_POINT('Ctrl Pts',(10.0348042768741,33.302026797313,3.11032660483451));
#9601=CARTESIAN_POINT('Ctrl Pts',(10.1240943721748,33.2878314013858,2.8060907455077));
#9602=CARTESIAN_POINT('Ctrl Pts',(10.3357079403615,33.247928484519,1.94215663404644));
#9603=CARTESIAN_POINT('Ctrl Pts',(10.4262118827604,33.2221934079735,1.37583340133174));
#9604=CARTESIAN_POINT('Ctrl Pts',(10.5053297003632,33.1750835843259,0.346762646039677));
#9605=CARTESIAN_POINT('Ctrl Pts',(10.5104404522202,33.1539157153092,-0.113258737358978));
#9606=CARTESIAN_POINT('Ctrl Pts',(10.4651880088415,33.1156496581278,-0.942605781500887));
#9607=CARTESIAN_POINT('Ctrl Pts',(10.4253514217436,33.098600139274,-1.31176579931775));
#9608=CARTESIAN_POINT('Ctrl Pts',(10.3208952683169,33.0689976127102,-1.95703721848463));
#9609=CARTESIAN_POINT('Ctrl Pts',(10.2644883953892,33.0563160316584,-2.2340893270028));
#9610=CARTESIAN_POINT('Ctrl Pts',(10.041088696114,33.0143605989711,-3.14219107947203));
#9611=CARTESIAN_POINT('Ctrl Pts',(9.82648095911503,32.9850991701866,-3.75993030389822));
#9612=CARTESIAN_POINT('Ctrl Pts',(9.36165983621652,32.9338900091296,-4.78015711496229));
#9613=CARTESIAN_POINT('Ctrl Pts',(9.13905893701823,32.9122897687789,-5.19308853275904));
#9614=CARTESIAN_POINT('Ctrl Pts',(8.70777308487517,32.8749737998869,-5.87898010982293));
#9615=CARTESIAN_POINT('Ctrl Pts',(8.51190435680739,32.8592905508418,-6.15915713765298));
#9616=CARTESIAN_POINT('Ctrl Pts',(7.90966258317944,32.8147389731778,-6.9368857146172));
#9617=CARTESIAN_POINT('Ctrl Pts',(7.47088088258671,32.7862332018928,-7.40736825144903));
#9618=CARTESIAN_POINT('Ctrl Pts',(6.59226331426678,32.7330610427167,-8.19145537949761));
#9619=CARTESIAN_POINT('Ctrl Pts',(6.16595443142408,32.7086342560755,-8.51697476988249));
#9620=CARTESIAN_POINT('Ctrl Pts',(5.21318211352657,32.6563709747048,-9.13531791234831));
#9621=CARTESIAN_POINT('Ctrl Pts',(4.68256757704756,32.6286119105837,-9.41832823497058));
#9622=CARTESIAN_POINT('Ctrl Pts',(3.83812832133132,32.5870875851872,-9.77962272300775));
#9623=CARTESIAN_POINT('Ctrl Pts',(3.5400433955146,32.5728350665806,-9.891427907448));
#9624=CARTESIAN_POINT('Ctrl Pts',(2.69553446102158,32.5330091446118,-10.1651108589706));
#9625=CARTESIAN_POINT('Ctrl Pts',(2.14035208403521,32.5074076986813,-10.296322581333));
#9626=CARTESIAN_POINT('Ctrl Pts',(1.12328449695624,32.4604531191923,-10.4508423149459));
#9627=CARTESIAN_POINT('Ctrl Pts',(0.665255284381629,32.4393021605012,-10.4899617799723));
#9628=CARTESIAN_POINT('Ctrl Pts',(-0.165842753504508,32.4010044834549,-10.5062803531098));
#9629=CARTESIAN_POINT('Ctrl Pts',(-0.537968685621155,32.3839068517497,-10.4938094379395));
#9630=CARTESIAN_POINT('Ctrl Pts',(-1.19007607645678,32.354263738098,-10.4371698539277));
#9631=CARTESIAN_POINT('Ctrl Pts',(-1.47039813209097,32.3415882620907,-10.4013810758494));
#9632=CARTESIAN_POINT('Ctrl Pts',(-2.39225583406765,32.2996444969063,-10.2456711986442));
#9633=CARTESIAN_POINT('Ctrl Pts',(-3.02403528342239,32.2703889992753,-10.0772939761365));
#9634=CARTESIAN_POINT('Ctrl Pts',(-4.07549501224391,32.2191957053056,-9.68920649976376));
#9635=CARTESIAN_POINT('Ctrl Pts',(-4.50355433057597,32.1976053902157,-9.4978087160507));
#9636=CARTESIAN_POINT('Ctrl Pts',(-5.22369264015762,32.1600678617824,-9.11615071658563));
#9637=CARTESIAN_POINT('Ctrl Pts',(-5.52177054628588,32.1441563014154,-8.93874893922606));
#9638=CARTESIAN_POINT('Ctrl Pts',(-6.04824302722397,32.1155373506617,-8.58901609167487));
#9639=CARTESIAN_POINT('Ctrl Pts',(-6.27941783779057,32.1027340047969,-8.42148182420838));
#9640=CARTESIAN_POINT('Ctrl Pts',(-7.01978009718587,32.0604301251586,-7.83748106677449));
#9641=CARTESIAN_POINT('Ctrl Pts',(-7.49667198872497,32.0309341063268,-7.38263550097256));
#9642=CARTESIAN_POINT('Ctrl Pts',(-8.23899565964519,31.9792083802575,-6.52801900409605));
#9643=CARTESIAN_POINT('Ctrl Pts',(-8.52547493261577,31.9573297821157,-6.14917464006969));
#9644=CARTESIAN_POINT('Ctrl Pts',(-8.98229265647638,31.9189310046498,-5.45148389254653));
#9645=CARTESIAN_POINT('Ctrl Pts',(-9.16366221499971,31.9024568708651,-5.14077510401679));
#9646=CARTESIAN_POINT('Ctrl Pts',(-9.47731248523631,31.871579186215,-4.53390107052915));
#9647=CARTESIAN_POINT('Ctrl Pts',(-9.61251774001361,31.8570883740581,-4.23971900875921));
#9648=CARTESIAN_POINT('Ctrl Pts',(-9.76993596611932,31.8382643952994,-3.85078765283611));
#9649=CARTESIAN_POINT('Ctrl Pts',(-9.80471763308074,31.8339581199903,-3.76134517542839));
#9650=CARTESIAN_POINT('Ctrl Pts',(-9.83826093350753,31.8296488111843,-3.67146058186924));
#9651=CARTESIAN_POINT('Ctrl Pts',(-9.83826089557905,31.0116616139852,-3.67146068350461));
#9652=CARTESIAN_POINT('Ctrl Pts',(-9.82914856923431,31.0128307644932,-3.69587860641687));
#9653=CARTESIAN_POINT('Ctrl Pts',(-9.81994500822106,31.0139999610707,-3.72026348698511));
#9654=CARTESIAN_POINT('Ctrl Pts',(-9.60744622470539,31.0407334114432,-4.27699665625298));
#9655=CARTESIAN_POINT('Ctrl Pts',(-9.36124837708719,31.0663477931998,-4.79194460643673));
#9656=CARTESIAN_POINT('Ctrl Pts',(-8.84343503861281,31.1133136620883,-5.68115199578211));
#9657=CARTESIAN_POINT('Ctrl Pts',(-8.58659952399314,31.1344624286705,-6.06235346052566));
#9658=CARTESIAN_POINT('Ctrl Pts',(-8.0779015442922,31.1727642891362,-6.71989865898381));
#9659=CARTESIAN_POINT('Ctrl Pts',(-7.83465925602574,31.1898682421531,-7.00197556762376));
#9660=CARTESIAN_POINT('Ctrl Pts',(-7.38137989219953,31.2195167317468,-7.4743572830578));
#9661=CARTESIAN_POINT('Ctrl Pts',(-7.1776665519123,31.2321914486825,-7.67019504977119));
#9662=CARTESIAN_POINT('Ctrl Pts',(-6.47812054187384,31.2741338280966,-8.29039217655118));
#9663=CARTESIAN_POINT('Ctrl Pts',(-5.95067359768883,31.303388653166,-8.67675682070298));
#9664=CARTESIAN_POINT('Ctrl Pts',(-4.98887166047795,31.3545800935956,-9.25210887203168));
#9665=CARTESIAN_POINT('Ctrl Pts',(-4.57130897831263,31.376169227222,-9.4653834087176));
#9666=CARTESIAN_POINT('Ctrl Pts',(-3.79868502152885,31.4148918552883,-9.7969219746833));
#9667=CARTESIAN_POINT('Ctrl Pts',(-3.44887523636577,31.4319707435522,-9.92547051903154));
#9668=CARTESIAN_POINT('Ctrl Pts',(-2.78894922061205,31.4631908145377,-10.1288681297488));
#9669=CARTESIAN_POINT('Ctrl Pts',(-2.48082846589552,31.4774403983092,-10.2087071239348));
#9670=CARTESIAN_POINT('Ctrl Pts',(-1.61221589782715,31.5172671051568,-10.392123979522));
#9671=CARTESIAN_POINT('Ctrl Pts',(-1.04623331237099,31.5428722241993,-10.4642657505441));
#9672=CARTESIAN_POINT('Ctrl Pts',(-0.0184858863972343,31.5898300287755,
-10.51101897649));
#9673=CARTESIAN_POINT('Ctrl Pts',(0.44110533347316,31.6109803849648,-10.5017749605602));
#9674=CARTESIAN_POINT('Ctrl Pts',(1.26933972814084,31.6492792475791,-10.4306392692086));
#9675=CARTESIAN_POINT('Ctrl Pts',(1.63813055474911,31.66637865205,-10.379113803606));
#9676=CARTESIAN_POINT('Ctrl Pts',(2.28070312194509,31.696023293501,-10.254227734207));
#9677=CARTESIAN_POINT('Ctrl Pts',(2.55570528502207,31.7086985765141,-10.1891691013496));
#9678=CARTESIAN_POINT('Ctrl Pts',(3.45607871398569,31.75064201096,-9.93741325689512));
#9679=CARTESIAN_POINT('Ctrl Pts',(4.0666539501315,31.7798973590637,-9.70355424353691));
#9680=CARTESIAN_POINT('Ctrl Pts',(5.07148209200513,31.8310902257058,-9.20708673399526));
#9681=CARTESIAN_POINT('Ctrl Pts',(5.47704407566804,31.8526802623373,-8.97175315950559));
#9682=CARTESIAN_POINT('Ctrl Pts',(6.15308232009437,31.8902184156435,-8.51649927806003));
#9683=CARTESIAN_POINT('Ctrl Pts',(6.43087446562323,31.9061308667628,-8.30873332574524));
#9684=CARTESIAN_POINT('Ctrl Pts',(6.91767933539055,31.9347507915758,-7.90557746905667));
#9685=CARTESIAN_POINT('Ctrl Pts',(7.12996222725988,31.9475542432224,-7.71466684323086));
#9686=CARTESIAN_POINT('Ctrl Pts',(7.80483323400902,31.9898585540256,-7.05606191798188));
#9687=CARTESIAN_POINT('Ctrl Pts',(8.23126914646099,32.019354905531,-6.55359562378533));
#9688=CARTESIAN_POINT('Ctrl Pts',(8.87964062679311,32.0710813188298,-5.62566181671774));
#9689=CARTESIAN_POINT('Ctrl Pts',(9.12470734527588,32.0929602648956,-5.21879242579634));
#9690=CARTESIAN_POINT('Ctrl Pts',(9.50567038337168,32.131361794661,-4.47688803501034));
#9691=CARTESIAN_POINT('Ctrl Pts',(9.65338821463603,32.1478382856922,-4.14878388954857));
#9692=CARTESIAN_POINT('Ctrl Pts',(9.90154503783663,32.1787229375254,-3.51214808074365));
#9693=CARTESIAN_POINT('Ctrl Pts',(10.0050968633687,32.1932183520988,-3.20527982364734));
#9694=CARTESIAN_POINT('Ctrl Pts',(10.2472581585438,32.2326382453562,-2.36065233089806));
#9695=CARTESIAN_POINT('Ctrl Pts',(10.3576746050566,32.2575915458213,-1.81591241339751));
#9696=CARTESIAN_POINT('Ctrl Pts',(10.4795777665442,32.3037695734767,-0.811350842455702));
#9697=CARTESIAN_POINT('Ctrl Pts',(10.5049559575086,32.3248137670466,-0.354584559319434));
#9698=CARTESIAN_POINT('Ctrl Pts',(10.4968081321095,32.3633222300471,0.481156570536684));
#9699=CARTESIAN_POINT('Ctrl Pts',(10.4726219990081,32.3807349184809,0.859475314857011));
#9700=CARTESIAN_POINT('Ctrl Pts',(10.3524566095498,32.4269837209511,1.87357430956689));
#9701=CARTESIAN_POINT('Ctrl Pts',(10.218494273624,32.4555067655601,2.50320456839082));
#9702=CARTESIAN_POINT('Ctrl Pts',(9.8684212966746,32.5087677590744,3.62956853112552));
#9703=CARTESIAN_POINT('Ctrl Pts',(9.66988908326435,32.5332666402691,4.12949488227611));
#9704=CARTESIAN_POINT('Ctrl Pts',(9.17479296395958,32.5851389791878,5.14222437862356));
#9705=CARTESIAN_POINT('Ctrl Pts',(8.87134937579214,32.612432630889,5.6496459768974));
#9706=CARTESIAN_POINT('Ctrl Pts',(8.34676654387113,32.6530835281836,6.37947658030121));
#9707=CARTESIAN_POINT('Ctrl Pts',(8.15569412326338,32.6669120266757,6.62200046351361));
#9708=CARTESIAN_POINT('Ctrl Pts',(7.56363032744996,32.7075935652371,7.30892723128319));
#9709=CARTESIAN_POINT('Ctrl Pts',(7.13503867239633,32.7344713677619,7.7278795958213));
#9710=CARTESIAN_POINT('Ctrl Pts',(6.3141700865968,32.7830185034957,8.40347411311074));
#9711=CARTESIAN_POINT('Ctrl Pts',(5.93600229268122,32.8044417796721,8.6747327087716));
#9712=CARTESIAN_POINT('Ctrl Pts',(5.23817701280554,32.8422829902838,9.10822087290215));
#9713=CARTESIAN_POINT('Ctrl Pts',(4.925840367004,32.8586591790379,9.28085650042046));
#9714=CARTESIAN_POINT('Ctrl Pts',(4.34907050639899,32.8877191716683,9.56231593541395));
#9715=CARTESIAN_POINT('Ctrl Pts',(4.08783385110028,32.9005116248716,9.6768754295446));
#9716=CARTESIAN_POINT('Ctrl Pts',(3.21039784566193,32.9427746911704,10.0197751212775));
#9717=CARTESIAN_POINT('Ctrl Pts',(2.57746250091129,32.9722400284041,10.2009416604426));
#9718=CARTESIAN_POINT('Ctrl Pts',(1.46610156997011,33.0239024017958,10.4089379546954));
#9719=CARTESIAN_POINT('Ctrl Pts',(0.995073406961301,33.0457489264139,10.4644761951211));
#9720=CARTESIAN_POINT('Ctrl Pts',(0.161400278282493,33.0841841243111,10.505962333541));
#9721=CARTESIAN_POINT('Ctrl Pts',(-0.199811410660965,33.1007256701809,10.5053027578804));
#9722=CARTESIAN_POINT('Ctrl Pts',(-0.882888888169412,33.1316454499507,10.4688051310715));
#9723=CARTESIAN_POINT('Ctrl Pts',(-1.20453184458581,33.1461132205511,10.4366891497265));
#9724=CARTESIAN_POINT('Ctrl Pts',(-2.07398367875824,33.1855374088523,10.309140500572));
#9725=CARTESIAN_POINT('Ctrl Pts',(-2.61650358109148,33.2105223051167,10.1849731014887));
#9726=CARTESIAN_POINT('Ctrl Pts',(-3.58249896810754,33.256726705187,9.88156959161748));
#9727=CARTESIAN_POINT('Ctrl Pts',(-4.00895679594617,33.2777643661218,9.7163764531419));
#9728=CARTESIAN_POINT('Ctrl Pts',(-4.76723691466898,33.316286372409,9.36420141374558));
#9729=CARTESIAN_POINT('Ctrl Pts',(-5.10228556222887,33.333718992615,9.18594114613759));
#9730=CARTESIAN_POINT('Ctrl Pts',(-5.97535648448704,33.3799056759568,8.65889387582258));
#9731=CARTESIAN_POINT('Ctrl Pts',(-6.4923125805193,33.408349982469,8.27835885360256));
#9732=CARTESIAN_POINT('Ctrl Pts',(-7.37171386237732,33.4614452932092,7.4976942647904));
#9733=CARTESIAN_POINT('Ctrl Pts',(-7.74428822663554,33.4858591201902,7.11221209581097));
#9734=CARTESIAN_POINT('Ctrl Pts',(-8.46914763228307,33.5381329977369,6.23742406866072));
#9735=CARTESIAN_POINT('Ctrl Pts',(-8.81206575181795,33.5659164259542,5.74277481701839));
#9736=CARTESIAN_POINT('Ctrl Pts',(-9.2689969616897,33.6074613392789,4.94549340146927));
#9737=CARTESIAN_POINT('Ctrl Pts',(-9.41456188314599,33.6217110837854,4.66242832467283));
#9738=CARTESIAN_POINT('Ctrl Pts',(-9.78427601634383,33.6615377487643,3.8553104295076));
#9739=CARTESIAN_POINT('Ctrl Pts',(-9.97896367270501,33.6871426677592,3.31899693066528));
#9740=CARTESIAN_POINT('Ctrl Pts',(-10.2503031528505,33.7341002981444,2.32661719717631));
#9741=CARTESIAN_POINT('Ctrl Pts',(-10.3422270835954,33.7552506886358,1.87621716340056));
#9742=CARTESIAN_POINT('Ctrl Pts',(-10.4547369383482,33.7935494866052,1.05258391474129));
#9743=CARTESIAN_POINT('Ctrl Pts',(-10.4854686962397,33.8106487929695,0.681483470410139));
#9744=CARTESIAN_POINT('Ctrl Pts',(-10.5047634388197,33.8402933514364,0.0271736341898603));
#9745=CARTESIAN_POINT('Ctrl Pts',(-10.5016934800972,33.8529686466748,-0.255402988241976));
#9746=CARTESIAN_POINT('Ctrl Pts',(-10.4538383790911,33.894912103948,-1.18908610520262));
#9747=CARTESIAN_POINT('Ctrl Pts',(-10.3597932795764,33.9241674633898,-1.83611623213397));
#9748=CARTESIAN_POINT('Ctrl Pts',(-10.1077088029461,33.973114734744,-2.87766610130898));
#9749=CARTESIAN_POINT('Ctrl Pts',(-9.98479584838443,33.9924154610121,-3.27879705254936));
#9750=CARTESIAN_POINT('Ctrl Pts',(-9.83826088462892,34.0117278664922,-3.67146071284722));
#9751=CARTESIAN_POINT('Origin',(0.,20.,0.));
#9752=CARTESIAN_POINT('',(-9.83826089695936,37.8294631792708,-3.67146067980585));
#9753=CARTESIAN_POINT('',(-9.83826083089393,37.0111767992967,-3.67146085683862));
#9754=CARTESIAN_POINT('',(-9.83826089695937,20.,-3.67146067980583));
#9755=CARTESIAN_POINT('',(-10.5009999970343,37.6589303301852,0.000249570010058437));
#9756=CARTESIAN_POINT('Ctrl Pts',(-10.5009999970343,37.6589303301852,0.000249570010072427));
#9757=CARTESIAN_POINT('Ctrl Pts',(-10.5010060172308,37.6704494325525,-0.253058443389185));
#9758=CARTESIAN_POINT('Ctrl Pts',(-10.4918421461636,37.6819685349198,-0.506402163384309));
#9759=CARTESIAN_POINT('Ctrl Pts',(-10.4735267137384,37.6934876372871,-0.759104193512294));
#9760=CARTESIAN_POINT('Ctrl Pts',(-10.4552121477138,37.7050061947502,-1.01179426972174));
#9761=CARTESIAN_POINT('Ctrl Pts',(-10.4277469013743,37.7165247522132,-1.26384243591084));
#9762=CARTESIAN_POINT('Ctrl Pts',(-10.39120133153,37.7280433096763,-1.51457449061109));
#9763=CARTESIAN_POINT('Ctrl Pts',(-10.3546588348145,37.7395608985401,-1.76528546117186));
#9764=CARTESIAN_POINT('Ctrl Pts',(-10.3090375811287,37.751078487404,-2.014680263077));
#9765=CARTESIAN_POINT('Ctrl Pts',(-10.2544595205487,37.7625960762678,-2.26209216024217));
#9766=CARTESIAN_POINT('Ctrl Pts',(-10.1998725596876,37.7741155433548,-2.50954440393833));
#9767=CARTESIAN_POINT('Ctrl Pts',(-10.1363259314528,37.7856350104418,-2.75501282140218));
#9768=CARTESIAN_POINT('Ctrl Pts',(-10.0639925248397,37.7971544775288,-2.99784180035765));
#9769=CARTESIAN_POINT('Ctrl Pts',(-9.99636791331339,37.8079240447762,-3.22486298099979));
#9770=CARTESIAN_POINT('Ctrl Pts',(-9.92106382279401,37.8186936120235,-3.44957711398867));
#9771=CARTESIAN_POINT('Ctrl Pts',(-9.83826089695936,37.8294631792708,-3.67146067980586));
#9772=CARTESIAN_POINT('Ctrl Pts',(-10.5009999972296,37.6587489740896,0.000241215157813779));
#9773=CARTESIAN_POINT('Ctrl Pts',(-10.5009931671448,37.6450509232821,0.297580407341688));
#9774=CARTESIAN_POINT('Ctrl Pts',(-10.4883574507233,37.6313755496597,0.594788982950907));
#9775=CARTESIAN_POINT('Ctrl Pts',(-10.4177560221554,37.5935121766817,1.42381184909578));
#9776=CARTESIAN_POINT('Ctrl Pts',(-10.3317628358919,37.5696958577354,1.95232579157638));
#9777=CARTESIAN_POINT('Ctrl Pts',(-10.0830089073701,37.5222180834809,2.97933311726381));
#9778=CARTESIAN_POINT('Ctrl Pts',(-9.92246895061352,37.4986285760186,3.47679235254345));
#9779=CARTESIAN_POINT('Ctrl Pts',(-9.48366771275629,37.445376966917,4.55440652484981));
#9780=CARTESIAN_POINT('Ctrl Pts',(-9.18778777907868,37.4156408468801,5.12514538123641));
#9781=CARTESIAN_POINT('Ctrl Pts',(-8.64388992816215,37.3696030268651,5.97399188297625));
#9782=CARTESIAN_POINT('Ctrl Pts',(-8.43007051008348,37.3531237094165,6.27210706359289));
#9783=CARTESIAN_POINT('Ctrl Pts',(-7.91428582619626,37.3160624723504,6.91707765044198));
#9784=CARTESIAN_POINT('Ctrl Pts',(-7.6042648243848,37.2955066648173,7.25651669786153));
#9785=CARTESIAN_POINT('Ctrl Pts',(-6.86216294971548,37.2489348923546,7.96907545431884));
#9786=CARTESIAN_POINT('Ctrl Pts',(-6.41989159324911,37.2228467037766,8.32949030318713));
#9787=CARTESIAN_POINT('Ctrl Pts',(-5.68843780410364,37.1819424163878,8.83254825725357));
#9788=CARTESIAN_POINT('Ctrl Pts',(-5.41822249890715,37.1672686695633,9.0008388875092));
#9789=CARTESIAN_POINT('Ctrl Pts',(-4.61698912534079,37.1252235735471,9.45067465024983));
#9790=CARTESIAN_POINT('Ctrl Pts',(-4.06893898855017,37.0984585533248,9.69925685163864));
#9791=CARTESIAN_POINT('Ctrl Pts',(-2.99791507425247,37.0474310088776,10.0782011499541));
#9792=CARTESIAN_POINT('Ctrl Pts',(-2.48028825814185,37.0232531232271,10.2179148112985));
#9793=CARTESIAN_POINT('Ctrl Pts',(-1.3247524020341,36.9694343513984,10.4367885293251));
#9794=CARTESIAN_POINT('Ctrl Pts',(-0.685640791880849,36.939738817857,10.4981620912132));
#9795=CARTESIAN_POINT('Ctrl Pts',(0.335063923662304,36.8931136972875,10.5025299849476));
#9796=CARTESIAN_POINT('Ctrl Pts',(0.714866487983967,36.8760381714026,10.4835286885906));
#9797=CARTESIAN_POINT('Ctrl Pts',(1.54694157984521,36.8384971023869,10.3964640262963));
#9798=CARTESIAN_POINT('Ctrl Pts',(1.99748379721537,36.8180526336035,10.3193771823113));
#9799=CARTESIAN_POINT('Ctrl Pts',(2.98332707116183,36.7721575552213,10.0837012783703));
#9800=CARTESIAN_POINT('Ctrl Pts',(3.51390673322399,36.746646284169,9.91129184004001));
#9801=CARTESIAN_POINT('Ctrl Pts',(4.32559075883288,36.7061501330183,9.5741268055798));
#9802=CARTESIAN_POINT('Ctrl Pts',(4.61705629253519,36.6913012439449,9.43702458443572));
#9803=CARTESIAN_POINT('Ctrl Pts',(5.22340538795978,36.6599241217061,9.11697935372812));
#9804=CARTESIAN_POINT('Ctrl Pts',(5.53600520905962,36.6435290477408,8.9306173899538));
#9805=CARTESIAN_POINT('Ctrl Pts',(6.23101235461873,36.605982894881,8.46573646258003));
#9806=CARTESIAN_POINT('Ctrl Pts',(6.6055336342901,36.5848593384056,8.17686556556475));
#9807=CARTESIAN_POINT('Ctrl Pts',(7.45036901534075,36.5338405387999,7.42919717806922));
#9808=CARTESIAN_POINT('Ctrl Pts',(7.8996172681901,36.5037756079646,6.94960252920526));
#9809=CARTESIAN_POINT('Ctrl Pts',(8.47548669597734,36.460445537834,6.20629675579876));
#9810=CARTESIAN_POINT('Ctrl Pts',(8.64056751757498,36.4473377495159,5.97432755210562));
#9811=CARTESIAN_POINT('Ctrl Pts',(8.99222503301976,36.4179250758232,5.43506312840404));
#9812=CARTESIAN_POINT('Ctrl Pts',(9.17285809141486,36.4017657998048,5.12432436372973));
#9813=CARTESIAN_POINT('Ctrl Pts',(9.54947404862761,36.3648216195109,4.39246296582987));
#9814=CARTESIAN_POINT('Ctrl Pts',(9.73416502573225,36.3440663805361,3.96638526046115));
#9815=CARTESIAN_POINT('Ctrl Pts',(10.0914118035039,36.295970740073,2.96533666616792));
#9816=CARTESIAN_POINT('Ctrl Pts',(10.2440998739793,36.2685274735933,2.3849947684543));
#9817=CARTESIAN_POINT('Ctrl Pts',(10.3989541809779,36.2267776026196,1.49231921162564));
#9818=CARTESIAN_POINT('Ctrl Pts',(10.4381388239824,36.212623356528,1.18765527177303));
#9819=CARTESIAN_POINT('Ctrl Pts',(10.5131583355003,36.1717595586685,0.297343632478159));
#9820=CARTESIAN_POINT('Ctrl Pts',(10.513360776764,36.1456246276376,-0.290111434756389));
#9821=CARTESIAN_POINT('Ctrl Pts',(10.4196825005028,36.0951066353059,-1.41106751099651));
#9822=CARTESIAN_POINT('Ctrl Pts',(10.333645272681,36.0707979122,-1.94336046620219));
#9823=CARTESIAN_POINT('Ctrl Pts',(10.0568119201155,36.0168739070513,-3.08889598606517));
#9824=CARTESIAN_POINT('Ctrl Pts',(9.84987484321755,35.9872087190027,-3.69603793676894));
#9825=CARTESIAN_POINT('Ctrl Pts',(9.44458832182835,35.9417823433404,-4.60392992676662));
#9826=CARTESIAN_POINT('Ctrl Pts',(9.28396371067778,35.9258453826508,-4.91980086565283));
#9827=CARTESIAN_POINT('Ctrl Pts',(8.87578105869489,35.8890342822107,-5.63103608956011));
#9828=CARTESIAN_POINT('Ctrl Pts',(8.6172471334104,35.8681926938872,-6.01922787277115));
#9829=CARTESIAN_POINT('Ctrl Pts',(7.93718123420258,35.8176213233452,-6.90630879524323));
#9830=CARTESIAN_POINT('Ctrl Pts',(7.49326434197177,35.7877175010241,-7.38558709812607));
#9831=CARTESIAN_POINT('Ctrl Pts',(6.7990631115209,35.74476429676,-8.00764005631805));
#9832=CARTESIAN_POINT('Ctrl Pts',(6.58291778086649,35.7318578329585,-8.18625399876423));
#9833=CARTESIAN_POINT('Ctrl Pts',(6.08774374670913,35.7034345248684,-8.56313850062324));
#9834=CARTESIAN_POINT('Ctrl Pts',(5.80565073700636,35.6880405800981,-8.75684803972511));
#9835=CARTESIAN_POINT('Ctrl Pts',(5.11595898167302,35.6516562161267,-9.18245043650225));
#9836=CARTESIAN_POINT('Ctrl Pts',(4.7013057683148,35.6307053974818,-9.40149733726477));
#9837=CARTESIAN_POINT('Ctrl Pts',(3.6773831583457,35.5799996353671,-9.8576683107361));
#9838=CARTESIAN_POINT('Ctrl Pts',(3.05790661175083,35.5500736248345,-10.0670719907663));
#9839=CARTESIAN_POINT('Ctrl Pts',(2.14816247853522,35.5069886249336,-10.2828110046282));
#9840=CARTESIAN_POINT('Ctrl Pts',(1.87077042196794,35.4939788034298,-10.3368769361586));
#9841=CARTESIAN_POINT('Ctrl Pts',(1.22388011677837,35.4640826408215,-10.4360656513436));
#9842=CARTESIAN_POINT('Ctrl Pts',(0.853495917054556,35.4473616985031,-10.4728648086759));
#9843=CARTESIAN_POINT('Ctrl Pts',(0.0231684158759233,35.4100599734809,-10.5110119369182));
#9844=CARTESIAN_POINT('Ctrl Pts',(-0.436478849810725,35.3895029968399,-10.5019707519977));
#9845=CARTESIAN_POINT('Ctrl Pts',(-1.46130585503684,35.3429427133106,-10.4143992646476));
#9846=CARTESIAN_POINT('Ctrl Pts',(-2.02366631855655,35.3168675595913,-10.3198776322952));
#9847=CARTESIAN_POINT('Ctrl Pts',(-2.88423401563315,35.2759662593278,-10.1021564200989));
#9848=CARTESIAN_POINT('Ctrl Pts',(-3.18918480192251,35.2612824842756,-10.0100685736161));
#9849=CARTESIAN_POINT('Ctrl Pts',(-4.05388845964617,35.2193317474278,-9.70541537184412));
#9850=CARTESIAN_POINT('Ctrl Pts',(-4.60025503841201,35.1926655424663,-9.4586870525714));
#9851=CARTESIAN_POINT('Ctrl Pts',(-5.59105010693511,35.1416887258416,-8.90500339111274));
#9852=CARTESIAN_POINT('Ctrl Pts',(-6.03869717872041,35.1174588941208,-8.6077315681033));
#9853=CARTESIAN_POINT('Ctrl Pts',(-6.96717991364704,35.063560127356,-7.88293660805527));
#9854=CARTESIAN_POINT('Ctrl Pts',(-7.4354860049986,35.0338372604638,-7.44283682841304));
#9855=CARTESIAN_POINT('Ctrl Pts',(-8.10849382247395,34.9874710629029,-6.68303683256363));
#9856=CARTESIAN_POINT('Ctrl Pts',(-8.34116654542886,34.970673078064,-6.39027369024781));
#9857=CARTESIAN_POINT('Ctrl Pts',(-8.82355171872713,34.9333201812836,-5.71194377016188));
#9858=CARTESIAN_POINT('Ctrl Pts',(-9.06458373155467,34.9127884207058,-5.32115429414048));
#9859=CARTESIAN_POINT('Ctrl Pts',(-9.49243924227483,34.8714136217851,-4.51352483129694));
#9860=CARTESIAN_POINT('Ctrl Pts',(-9.67914359682593,34.8506211757911,-4.09784071169662));
#9861=CARTESIAN_POINT('Ctrl Pts',(-9.83826090449496,34.8296849384879,-3.671460659613));
#9862=CARTESIAN_POINT('Ctrl Pts',(-9.83826088462892,34.0117278664922,-3.67146071284722));
#9863=CARTESIAN_POINT('Ctrl Pts',(-9.82107553834802,34.01399278926,-3.71751157198144));
#9864=CARTESIAN_POINT('Ctrl Pts',(-9.80356528834997,34.0162576204145,-3.76344598199641));
#9865=CARTESIAN_POINT('Ctrl Pts',(-9.65997591879196,34.0344885301241,-4.13231731106991));
#9866=CARTESIAN_POINT('Ctrl Pts',(-9.51829653611892,34.0504009223036,-4.44895786013873));
#9867=CARTESIAN_POINT('Ctrl Pts',(-9.23190495344731,34.0790207844127,-5.01242190650544));
#9868=CARTESIAN_POINT('Ctrl Pts',(-9.09228079640018,34.0918242307828,-5.26145186382657));
#9869=CARTESIAN_POINT('Ctrl Pts',(-8.59798323113089,34.1341285213107,-6.06449631212284));
#9870=CARTESIAN_POINT('Ctrl Pts',(-8.20144663832499,34.1636248574456,-6.5908785424878));
#9871=CARTESIAN_POINT('Ctrl Pts',(-7.43857670499025,34.2153512391263,-7.42722457068528));
#9872=CARTESIAN_POINT('Ctrl Pts',(-7.09546775876342,34.2372301692476,-7.75566989286965));
#9873=CARTESIAN_POINT('Ctrl Pts',(-6.4553518203272,34.2756317152955,-8.2902792038028));
#9874=CARTESIAN_POINT('Ctrl Pts',(-6.16770279300873,34.2921082380427,-8.50645369867616));
#9875=CARTESIAN_POINT('Ctrl Pts',(-5.60111594826016,34.3229929066519,-8.88837882906752));
#9876=CARTESIAN_POINT('Ctrl Pts',(-5.32448466339852,34.3374883074028,-9.0568010279565));
#9877=CARTESIAN_POINT('Ctrl Pts',(-4.55366832272441,34.376908202781,-9.47855919454229));
#9878=CARTESIAN_POINT('Ctrl Pts',(-4.04648081827942,34.4018615190202,-9.70592368130221));
#9879=CARTESIAN_POINT('Ctrl Pts',(-3.09322247052688,34.4480395598217,-10.0454872972977));
#9880=CARTESIAN_POINT('Ctrl Pts',(-2.65318347112359,34.46908375011,-10.1705676972919));
#9881=CARTESIAN_POINT('Ctrl Pts',(-1.83605970106974,34.5075922198815,-10.3461769530387));
#9882=CARTESIAN_POINT('Ctrl Pts',(-1.46166637200327,34.5250049182953,-10.4056734971707));
#9883=CARTESIAN_POINT('Ctrl Pts',(-0.447842327974835,34.5711669666702,-10.5109760815768));
#9884=CARTESIAN_POINT('Ctrl Pts',(0.193906747451343,34.5996062622448,-10.5187261956888));
#9885=CARTESIAN_POINT('Ctrl Pts',(1.36593990272974,34.6526930442481,-10.4255319750211));
#9886=CARTESIAN_POINT('Ctrl Pts',(1.89548321630696,34.677103510136,-10.3423705523182));
#9887=CARTESIAN_POINT('Ctrl Pts',(3.00113641060863,34.7293801120193,-10.0809355232661));
#9888=CARTESIAN_POINT('Ctrl Pts',(3.57298191992697,34.75716983612,-9.89272084778132));
#9889=CARTESIAN_POINT('Ctrl Pts',(4.41813422754015,34.7987200223659,-9.53164668932002));
#9890=CARTESIAN_POINT('Ctrl Pts',(4.70484309408987,34.8129690032317,-9.39343674045633));
#9891=CARTESIAN_POINT('Ctrl Pts',(5.48621139839481,34.8527958671224,-8.97201120350292));
#9892=CARTESIAN_POINT('Ctrl Pts',(5.96474156420531,34.8784017365229,-8.66125507940379));
#9893=CARTESIAN_POINT('Ctrl Pts',(6.77922211186451,34.925360194481,-8.03268365815304));
#9894=CARTESIAN_POINT('Ctrl Pts',(7.12395001650136,34.9465104220155,-7.7285952760906));
#9895=CARTESIAN_POINT('Ctrl Pts',(7.70998674334918,34.9848095270804,-7.13901738239864));
#9896=CARTESIAN_POINT('Ctrl Pts',(7.95810712087114,35.001909299506,-6.86134184945294));
#9897=CARTESIAN_POINT('Ctrl Pts',(8.36772949891579,35.0315542520744,-6.35073976792056));
#9898=CARTESIAN_POINT('Ctrl Pts',(8.53552910504756,35.0442294891182,-6.12336008969783));
#9899=CARTESIAN_POINT('Ctrl Pts',(9.05987166239957,35.086172837601,-5.34933515696538));
#9900=CARTESIAN_POINT('Ctrl Pts',(9.37464318187299,35.1154281429425,-4.77626458284983));
#9901=CARTESIAN_POINT('Ctrl Pts',(9.82053445804387,35.1666208932384,-3.74799656513446));
#9902=CARTESIAN_POINT('Ctrl Pts',(9.97791192030554,35.1882108563075,-3.30630289440341));
#9903=CARTESIAN_POINT('Ctrl Pts',(10.1995496528347,35.2257491612139,-2.52197783212394));
#9904=CARTESIAN_POINT('Ctrl Pts',(10.2772472934879,35.2416618343669,-2.18389268400027));
#9905=CARTESIAN_POINT('Ctrl Pts',(10.3881555855434,35.2702819956406,-1.56162296899322));
#9906=CARTESIAN_POINT('Ctrl Pts',(10.4267570454005,35.283085467408,-1.2787429923918));
#9907=CARTESIAN_POINT('Ctrl Pts',(10.5160749685079,35.325389855962,-0.340000797934821));
#9908=CARTESIAN_POINT('Ctrl Pts',(10.5167309121742,35.3548862665161,0.319029727509173));
#9909=CARTESIAN_POINT('Ctrl Pts',(10.4117576583452,35.4066128012676,1.44616465904065));
#9910=CARTESIAN_POINT('Ctrl Pts',(10.3357994845268,35.4284918085721,1.91502709021752));
#9911=CARTESIAN_POINT('Ctrl Pts',(10.1470053802454,35.466893275827,2.72737526988958));
#9912=CARTESIAN_POINT('Ctrl Pts',(10.0476700661485,35.4833696450731,3.07321267737527));
#9913=CARTESIAN_POINT('Ctrl Pts',(9.82557113631646,35.5142542319246,3.71939926495458));
#9914=CARTESIAN_POINT('Ctrl Pts',(9.70625756771215,35.5287496990205,4.02049086457001));
#9915=CARTESIAN_POINT('Ctrl Pts',(9.34515643256911,35.5681695839986,4.82151728307303));
#9916=CARTESIAN_POINT('Ctrl Pts',(9.077344045512,35.5931228243038,5.30855768187026));
#9917=CARTESIAN_POINT('Ctrl Pts',(8.52111097531407,35.6393008014113,6.15390187850402));
#9918=CARTESIAN_POINT('Ctrl Pts',(8.24526505777467,35.6603450070749,6.51885221762408));
#9919=CARTESIAN_POINT('Ctrl Pts',(7.69890254694489,35.6988534447153,7.15132096731503));
#9920=CARTESIAN_POINT('Ctrl Pts',(7.43593714038595,35.7162660959639,7.42437523245819));
#9921=CARTESIAN_POINT('Ctrl Pts',(6.95270705750426,35.7461795903885,7.87465608880977));
#9922=CARTESIAN_POINT('Ctrl Pts',(6.73898304516037,35.7588197397611,8.05831587719436));
#9923=CARTESIAN_POINT('Ctrl Pts',(6.00699561721915,35.8007055181527,8.63782479840948));
#9924=CARTESIAN_POINT('Ctrl Pts',(5.45929559545112,35.829936257828,8.99400258021143));
#9925=CARTESIAN_POINT('Ctrl Pts',(4.46839230002774,35.8810536570763,9.51434949451566));
#9926=CARTESIAN_POINT('Ctrl Pts',(4.04062426561489,35.9025926050085,9.70374780135818));
#9927=CARTESIAN_POINT('Ctrl Pts',(3.24974289814775,35.9413721257924,9.99252423901558));
#9928=CARTESIAN_POINT('Ctrl Pts',(2.8911756253112,35.9585568610987,10.1021032799281));
#9929=CARTESIAN_POINT('Ctrl Pts',(2.21977424548672,35.9898315369082,10.2685991161173));
#9930=CARTESIAN_POINT('Ctrl Pts',(1.90873810723697,36.0040336957253,10.3309364538006));
#9931=CARTESIAN_POINT('Ctrl Pts',(1.02984421106209,36.0439251099452,10.4660299115486));
#9932=CARTESIAN_POINT('Ctrl Pts',(0.458184335963544,36.0696419646578,10.5065888423917));
#9933=CARTESIAN_POINT('Ctrl Pts',(-0.573387406794513,36.1167298271369,10.4953972652735));
#9934=CARTESIAN_POINT('Ctrl Pts',(-1.032028171556,36.1378945809863,10.4602602415402));
#9935=CARTESIAN_POINT('Ctrl Pts',(-1.85436440864884,36.1761664768795,10.3426369619515));
#9936=CARTESIAN_POINT('Ctrl Pts',(-2.21881118676237,36.1932248717734,10.2706231398251));
#9937=CARTESIAN_POINT('Ctrl Pts',(-2.85262671330958,36.2228348974054,10.1100633213754));
#9938=CARTESIAN_POINT('Ctrl Pts',(-3.12365628849769,36.2355153632179,10.029637792301));
#9939=CARTESIAN_POINT('Ctrl Pts',(-4.0086830890575,36.2774686554225,9.72765425242399));
#9940=CARTESIAN_POINT('Ctrl Pts',(-4.60525566416108,36.3067289912895,9.45983057912808));
#9941=CARTESIAN_POINT('Ctrl Pts',(-5.58085013884738,36.3579352482258,8.90756157266984));
#9942=CARTESIAN_POINT('Ctrl Pts',(-5.97269230029302,36.3795336797535,8.6497097037301));
#9943=CARTESIAN_POINT('Ctrl Pts',(-6.61826543378769,36.4168520082205,8.16004546041644));
#9944=CARTESIAN_POINT('Ctrl Pts',(-6.8802984990199,36.4325393661667,7.94035799165896));
#9945=CARTESIAN_POINT('Ctrl Pts',(-7.33695081661843,36.4607156866972,7.51789532230048));
#9946=CARTESIAN_POINT('Ctrl Pts',(-7.53503811670473,36.4732972265957,7.31934431775822));
#9947=CARTESIAN_POINT('Ctrl Pts',(-8.16646712116347,36.5151189574526,6.63360230140625));
#9948=CARTESIAN_POINT('Ctrl Pts',(-8.56237840794939,36.5443408813799,6.11404270893559));
#9949=CARTESIAN_POINT('Ctrl Pts',(-9.15431016417877,36.5953852458462,5.16591720935694));
#9950=CARTESIAN_POINT('Ctrl Pts',(-9.37447975952864,36.6168585856071,4.75470442785361));
#9951=CARTESIAN_POINT('Ctrl Pts',(-9.71260358222404,36.6546272696711,4.00770226716491));
#9952=CARTESIAN_POINT('Ctrl Pts',(-9.84219671917791,36.6708823428343,3.67797826849634));
#9953=CARTESIAN_POINT('Ctrl Pts',(-10.158797385242,36.7159212325916,2.73500596547848));
#9954=CARTESIAN_POINT('Ctrl Pts',(-10.3067023173824,36.744370277336,2.11029105045309));
#9955=CARTESIAN_POINT('Ctrl Pts',(-10.4725128634216,36.7976415472326,0.942339456098136));
#9956=CARTESIAN_POINT('Ctrl Pts',(-10.5070723079455,36.8222295342717,0.403654384983058));
#9957=CARTESIAN_POINT('Ctrl Pts',(-10.4925952456766,36.8739423694035,-0.719977388160804));
#9958=CARTESIAN_POINT('Ctrl Pts',(-10.4362377743516,36.9009827940751,-1.30303665011896));
#9959=CARTESIAN_POINT('Ctrl Pts',(-10.2768407726382,36.9412896196935,-2.1797661302418));
#9960=CARTESIAN_POINT('Ctrl Pts',(-10.2088843604856,36.9550178146084,-2.47861258304013));
#9961=CARTESIAN_POINT('Ctrl Pts',(-10.0448419571441,36.9828740075259,-3.07752305632839));
#9962=CARTESIAN_POINT('Ctrl Pts',(-9.94816557881936,36.9969829310156,-3.37695367868638));
#9963=CARTESIAN_POINT('Ctrl Pts',(-9.83826083089393,37.0111767992967,-3.67146085683862));
#9964=CARTESIAN_POINT('Origin',(0.,20.,0.));
#9965=CARTESIAN_POINT('',(-9.92805791774766,39.9999999999999,-3.42120840958979));
#9966=CARTESIAN_POINT('Ctrl Pts',(-9.83826083089393,37.0111767992967,-3.67146085683862));
#9967=CARTESIAN_POINT('Ctrl Pts',(-9.73905989430054,37.0239883024752,-3.93728547731821));
#9968=CARTESIAN_POINT('Ctrl Pts',(-9.62908183107698,37.0368682888152,-4.19909901233635));
#9969=CARTESIAN_POINT('Ctrl Pts',(-9.31204345078195,37.0709788240597,-4.8755833547218));
#9970=CARTESIAN_POINT('Ctrl Pts',(-9.08799623536165,37.0923167188737,-5.28145627578774));
#9971=CARTESIAN_POINT('Ctrl Pts',(-8.64281680448154,37.1302894779228,-5.97521515508012));
#9972=CARTESIAN_POINT('Ctrl Pts',(-8.43217506162394,37.146880163272,-6.26896461977247));
#9973=CARTESIAN_POINT('Ctrl Pts',(-8.02950610498512,37.1761071144259,-6.773389170174));
#9974=CARTESIAN_POINT('Ctrl Pts',(-7.84325783494508,37.1888583955273,-6.98821000109359));
#9975=CARTESIAN_POINT('Ctrl Pts',(-7.19985813159442,37.2309848555009,-7.67214501608539));
#9976=CARTESIAN_POINT('Ctrl Pts',(-6.70757534334714,37.2603519889738,-8.10605795831986));
#9977=CARTESIAN_POINT('Ctrl Pts',(-5.79684588091793,37.3118068234315,-8.76868790868151));
#9978=CARTESIAN_POINT('Ctrl Pts',(-5.3973391202167,37.3335457799443,-9.02009036176285));
#9979=CARTESIAN_POINT('Ctrl Pts',(-4.6603466040634,37.3721009978974,-9.41732115860841));
#9980=CARTESIAN_POINT('Ctrl Pts',(-4.32953661791407,37.3888667626374,-9.57391756462574));
#9981=CARTESIAN_POINT('Ctrl Pts',(-3.69418348777181,37.4199177555993,-9.83499562536363));
#9982=CARTESIAN_POINT('Ctrl Pts',(-3.391700343897,37.4343002646923,-9.94336477591121));
#9983=CARTESIAN_POINT('Ctrl Pts',(-2.55140399884652,37.4737382637981,-10.2015995051287));
#9984=CARTESIAN_POINT('Ctrl Pts',(-2.00587894423726,37.4988211085439,-10.322728629309));
#9985=CARTESIAN_POINT('Ctrl Pts',(-1.00127896734655,37.5451076147441,-10.4631151954579));
#9986=CARTESIAN_POINT('Ctrl Pts',(-0.545597948904389,37.5661253639356,-10.4967448073524));
#9987=CARTESIAN_POINT('Ctrl Pts',(0.291343322489434,37.6046892413099,-10.5038532182323));
#9988=CARTESIAN_POINT('Ctrl Pts',(0.671777392509451,37.6221832103093,-10.4863981134722));
#9989=CARTESIAN_POINT('Ctrl Pts',(1.68827749329314,37.6684519883671,-10.3842032878484));
#9990=CARTESIAN_POINT('Ctrl Pts',(2.31891574870903,37.6969177537914,-10.261803365034));
#9991=CARTESIAN_POINT('Ctrl Pts',(3.44880206949852,37.7500520728763,-9.93296182153168));
#9992=CARTESIAN_POINT('Ctrl Pts',(3.95093229497363,37.7744828223189,-9.74413037141234));
#9993=CARTESIAN_POINT('Ctrl Pts',(4.98035424853465,37.8267427820846,-9.26429604315755));
#9994=CARTESIAN_POINT('Ctrl Pts',(5.50154477174102,37.8544943192975,-8.96460592972659));
#9995=CARTESIAN_POINT('Ctrl Pts',(6.25555846737383,37.8960118213246,-8.44039357706595));
#9996=CARTESIAN_POINT('Ctrl Pts',(6.50843760648304,37.9102647424265,-8.24696908397847));
#9997=CARTESIAN_POINT('Ctrl Pts',(7.18833163006239,37.9500905056219,-7.6761487026352));
#9998=CARTESIAN_POINT('Ctrl Pts',(7.59399490846076,37.9756913960834,-7.27506651489101));
#9999=CARTESIAN_POINT('Ctrl Pts',(8.26437312698382,38.0226453103723,-6.49476775697042));
#10000=CARTESIAN_POINT('Ctrl Pts',(8.54044653188181,38.0437961782442,-6.12720442133533));
#10001=CARTESIAN_POINT('Ctrl Pts',(8.99504740759032,38.0820942285981,-5.43125770824885));
#10002=CARTESIAN_POINT('Ctrl Pts',(9.18183133665637,38.0991923168503,-5.10915135950574));
#10003=CARTESIAN_POINT('Ctrl Pts',(9.47966242311408,38.1288368754527,-4.52623557170313));
#10004=CARTESIAN_POINT('Ctrl Pts',(9.59799392918533,38.1415133374784,-4.26958124020874));
#10005=CARTESIAN_POINT('Ctrl Pts',(9.95489857914898,38.1834602424146,-3.40539605679225));
#10006=CARTESIAN_POINT('Ctrl Pts',(10.1472103829282,38.2127179562829,-2.78043637764054));
#10007=CARTESIAN_POINT('Ctrl Pts',(10.3758195659338,38.2639163761495,-1.68309454794301));
#10008=CARTESIAN_POINT('Ctrl Pts',(10.440564379196,38.2855095746426,-1.21862389289477));
#10009=CARTESIAN_POINT('Ctrl Pts',(10.4985530174163,38.3228346917503,-0.410288687911039));
#10010=CARTESIAN_POINT('Ctrl Pts',(10.5063464927678,38.3385339041418,-0.0681825709019842));
#10011=CARTESIAN_POINT('Ctrl Pts',(10.4901281404209,38.3667168772567,0.553848274071962));
#10012=CARTESIAN_POINT('Ctrl Pts',(10.4716122148784,38.3792935880818,0.833592965782277));
#10013=CARTESIAN_POINT('Ctrl Pts',(10.3728913525475,38.4211091065636,1.76038397983086));
#10014=CARTESIAN_POINT('Ctrl Pts',(10.2436638455507,38.4503293711814,2.40065726962739));
#10015=CARTESIAN_POINT('Ctrl Pts',(9.92175328152203,38.5013651471385,3.47084560352994));
#10016=CARTESIAN_POINT('Ctrl Pts',(9.7580567830438,38.522831439781,3.90746400638749));
#10017=CARTESIAN_POINT('Ctrl Pts',(9.41973061163887,38.5606096343644,4.65459655315724));
#10018=CARTESIAN_POINT('Ctrl Pts',(9.25728787107139,38.576881052438,4.96983196561479));
#10019=CARTESIAN_POINT('Ctrl Pts',(8.75756552048223,38.6219139102628,5.8297379395082));
#10020=CARTESIAN_POINT('Ctrl Pts',(8.38597842898762,38.6503417503912,6.35265165756233));
#10021=CARTESIAN_POINT('Ctrl Pts',(7.61834100524716,38.7035717469729,7.24720422801135));
#10022=CARTESIAN_POINT('Ctrl Pts',(7.23667634886596,38.7281402557982,7.62834059879137));
#10023=CARTESIAN_POINT('Ctrl Pts',(6.38221701622929,38.7798927307959,8.35952978542744));
#10024=CARTESIAN_POINT('Ctrl Pts',(5.90583190373884,38.8069933455544,8.70262161585597));
#10025=CARTESIAN_POINT('Ctrl Pts',(5.14023112974277,38.8473792103231,9.16204970181207));
#10026=CARTESIAN_POINT('Ctrl Pts',(4.87036283062654,38.8611285463629,9.30831350363304));
#10027=CARTESIAN_POINT('Ctrl Pts',(4.05603717759795,38.9017532074208,9.70454111941243));
#10028=CARTESIAN_POINT('Ctrl Pts',(3.49618632051631,38.9286507952904,9.91999073676913));
#10029=CARTESIAN_POINT('Ctrl Pts',(2.47579919000137,38.9771556318177,10.2154924447661));
#10030=CARTESIAN_POINT('Ctrl Pts',(2.02251223623083,38.9985143726746,10.3148098128499));
#10031=CARTESIAN_POINT('Ctrl Pts',(1.20823159854175,39.0364477633893,10.4374678467502));
#10032=CARTESIAN_POINT('Ctrl Pts',(0.849774263710614,39.05297889355,10.4727483234094));
#10033=CARTESIAN_POINT('Ctrl Pts',(-0.150557562894974,39.0983254819715,
10.5194964790874));
#10034=CARTESIAN_POINT('Ctrl Pts',(-0.792721234902023,39.1268098596827,
10.4906666181723));
#10035=CARTESIAN_POINT('Ctrl Pts',(-1.96185848709003,39.1801001668114,10.33016123741));
#10036=CARTESIAN_POINT('Ctrl Pts',(-2.48904105681407,39.2046700212431,10.2159566660736));
#10037=CARTESIAN_POINT('Ctrl Pts',(-3.56660513830276,39.2564220553846,9.89412535282592));
#10038=CARTESIAN_POINT('Ctrl Pts',(-4.11308549598285,39.2835206738592,9.67971888053443));
#10039=CARTESIAN_POINT('Ctrl Pts',(-4.91444035227622,39.3239230545017,9.28513076552596));
#10040=CARTESIAN_POINT('Ctrl Pts',(-5.18396213346218,39.3376903890689,9.13739117525792));
#10041=CARTESIAN_POINT('Ctrl Pts',(-5.9588643346019,39.3783492217483,8.66728915003368));
#10042=CARTESIAN_POINT('Ctrl Pts',(-6.44356352423443,39.4052637002322,8.31326851901633));
#10043=CARTESIAN_POINT('Ctrl Pts',(-7.24559578786201,39.4538217092952,7.61497987927717));
#10044=CARTESIAN_POINT('Ctrl Pts',(-7.57516283688475,39.4752169540367,7.28721308807987));
#10045=CARTESIAN_POINT('Ctrl Pts',(-8.11832879363577,39.5130830508623,6.67021071066468));
#10046=CARTESIAN_POINT('Ctrl Pts',(-8.34083831023809,39.529511718192,6.38978908018728));
#10047=CARTESIAN_POINT('Ctrl Pts',(-8.92008950432261,39.5746764430164,5.57782727539355));
#10048=CARTESIAN_POINT('Ctrl Pts',(-9.24322060555003,39.6030796878232,5.02424581969796));
#10049=CARTESIAN_POINT('Ctrl Pts',(-9.74010614398457,39.6560841395034,3.96065361798012));
#10050=CARTESIAN_POINT('Ctrl Pts',(-9.92896772308112,39.6804485897593,3.46006088302585));
#10051=CARTESIAN_POINT('Ctrl Pts',(-10.2479972573181,39.7327488282212,2.36906749788065));
#10052=CARTESIAN_POINT('Ctrl Pts',(-10.3670148749052,39.7606089961443,1.77735091653152));
#10053=CARTESIAN_POINT('Ctrl Pts',(-10.4707089883898,39.8023742578623,0.859370525804358));
#10054=CARTESIAN_POINT('Ctrl Pts',(-10.4921025603994,39.8167677730611,0.538564742257382));
#10055=CARTESIAN_POINT('Ctrl Pts',(-10.5031253573529,39.8406699778085,0.00595797520689834));
#10056=CARTESIAN_POINT('Ctrl Pts',(-10.5011174646234,39.8501577388957,-0.205448543471378));
#10057=CARTESIAN_POINT('Ctrl Pts',(-10.474427538646,39.8804582490252,-0.877597004694431));
#10058=CARTESIAN_POINT('Ctrl Pts',(-10.4257701944779,39.9013847797024,-1.3368282622233));
#10059=CARTESIAN_POINT('Ctrl Pts',(-10.2512300573561,39.948272470248,-2.34498902998284));
#10060=CARTESIAN_POINT('Ctrl Pts',(-10.111105597097,39.9742790179436,-2.89001950066633));
#10061=CARTESIAN_POINT('Ctrl Pts',(-9.92805791774766,39.9999999999999,-3.42120840958979));
#10062=CARTESIAN_POINT('',(-1.99079507083261,40.,10.3105642903746));
#10063=CARTESIAN_POINT('Origin',(0.,40.,0.));
#10064=CARTESIAN_POINT('Ctrl Pts',(-9.83826089695936,37.8294631792708,-3.67146067980586));
#10065=CARTESIAN_POINT('Ctrl Pts',(-9.77094254382746,37.8382187820919,-3.85185087842846));
#10066=CARTESIAN_POINT('Ctrl Pts',(-9.69866848483662,37.846974384913,-4.03037036327237));
#10067=CARTESIAN_POINT('Ctrl Pts',(-9.62155384401236,37.8557299877341,-4.20674489680216));
#10068=CARTESIAN_POINT('Ctrl Pts',(-9.51967913321628,37.8672968509875,-4.43974999678165));
#10069=CARTESIAN_POINT('Ctrl Pts',(-9.40932061872495,37.8788637142408,-4.66908884410418));
#10070=CARTESIAN_POINT('Ctrl Pts',(-9.29076776060943,37.8904305774941,-4.89414297077848));
#10071=CARTESIAN_POINT('Ctrl Pts',(-9.17223566898852,37.90199541462,-5.1191576754989));
#10072=CARTESIAN_POINT('Ctrl Pts',(-9.04551222811113,37.9135602517459,-5.33988891303509));
#10073=CARTESIAN_POINT('Ctrl Pts',(-8.91093325131949,37.9251250888717,-5.55574203779555));
#10074=CARTESIAN_POINT('Ctrl Pts',(-8.77636931441923,37.9366886335677,-5.77157103986145));
#10075=CARTESIAN_POINT('Ctrl Pts',(-8.63395174090342,37.9482521782636,-5.98252278281403));
#10076=CARTESIAN_POINT('Ctrl Pts',(-8.48406072464668,37.9598157229596,-6.18802994663953));
#10077=CARTESIAN_POINT('Ctrl Pts',(-8.33415787571415,37.9713801805033,-6.39355333358303));
#10078=CARTESIAN_POINT('Ctrl Pts',(-8.17678056561697,37.982944638047,-6.5936310568969));
#10079=CARTESIAN_POINT('Ctrl Pts',(-8.01235129321971,37.9945090955907,-6.78772625803666));
#10080=CARTESIAN_POINT('Ctrl Pts',(-7.84792499971485,38.0060733436262,-6.98181794283954));
#10081=CARTESIAN_POINT('Ctrl Pts',(-7.67644717980999,38.0176375916618,-7.16992711216884));
#10082=CARTESIAN_POINT('Ctrl Pts',(-7.49837995428014,38.0292018396973,-7.35155079294497));
#10083=CARTESIAN_POINT('Ctrl Pts',(-7.32027095783454,38.040768800468,-7.53321707890824));
#10084=CARTESIAN_POINT('Ctrl Pts',(-7.13556965973243,38.0523357612388,-7.70839463730592));
#10085=CARTESIAN_POINT('Ctrl Pts',(-6.94477534909153,38.0639027220095,-7.87661706258788));
#10086=CARTESIAN_POINT('Ctrl Pts',(-6.77939063709363,38.0739292184461,-8.02243596705831));
#10087=CARTESIAN_POINT('Ctrl Pts',(-6.60942841200211,38.0839557148826,-8.16302942840252));
#10088=CARTESIAN_POINT('Ctrl Pts',(-6.43523447667231,38.0939822113192,-8.2981177522525));
#10089=CARTESIAN_POINT('Ctrl Pts',(-6.23426730180032,38.1055497590579,-8.45396886584565));
#10090=CARTESIAN_POINT('Ctrl Pts',(-6.02760467181233,38.1171173067966,-8.60254000476339));
#10091=CARTESIAN_POINT('Ctrl Pts',(-5.81579678690838,38.1286848545354,-8.74342660136094));
#10092=CARTESIAN_POINT('Ctrl Pts',(-5.6040259696663,38.1402503778832,-8.88428854195134));
#10093=CARTESIAN_POINT('Ctrl Pts',(-5.38711192540109,38.151815901231,-9.01746847168526));
#10094=CARTESIAN_POINT('Ctrl Pts',(-5.16563415427181,38.1633814245789,-9.14260492333671));
#10095=CARTESIAN_POINT('Ctrl Pts',(-4.94418113678743,38.1749456552965,-9.26772738900991));
#10096=CARTESIAN_POINT('Ctrl Pts',(-4.71816565177371,38.1865098860141,-9.38480803549227));
#10097=CARTESIAN_POINT('Ctrl Pts',(-4.48819309123835,38.1980741167318,-9.49353062752527));
#10098=CARTESIAN_POINT('Ctrl Pts',(-4.25820248152583,38.209639255057,-9.60226175254725));
#10099=CARTESIAN_POINT('Ctrl Pts',(-4.0242544245351,38.2212043933823,-9.70263339102094));
#10100=CARTESIAN_POINT('Ctrl Pts',(-3.78697688107134,38.2327695317075,-9.79437629980752));
#10101=CARTESIAN_POINT('Ctrl Pts',(-3.54970371597984,38.2443344566267,-9.88611751570483));
#10102=CARTESIAN_POINT('Ctrl Pts',(-3.30910144613982,38.2558993815458,-9.969230222245));
#10103=CARTESIAN_POINT('Ctrl Pts',(-3.06581660782314,38.2674643064649,-10.0434938904345));
#10104=CARTESIAN_POINT('Ctrl Pts',(-2.82247493856302,38.2790319329318,-10.1177749064964));
#10105=CARTESIAN_POINT('Ctrl Pts',(-2.57644971301954,38.2905995593986,-10.1832026711533));
#10106=CARTESIAN_POINT('Ctrl Pts',(-2.32840260480898,38.3021671858654,-10.2396065505428));
#10107=CARTESIAN_POINT('Ctrl Pts',(-2.11348977034709,38.3121896022117,-10.2884759676535));
#10108=CARTESIAN_POINT('Ctrl Pts',(-1.8970594779061,38.322212018558,-10.3305720727984));
#10109=CARTESIAN_POINT('Ctrl Pts',(-1.67954864780435,38.3322344349043,-10.3658148420497));
#10110=CARTESIAN_POINT('Ctrl Pts',(-1.42852518973776,38.3438010387753,-10.406487583748));
#10111=CARTESIAN_POINT('Ctrl Pts',(-1.17598466307407,38.3553676426462,-10.4380439947674));
#10112=CARTESIAN_POINT('Ctrl Pts',(-0.922603674343791,38.3669342465172,
-10.4603921274533));
#10113=CARTESIAN_POINT('Ctrl Pts',(-0.669267061252899,38.3784988246819,
-10.4827363462202));
#10114=CARTESIAN_POINT('Ctrl Pts',(-0.415090555598662,38.3900634028467,
-10.4958754816972));
#10115=CARTESIAN_POINT('Ctrl Pts',(-0.160755867377762,38.4016279810114,
-10.4997694522834));
#10116=CARTESIAN_POINT('Ctrl Pts',(0.0935504220672181,38.4131912678861,
-10.5036629880725));
#10117=CARTESIAN_POINT('Ctrl Pts',(0.348014582076939,38.4247545547607,-10.4983134159245));
#10118=CARTESIAN_POINT('Ctrl Pts',(0.601953812652019,38.4363178416354,-10.4837327611607));
#10119=CARTESIAN_POINT('Ctrl Pts',(0.855913169215033,38.4478820449599,-10.4691509508051));
#10120=CARTESIAN_POINT('Ctrl Pts',(1.10934723657866,38.4594462482844,-10.4453366084573));
#10121=CARTESIAN_POINT('Ctrl Pts',(1.36157588496065,38.4710104516089,-10.4123538217587));
#10122=CARTESIAN_POINT('Ctrl Pts',(1.61380001522755,38.4825744477865,-10.3793716258734));
#10123=CARTESIAN_POINT('Ctrl Pts',(1.8648184953714,38.494138443964,-10.3372213518512));
#10124=CARTESIAN_POINT('Ctrl Pts',(2.11395819808633,38.5057024401416,-10.2860187505538));
#10125=CARTESIAN_POINT('Ctrl Pts',(2.36315646670326,38.517269154697,-10.2348041129309));
#10126=CARTESIAN_POINT('Ctrl Pts',(2.61047480368251,38.5288358692525,-10.1745329500001));
#10127=CARTESIAN_POINT('Ctrl Pts',(2.85525066777235,38.5404025838079,-10.105372067578));
#10128=CARTESIAN_POINT('Ctrl Pts',(3.06746464147513,38.5504306087018,-10.0454114757192));
#10129=CARTESIAN_POINT('Ctrl Pts',(3.2777676572117,38.5604586335956,-9.97876982858072));
#10130=CARTESIAN_POINT('Ctrl Pts',(3.48573704249832,38.5704866584894,-9.90558621539155));
#10131=CARTESIAN_POINT('Ctrl Pts',(3.7256265304417,38.5820538310016,-9.82117004293616));
#10132=CARTESIAN_POINT('Ctrl Pts',(3.96248524580083,38.5936210035138,-9.7280223607574));
#10133=CARTESIAN_POINT('Ctrl Pts',(4.19567502657272,38.605188176026,-9.62638624154433));
#10134=CARTESIAN_POINT('Ctrl Pts',(4.42882392223932,38.6167533204687,-9.52476794216635));
#10135=CARTESIAN_POINT('Ctrl Pts',(4.65830491383272,38.6283184649115,-9.41466428731077));
#10136=CARTESIAN_POINT('Ctrl Pts',(4.88350017832237,38.6398836093542,-9.29636633359107));
#10137=CARTESIAN_POINT('Ctrl Pts',(5.10867022262449,38.6514474585872,-9.17808162835856));
#10138=CARTESIAN_POINT('Ctrl Pts',(5.32955525319949,38.6630113078201,-9.0516045853062));
#10139=CARTESIAN_POINT('Ctrl Pts',(5.54556142486565,38.6745751570531,-8.91727253609768));
#10140=CARTESIAN_POINT('Ctrl Pts',(5.76158452743253,38.6861399126786,-8.78292995773359));
#10141=CARTESIAN_POINT('Ctrl Pts',(5.97272777009596,38.6977046683041,-8.64073128630361));
#10142=CARTESIAN_POINT('Ctrl Pts',(6.17842456612679,38.7092694239296,-8.4910582897941));
#10143=CARTESIAN_POINT('Ctrl Pts',(6.38411756461389,38.7208339660483,-8.34138805652523));
#10144=CARTESIAN_POINT('Ctrl Pts',(6.58436409479135,38.732398508167,-8.18424393853169));
#10145=CARTESIAN_POINT('Ctrl Pts',(6.77862844023465,38.7439630502857,-8.02004971737968));
#10146=CARTESIAN_POINT('Ctrl Pts',(6.9729382103727,38.7555302965331,-7.85581710280887));
#10147=CARTESIAN_POINT('Ctrl Pts',(7.16126278800572,38.7670975427805,-7.68453126845112));
#10148=CARTESIAN_POINT('Ctrl Pts',(7.34310018304362,38.7786647890279,-7.50665576017609));
#10149=CARTESIAN_POINT('Ctrl Pts',(7.50068867675949,38.7886894867101,-7.35250081634749));
#10150=CARTESIAN_POINT('Ctrl Pts',(7.65340527614783,38.7987141843923,-7.19339723453153));
#10151=CARTESIAN_POINT('Ctrl Pts',(7.80094570771884,38.8087388820745,-7.02966905801567));
#10152=CARTESIAN_POINT('Ctrl Pts',(7.97121434138562,38.8203078571622,-6.8407190013345));
#10153=CARTESIAN_POINT('Ctrl Pts',(8.13464093951674,38.8318768322498,-6.64555079086006));
#10154=CARTESIAN_POINT('Ctrl Pts',(8.29078139631834,38.8434458073375,-6.44468345525688));
#10155=CARTESIAN_POINT('Ctrl Pts',(8.44689466556719,38.8550127680073,-6.2438510951584));
#10156=CARTESIAN_POINT('Ctrl Pts',(8.59572415644224,38.8665797286772,-6.0373218092466));
#10157=CARTESIAN_POINT('Ctrl Pts',(8.73686658849573,38.878146689347,-5.82564702113225));
#10158=CARTESIAN_POINT('Ctrl Pts',(8.87799331885964,38.8897123632257,-5.61399578122921));
#10159=CARTESIAN_POINT('Ctrl Pts',(9.01143454448961,38.9012780371045,-5.39720041215829));
#10160=CARTESIAN_POINT('Ctrl Pts',(9.13683018625149,38.9128437109832,-5.17584149173867));
#10161=CARTESIAN_POINT('Ctrl Pts',(9.26223565280135,38.9244102910361,-4.954465227778));
#10162=CARTESIAN_POINT('Ctrl Pts',(9.37959413660401,38.935976871089,-4.72852493708156));
#10163=CARTESIAN_POINT('Ctrl Pts',(9.48859075957795,38.947543451142,-4.49862716806493));
#10164=CARTESIAN_POINT('Ctrl Pts',(9.59758534383811,38.9591098148492,-4.26873369914254));
#10165=CARTESIAN_POINT('Ctrl Pts',(9.69821826319937,38.9706761785565,-4.03488315072581));
#10166=CARTESIAN_POINT('Ctrl Pts',(9.79022185148132,38.9822425422637,-3.79770418789796));
#10167=CARTESIAN_POINT('Ctrl Pts',(9.88224680885461,38.9938115924171,-3.56047013701305));
#10168=CARTESIAN_POINT('Ctrl Pts',(9.96563832845879,39.0053806425705,-3.31990638438948));
#10169=CARTESIAN_POINT('Ctrl Pts',(10.0401773872344,39.0169496927239,-3.07666037008744));
#10170=CARTESIAN_POINT('Ctrl Pts',(10.1046960415992,39.0269634970358,-2.86611430497557));
#10171=CARTESIAN_POINT('Ctrl Pts',(10.1625830940346,39.0369773013477,-2.6535590560069));
#10172=CARTESIAN_POINT('Ctrl Pts',(10.2137267948667,39.0469911056596,-2.43942328426641));
#10173=CARTESIAN_POINT('Ctrl Pts',(10.2727689972203,39.0585514161357,-2.19221693508691));
#10174=CARTESIAN_POINT('Ctrl Pts',(10.3228415404747,39.0701117266117,-1.94282670607944));
#10175=CARTESIAN_POINT('Ctrl Pts',(10.3638027893578,39.0816720370877,-1.69191983950168));
#10176=CARTESIAN_POINT('Ctrl Pts',(10.404756765153,39.0932302949127,-1.44105752399942));
#10177=CARTESIAN_POINT('Ctrl Pts',(10.4366026314068,39.1047885527376,-1.18867938222004));
#10178=CARTESIAN_POINT('Ctrl Pts',(10.4592500983269,39.1163468105625,-0.935461586944217));
#10179=CARTESIAN_POINT('Ctrl Pts',(10.4818950172023,39.1279037679789,-0.682272280959553));
#10180=CARTESIAN_POINT('Ctrl Pts',(10.495343578375,39.1394607253953,-0.428243786373147));
#10181=CARTESIAN_POINT('Ctrl Pts',(10.4995573756991,39.1510176828117,-0.174057215886499));
#10182=CARTESIAN_POINT('Ctrl Pts',(10.5037715185744,39.1625755879527,0.0801501990879922));
#10183=CARTESIAN_POINT('Ctrl Pts',(10.498749376384,39.1741334930937,0.334515438451618));
#10184=CARTESIAN_POINT('Ctrl Pts',(10.4845046605004,39.1856913982347,0.588356204985865));
#10185=CARTESIAN_POINT('Ctrl Pts',(10.4702601673197,39.1972491226785,0.842193002955999));
#10186=CARTESIAN_POINT('Ctrl Pts',(10.4467934063272,39.2088068471224,1.0955050675247));
#10187=CARTESIAN_POINT('Ctrl Pts',(10.4141701280644,39.2203645715663,1.347613276772));
#10188=CARTESIAN_POINT('Ctrl Pts',(10.381538928838,39.2319251022369,1.59978269813591));
#10189=CARTESIAN_POINT('Ctrl Pts',(10.3397468037936,39.2434856329074,1.85074740453948));
#10190=CARTESIAN_POINT('Ctrl Pts',(10.2889112005542,39.255046163578,2.09983506664455));
#10191=CARTESIAN_POINT('Ctrl Pts',(10.2446487822583,39.2651118854669,2.31671500097967));
#10192=CARTESIAN_POINT('Ctrl Pts',(10.1935311964916,39.2751776073558,2.53217192609222));
#10193=CARTESIAN_POINT('Ctrl Pts',(10.1356674049065,39.2852433292447,2.74576897373338));
#10194=CARTESIAN_POINT('Ctrl Pts',(10.0690759979193,39.296827267396,2.99158293685373));
#10195=CARTESIAN_POINT('Ctrl Pts',(9.99352834835741,39.3084112055473,3.2350090451317));
#10196=CARTESIAN_POINT('Ctrl Pts',(9.90922078800109,39.3199951436986,3.47539125490169));
#10197=CARTESIAN_POINT('Ctrl Pts',(9.82492758520526,39.3315771091076,3.71573252762991));
#10198=CARTESIAN_POINT('Ctrl Pts',(9.73187754086394,39.3431590745166,3.95303067716415));
#10199=CARTESIAN_POINT('Ctrl Pts',(9.63031632810827,39.3547410399256,4.18664644083677));
#10200=CARTESIAN_POINT('Ctrl Pts',(9.52876641285088,39.3663217169763,4.42023621748527));
#10201=CARTESIAN_POINT('Ctrl Pts',(9.41870732932391,39.3779023940269,4.65014417391184));
#10202=CARTESIAN_POINT('Ctrl Pts',(9.30043265936412,39.3894830710776,4.87575156756713));
#10203=CARTESIAN_POINT('Ctrl Pts',(9.18214987722267,39.4010645424197,5.10137443510336));
#10204=CARTESIAN_POINT('Ctrl Pts',(9.05565050760297,39.4126460137618,5.32269590522329));
#10205=CARTESIAN_POINT('Ctrl Pts',(8.92127444893441,39.4242274851039,5.53912115834182));
#10206=CARTESIAN_POINT('Ctrl Pts',(8.7869018820538,39.4358086554992,5.75554078760817));
#10207=CARTESIAN_POINT('Ctrl Pts',(8.64465318193162,39.4473898258945,5.96706422131363));
#10208=CARTESIAN_POINT('Ctrl Pts',(8.49491242743469,39.4589709962898,6.17312431838334));
#10209=CARTESIAN_POINT('Ctrl Pts',(8.34514009761801,39.4705546087668,6.37922786663955));
#10210=CARTESIAN_POINT('Ctrl Pts',(8.18787271707229,39.4821382212438,6.57986555252028));
#10211=CARTESIAN_POINT('Ctrl Pts',(8.02353650941438,39.4937218337208,6.77450093232664));
#10212=CARTESIAN_POINT('Ctrl Pts',(7.88273702232438,39.5036464067572,6.94126005398868));
#10213=CARTESIAN_POINT('Ctrl Pts',(7.73674929148776,39.5135709797935,7.10361351542315));
#10214=CARTESIAN_POINT('Ctrl Pts',(7.58586439719135,39.5234955528298,7.26124385676619));
#10215=CARTESIAN_POINT('Ctrl Pts',(7.41051234539617,39.5350294724659,7.44443518223697));
#10216=CARTESIAN_POINT('Ctrl Pts',(7.22849149706608,39.5465633921019,7.62130277938994));
#10217=CARTESIAN_POINT('Ctrl Pts',(7.04028338094605,39.558097311738,7.79136771792828));
#10218=CARTESIAN_POINT('Ctrl Pts',(6.85210898568282,39.5696291648657,7.96140218628521));
#10219=CARTESIAN_POINT('Ctrl Pts',(6.65774974306552,39.5811610179933,8.12463624128184));
#10220=CARTESIAN_POINT('Ctrl Pts',(6.45772254452777,39.592692871121,8.28062923562563));
#10221=CARTESIAN_POINT('Ctrl Pts',(6.2577168989946,39.6042234816872,8.43660542166661));
#10222=CARTESIAN_POINT('Ctrl Pts',(6.05204473760968,39.6157540922535,8.58534193270929));
#10223=CARTESIAN_POINT('Ctrl Pts',(5.84125523482977,39.6272847028197,8.72643903786498));
#10224=CARTESIAN_POINT('Ctrl Pts',(5.63044338606736,39.6388165357562,8.86755110085016));
#10225=CARTESIAN_POINT('Ctrl Pts',(5.41451334264833,39.6503483686927,9.00102198096848));
#10226=CARTESIAN_POINT('Ctrl Pts',(5.19404353388615,39.6618802016292,9.12649509768649));
#10227=CARTESIAN_POINT('Ctrl Pts',(4.97357359805668,39.6734120412121,9.25196828672065));
#10228=CARTESIAN_POINT('Ctrl Pts',(4.74856413637869,39.6849438807949,9.36944356696252));
#10229=CARTESIAN_POINT('Ctrl Pts',(4.51961908132821,39.6964757203778,9.47860983265447));
#10230=CARTESIAN_POINT('Ctrl Pts',(4.2906085924439,39.7080108558277,9.58780729870271));
#10231=CARTESIAN_POINT('Ctrl Pts',(4.05766051472073,39.7195459912777,9.68869088273747));
#10232=CARTESIAN_POINT('Ctrl Pts',(3.82140107039531,39.7310811267276,9.7809966189127));
#10233=CARTESIAN_POINT('Ctrl Pts',(3.61203246650753,39.74130334329,9.86279619805342));
#10234=CARTESIAN_POINT('Ctrl Pts',(3.40006381849039,39.7515255598525,9.93786007685317));
#10235=CARTESIAN_POINT('Ctrl Pts',(3.18594275547069,39.7617477764149,10.0060366658764));
#10236=CARTESIAN_POINT('Ctrl Pts',(2.94219156771723,39.7733845457893,10.0836475478562));
#10237=CARTESIAN_POINT('Ctrl Pts',(2.69557041193126,39.7850213151637,10.1523578833729));
#10238=CARTESIAN_POINT('Ctrl Pts',(2.44674288382941,39.7966580845381,10.2119758254919));
#10239=CARTESIAN_POINT('Ctrl Pts',(2.19796065802866,39.8082927352867,10.2715829133858));
#10240=CARTESIAN_POINT('Ctrl Pts',(1.94697312436059,39.8199273860353,10.3221008501457));
#10241=CARTESIAN_POINT('Ctrl Pts',(1.69445649222457,39.8315620367839,10.3633883549715));
#10242=CARTESIAN_POINT('Ctrl Pts',(1.44197452343055,39.8431950904262,10.4046701921987));
#10243=CARTESIAN_POINT('Ctrl Pts',(1.18796414163377,39.8548281440686,10.4367240840553));
#10244=CARTESIAN_POINT('Ctrl Pts',(0.933110299572317,39.866461197711,10.4594601279814));
#10245=CARTESIAN_POINT('Ctrl Pts',(0.678258384732152,39.8780941633835,10.482195999976));
#10246=CARTESIAN_POINT('Ctrl Pts',(0.422563290990595,39.8897271290559,10.4956141379029));
#10247=CARTESIAN_POINT('Ctrl Pts',(0.166714969412438,39.9013600947284,10.4996765244923));
#10248=CARTESIAN_POINT('Ctrl Pts',(-0.0891139888816756,39.912992179987,
10.5037386036294));
#10249=CARTESIAN_POINT('Ctrl Pts',(-0.345095881899718,39.9246242652456,
10.4984463426919));
#10250=CARTESIAN_POINT('Ctrl Pts',(-0.600539942610578,39.9362563505041,
10.4838138469418));
#10251=CARTESIAN_POINT('Ctrl Pts',(-0.856008621241452,39.9478895567821,
10.4691799410137));
#10252=CARTESIAN_POINT('Ctrl Pts',(-1.11093909430189,39.9595227630601,10.4452040152679));
#10253=CARTESIAN_POINT('Ctrl Pts',(-1.36464347042229,39.971155969338,10.411952228023));
#10254=CARTESIAN_POINT('Ctrl Pts',(-1.57432647122329,39.9807706462253,10.3844701063579));
#10255=CARTESIAN_POINT('Ctrl Pts',(-1.7831719369394,39.9903853231127,10.3506527957081));
#10256=CARTESIAN_POINT('Ctrl Pts',(-1.99079507083262,40.,10.3105642903746));
#10257=CARTESIAN_POINT('Origin',(0.,13.3748739960349,0.));
#10258=CARTESIAN_POINT('',(-12.1744999965607,38.6251260039651,0.00028938649696687));
#10259=CARTESIAN_POINT('Ctrl Pts',(1.59078448392769,37.8125509746976,12.0701224093087));
#10260=CARTESIAN_POINT('Ctrl Pts',(1.30897780039443,37.8236982341459,12.1072631842262));
#10261=CARTESIAN_POINT('Ctrl Pts',(1.02589220353336,37.8348454935942,12.134527500853));
#10262=CARTESIAN_POINT('Ctrl Pts',(0.74223387350245,37.8459927530425,12.1518533206678));
#10263=CARTESIAN_POINT('Ctrl Pts',(0.547788829828789,37.8536340916558,12.1637300026965));
#10264=CARTESIAN_POINT('Ctrl Pts',(0.353074788441565,37.8612754302692,12.170937692811));
#10265=CARTESIAN_POINT('Ctrl Pts',(0.158319908679642,37.8689167688825,12.173470542804));
#10266=CARTESIAN_POINT('Ctrl Pts',(-0.12579174714368,37.8800640806664,12.1771655064749));
#10267=CARTESIAN_POINT('Ctrl Pts',(-0.410075244090132,37.8912113924504,
12.1709105297779));
#10268=CARTESIAN_POINT('Ctrl Pts',(-0.69382202769014,37.9023587042343,12.1547135401823));
#10269=CARTESIAN_POINT('Ctrl Pts',(-0.97752061690601,37.9135041226476,12.138519301645));
#10270=CARTESIAN_POINT('Ctrl Pts',(-1.26068240856565,37.9246495410609,12.1123864367957));
#10271=CARTESIAN_POINT('Ctrl Pts',(-1.54260128195161,37.9357949594742,12.0763749335188));
#10272=CARTESIAN_POINT('Ctrl Pts',(-1.82448885756292,37.9469391405571,12.0403674281293));
#10273=CARTESIAN_POINT('Ctrl Pts',(-2.10513352590578,37.95808332164,11.9944835080307));
#10274=CARTESIAN_POINT('Ctrl Pts',(-2.3838354609949,37.9692275027229,11.9388348989716));
#10275=CARTESIAN_POINT('Ctrl Pts',(-2.67131404013712,37.9807226268683,11.8814338512953));
#10276=CARTESIAN_POINT('Ctrl Pts',(-2.95672525267232,37.9922177510137,11.8136431952157));
#10277=CARTESIAN_POINT('Ctrl Pts',(-3.23931225686388,38.0037128751591,11.735642562405));
#10278=CARTESIAN_POINT('Ctrl Pts',(-3.51328659390697,38.0148576517066,11.6600192274806));
#10279=CARTESIAN_POINT('Ctrl Pts',(-3.78460605649641,38.0260024282542,11.5747991324066));
#10280=CARTESIAN_POINT('Ctrl Pts',(-4.05259512972827,38.0371472048018,11.4801969915373));
#10281=CARTESIAN_POINT('Ctrl Pts',(-4.33322097422901,38.0488175027461,11.3811339761955));
#10282=CARTESIAN_POINT('Ctrl Pts',(-4.61019448973532,38.0604878006904,11.2717829285034));
#10283=CARTESIAN_POINT('Ctrl Pts',(-4.88276104735215,38.0721580986347,11.152447928794));
#10284=CARTESIAN_POINT('Ctrl Pts',(-5.15532760496899,38.0838283965791,11.0331129290845));
#10285=CARTESIAN_POINT('Ctrl Pts',(-5.42348690088374,38.0954986945234,10.9037941199549));
#10286=CARTESIAN_POINT('Ctrl Pts',(-5.68651039168178,38.1071689924677,10.7648525217624));
#10287=CARTESIAN_POINT('Ctrl Pts',(-5.93774685158698,38.1183163022865,10.6321373975067));
#10288=CARTESIAN_POINT('Ctrl Pts',(-6.18437272836615,38.1294636121054,10.4906033555107));
#10289=CARTESIAN_POINT('Ctrl Pts',(-6.42576965953203,38.1406109219243,10.340596430218));
#10290=CARTESIAN_POINT('Ctrl Pts',(-6.66712559058785,38.1517563384261,10.1906149828815));
#10291=CARTESIAN_POINT('Ctrl Pts',(-6.9032541226648,38.1629017549279,10.0321636661054));
#10292=CARTESIAN_POINT('Ctrl Pts',(-7.13356394341092,38.1740471714297,9.86563306206286));
#10293=CARTESIAN_POINT('Ctrl Pts',(-7.36384819705636,38.1851913506591,9.69912094487725));
#10294=CARTESIAN_POINT('Ctrl Pts',(-7.58831481311788,38.1963355298885,9.52453148764227));
#10295=CARTESIAN_POINT('Ctrl Pts',(-7.80640276521373,38.2074797091179,9.34229768939438));
#10296=CARTESIAN_POINT('Ctrl Pts',(-8.03135862286497,38.2189748346958,9.15432508483766));
#10297=CARTESIAN_POINT('Ctrl Pts',(-8.24952732595125,38.2304699602737,8.95821905765051));
#10298=CARTESIAN_POINT('Ctrl Pts',(-8.46033028003315,38.2419650858516,8.75449951754835));
#10299=CARTESIAN_POINT('Ctrl Pts',(-8.66470833983174,38.2531098607101,8.55698898203202));
#10300=CARTESIAN_POINT('Ctrl Pts',(-8.86216279097333,38.2642546355686,8.35232234771498));
#10301=CARTESIAN_POINT('Ctrl Pts',(-9.05220323824906,38.2753994104272,8.14101141034904));
#10302=CARTESIAN_POINT('Ctrl Pts',(-9.25120494426631,38.2870697113648,7.91973621531168));
#10303=CARTESIAN_POINT('Ctrl Pts',(-9.44207640298544,38.2987400123023,7.69117525897117));
#10304=CARTESIAN_POINT('Ctrl Pts',(-9.6243005169155,38.3104103132399,7.45595666632393));
#10305=CARTESIAN_POINT('Ctrl Pts',(-9.80652463084557,38.3220806141775,7.22073807367666));
#10306=CARTESIAN_POINT('Ctrl Pts',(-9.98010120145821,38.3337509151151,6.97886211532039));
#10307=CARTESIAN_POINT('Ctrl Pts',(-10.144563284333,38.3454212160527,6.73099443025792));
#10308=CARTESIAN_POINT('Ctrl Pts',(-10.3016546456759,38.3565684873844,6.49423546795641));
#10309=CARTESIAN_POINT('Ctrl Pts',(-10.4504774518845,38.367715758716,6.25193932153469));
#10310=CARTESIAN_POINT('Ctrl Pts',(-10.5906543344632,38.3788630300476,6.00470573949428));
#10311=CARTESIAN_POINT('Ctrl Pts',(-10.7308074057654,38.3900084078376,5.7575141540162));
#10312=CARTESIAN_POINT('Ctrl Pts',(-10.8623173540756,38.4011537856276,5.50538703934738));
#10313=CARTESIAN_POINT('Ctrl Pts',(-10.9848518805822,38.4122991634176,5.24895031522197));
#10314=CARTESIAN_POINT('Ctrl Pts',(-11.1073728029286,38.4234433038135,4.99254206149096));
#10315=CARTESIAN_POINT('Ctrl Pts',(-11.2209201783031,38.4345874442093,4.73182539434702));
#10316=CARTESIAN_POINT('Ctrl Pts',(-11.3252085991643,38.4457315846052,4.46744898520573));
#10317=CARTESIAN_POINT('Ctrl Pts',(-11.4327818597973,38.4572267391913,4.19474534149411));
#10318=CARTESIAN_POINT('Ctrl Pts',(-11.5305033242619,38.4687218937773,3.91814794521018));
#10319=CARTESIAN_POINT('Ctrl Pts',(-11.6181137451896,38.4802170483634,3.63839020087693));
#10320=CARTESIAN_POINT('Ctrl Pts',(-11.7030534493892,38.4913617845709,3.36716059371813));
#10321=CARTESIAN_POINT('Ctrl Pts',(-11.7784893469094,38.5025065207784,3.09296073127381));
#10322=CARTESIAN_POINT('Ctrl Pts',(-11.8442357567959,38.513651256986,2.81647467367221));
#10323=CARTESIAN_POINT('Ctrl Pts',(-11.9130830140131,38.5253216207613,2.52694849638708));
#10324=CARTESIAN_POINT('Ctrl Pts',(-11.9713047289161,38.5369919845366,2.23491559225353));
#10325=CARTESIAN_POINT('Ctrl Pts',(-12.0187474391742,38.5486623483119,1.94117496463956));
#10326=CARTESIAN_POINT('Ctrl Pts',(-12.0661901494323,38.5603327120872,1.64743433702562));
#10327=CARTESIAN_POINT('Ctrl Pts',(-12.1028538102164,38.5720030758626,1.35198631855737));
#10328=CARTESIAN_POINT('Ctrl Pts',(-12.1286469510863,38.5836734396379,1.05563885202526));
#10329=CARTESIAN_POINT('Ctrl Pts',(-12.1549901730804,38.5955926931028,0.752971288674556));
#10330=CARTESIAN_POINT('Ctrl Pts',(-12.1700001024465,38.6075119465678,0.449311157315627));
#10331=CARTESIAN_POINT('Ctrl Pts',(-12.173630879507,38.6194312000327,0.145469789009793));
#10332=CARTESIAN_POINT('Ctrl Pts',(-12.1742091193982,38.6213294680102,0.0970798171563845));
#10333=CARTESIAN_POINT('Ctrl Pts',(-12.1744988461963,38.6232277359876,0.0486852550215822));
#10334=CARTESIAN_POINT('Ctrl Pts',(-12.1744999965607,38.6251260039651,0.00028938649696687));
#10335=CARTESIAN_POINT('',(11.7598063682261,40.,-3.15424737243508));
#10336=CARTESIAN_POINT('Ctrl Pts',(-12.1748649577908,38.6251260151384,0.000289110302658423));
#10337=CARTESIAN_POINT('Ctrl Pts',(-12.1731836483798,38.6907258978333,-1.67221371080106));
#10338=CARTESIAN_POINT('Ctrl Pts',(-11.4051697641933,38.8357431883897,-5.37100026957135));
#10339=CARTESIAN_POINT('Ctrl Pts',(-7.77755196994913,39.060177886808,-10.0290176561892));
#10340=CARTESIAN_POINT('Ctrl Pts',(-2.02988957584845,39.2984301103931,-12.5280053565324));
#10341=CARTESIAN_POINT('Ctrl Pts',(4.21283654000685,39.5366823339782,-11.9717980432598));
#10342=CARTESIAN_POINT('Ctrl Pts',(9.3318903658005,39.7705389638472,-8.56008252992691));
#10343=CARTESIAN_POINT('Ctrl Pts',(11.263434788298,39.9249781858544,-5.00116413859683));
#10344=CARTESIAN_POINT('Ctrl Pts',(11.7598063682261,40.,-3.15424737243508));
#10345=CARTESIAN_POINT('',(8.61094305413662,40.,-8.60639936142963));
#10346=CARTESIAN_POINT('Origin',(0.,40.,0.));
#10347=CARTESIAN_POINT('',(-12.1744916248676,38.8748739948544,0.000309104184771874));
#10348=CARTESIAN_POINT('Ctrl Pts',(-12.1742135449704,38.8748739960349,0.000309067021438125));
#10349=CARTESIAN_POINT('Ctrl Pts',(-12.1728218038936,38.9322463659098,-1.46265402061263));
#10350=CARTESIAN_POINT('Ctrl Pts',(-11.5435367915227,39.0690361436464,-4.95189231269601));
#10351=CARTESIAN_POINT('Ctrl Pts',(-8.28522524716096,39.2852433292447,-9.61375508410346));
#10352=CARTESIAN_POINT('Ctrl Pts',(-2.67484068581488,39.5234955528298,-12.4063460053113));
#10353=CARTESIAN_POINT('Ctrl Pts',(3.58926667070469,39.7617477764149,-12.1735736829301));
#10354=CARTESIAN_POINT('Ctrl Pts',(7.17942834059384,39.9205825921383,-10.0386698338782));
#10355=CARTESIAN_POINT('Ctrl Pts',(8.61094305413662,40.,-8.60639936142963));
#10356=CARTESIAN_POINT('Ctrl Pts',(1.59078448392772,38.0622997972676,12.0701224093087));
#10357=CARTESIAN_POINT('Ctrl Pts',(1.32384075218273,38.0728606019514,12.1053043181693));
#10358=CARTESIAN_POINT('Ctrl Pts',(1.05575738715399,38.0834214066353,12.131623455312));
#10359=CARTESIAN_POINT('Ctrl Pts',(0.787134657080782,38.0939822113192,12.1490275035339));
#10360=CARTESIAN_POINT('Ctrl Pts',(0.503583140229768,38.1051299358117,12.1673987868252));
#10361=CARTESIAN_POINT('Ctrl Pts',(0.219345890921422,38.1162776603042,12.1758415742294));
#10362=CARTESIAN_POINT('Ctrl Pts',(-0.0648690228389137,38.1274253847967,
12.1743271789399));
#10363=CARTESIAN_POINT('Ctrl Pts',(-0.349035688152791,38.1385712168467,
12.1728130407349));
#10364=CARTESIAN_POINT('Ctrl Pts',(-0.633179758886583,38.1497170488967,
12.1613450960154));
#10365=CARTESIAN_POINT('Ctrl Pts',(-0.916592908336909,38.1608628809466,
12.1399467746109));
#10366=CARTESIAN_POINT('Ctrl Pts',(-1.19997459133722,38.1720074755108,12.1185508289933));
#10367=CARTESIAN_POINT('Ctrl Pts',(-1.48262524921969,38.1831520700749,12.0872267283601));
#10368=CARTESIAN_POINT('Ctrl Pts',(-1.76384016867791,38.194296664639,12.0460498965162));
#10369=CARTESIAN_POINT('Ctrl Pts',(-2.05389228566501,38.2057914788278,12.0035790799957));
#10370=CARTESIAN_POINT('Ctrl Pts',(-2.34241667380791,38.2172862930165,11.9506263064734));
#10371=CARTESIAN_POINT('Ctrl Pts',(-2.62864831310905,38.2287811072053,11.8873318409132));
#10372=CARTESIAN_POINT('Ctrl Pts',(-2.90617384669823,38.2399262917455,11.8259625584302));
#10373=CARTESIAN_POINT('Ctrl Pts',(-3.18154377189134,38.2510714762857,11.7548714598031));
#10374=CARTESIAN_POINT('Ctrl Pts',(-3.45407233157046,38.2622166608259,11.6742380727086));
#10375=CARTESIAN_POINT('Ctrl Pts',(-3.73942491370659,38.2738862898389,11.5898104250489));
#10376=CARTESIAN_POINT('Ctrl Pts',(-4.02166199993082,38.285555918852,11.4949209773659));
#10377=CARTESIAN_POINT('Ctrl Pts',(-4.30001441364412,38.2972255478651,11.3898343399916));
#10378=CARTESIAN_POINT('Ctrl Pts',(-4.57836682735739,38.3088951768782,11.2847477026174));
#10379=CARTESIAN_POINT('Ctrl Pts',(-4.85283425796642,38.3205648058912,11.1694640021579));
#10380=CARTESIAN_POINT('Ctrl Pts',(-5.12267062571763,38.3322344349043,11.0443060402367));
#10381=CARTESIAN_POINT('Ctrl Pts',(-5.38041794246529,38.343381248029,10.9247553320664));
#10382=CARTESIAN_POINT('Ctrl Pts',(-5.63401694334377,38.3545280611537,10.796160008172));
#10383=CARTESIAN_POINT('Ctrl Pts',(-5.88283226064311,38.3656748742783,10.6588336530381));
#10384=CARTESIAN_POINT('Ctrl Pts',(-6.1316053072015,38.376819793693,10.5215306280063));
#10385=CARTESIAN_POINT('Ctrl Pts',(-6.37559605922401,38.3879647131077,10.3754996620031));
#10386=CARTESIAN_POINT('Ctrl Pts',(-6.61419386041611,38.3991096325224,10.2211002258482));
#10387=CARTESIAN_POINT('Ctrl Pts',(-6.85276519254124,38.4102533155651,10.066717918137));
#10388=CARTESIAN_POINT('Ctrl Pts',(-7.08594454455926,38.4213969986079,9.90396913897554));
#10389=CARTESIAN_POINT('Ctrl Pts',(-7.31314931363975,38.4325406816507,9.7332572845071));
#10390=CARTESIAN_POINT('Ctrl Pts',(-7.54752711982908,38.4440361797206,9.55715591963368));
#10391=CARTESIAN_POINT('Ctrl Pts',(-7.77554672721654,38.4555316777905,9.37258068116194));
#10392=CARTESIAN_POINT('Ctrl Pts',(-7.99660336458607,38.4670271758604,9.18002096291129));
#10393=CARTESIAN_POINT('Ctrl Pts',(-8.21090626771047,38.4781714628565,8.99334433950392));
#10394=CARTESIAN_POINT('Ctrl Pts',(-8.41866514053532,38.4893157498526,8.79916406173953));
#10395=CARTESIAN_POINT('Ctrl Pts',(-8.61936384853658,38.5004600368487,8.59796586970085));
#10396=CARTESIAN_POINT('Ctrl Pts',(-8.82955005566236,38.5121311404555,8.38725656675452));
#10397=CARTESIAN_POINT('Ctrl Pts',(-9.03199227177261,38.5238022440623,8.16885006407581));
#10398=CARTESIAN_POINT('Ctrl Pts',(-9.22614151152845,38.535473347669,7.94334709421989));
#10399=CARTESIAN_POINT('Ctrl Pts',(-9.42029075128428,38.5471444512758,7.71784412436397));
#10400=CARTESIAN_POINT('Ctrl Pts',(-9.60614680231032,38.5588155548826,7.4852449475224));
#10401=CARTESIAN_POINT('Ctrl Pts',(-9.78320885115772,38.5704866584894,7.24619036629795));
#10402=CARTESIAN_POINT('Ctrl Pts',(-9.95232519265855,38.5816340181642,7.01786342408272));
#10403=CARTESIAN_POINT('Ctrl Pts',(-10.1134700589456,38.592781377839,6.78357934184873));
#10404=CARTESIAN_POINT('Ctrl Pts',(-10.2662355845482,38.6039287375138,6.54391757073364));
#10405=CARTESIAN_POINT('Ctrl Pts',(-10.4189751284731,38.6150742012955,6.30429656022115));
#10406=CARTESIAN_POINT('Ctrl Pts',(-10.5633380336435,38.6262196650772,6.05929991170006));
#10407=CARTESIAN_POINT('Ctrl Pts',(-10.6989600913802,38.6373651288589,5.80953554193913));
#10408=CARTESIAN_POINT('Ctrl Pts',(-10.8345670610239,38.6485093526963,5.55979895872045));
#10409=CARTESIAN_POINT('Ctrl Pts',(-10.9614349977632,38.6596535765337,5.30529594776737));
#10410=CARTESIAN_POINT('Ctrl Pts',(-11.0792453455692,38.6707978003711,5.04665957071439));
#10411=CARTESIAN_POINT('Ctrl Pts',(-11.20076485087,38.682292890513,4.77988024973298));
#10412=CARTESIAN_POINT('Ctrl Pts',(-11.3126470548315,38.693787980655,4.50870334116523));
#10413=CARTESIAN_POINT('Ctrl Pts',(-11.4145951579047,38.7052830707969,4.23384785167571));
#10414=CARTESIAN_POINT('Ctrl Pts',(-11.5134367040608,38.7164278831925,3.96736774334894));
#10415=CARTESIAN_POINT('Ctrl Pts',(-11.6029405119847,38.7275726955881,3.69743018378309));
#10416=CARTESIAN_POINT('Ctrl Pts',(-11.6828857891978,38.7387175079836,3.42470873017855));
#10417=CARTESIAN_POINT('Ctrl Pts',(-11.7666000466156,38.7503877369988,3.13912995972093));
#10418=CARTESIAN_POINT('Ctrl Pts',(-11.8398327384508,38.7620579660139,2.85049879505899));
#10419=CARTESIAN_POINT('Ctrl Pts',(-11.9023893162427,38.7737281950291,2.55960520678335));
#10420=CARTESIAN_POINT('Ctrl Pts',(-11.9649458940345,38.7853984240442,2.26871161850769));
#10421=CARTESIAN_POINT('Ctrl Pts',(-12.0168262958164,38.7970686530593,1.97555593644156));
#10422=CARTESIAN_POINT('Ctrl Pts',(-12.0578974154622,38.8087388820745,1.68094026312326));
#10423=CARTESIAN_POINT('Ctrl Pts',(-12.0989059319874,38.8203913226104,1.38677366109214));
#10424=CARTESIAN_POINT('Ctrl Pts',(-12.1291472088389,38.8320437631464,1.0910923577));
#10425=CARTESIAN_POINT('Ctrl Pts',(-12.1485371754145,38.8436962036824,0.794666437929197));
#10426=CARTESIAN_POINT('Ctrl Pts',(-12.1658307293892,38.8540888007279,0.530289621029534));
#10427=CARTESIAN_POINT('Ctrl Pts',(-12.1744932675459,38.8644813977734,0.265320699870421));
#10428=CARTESIAN_POINT('Ctrl Pts',(-12.174499996076,38.8748739948188,0.000309105303522327));
#10429=CARTESIAN_POINT('Ctrl Pts',(7.93208051261574,20.0005837734501,-6.87965285147223));
#10430=CARTESIAN_POINT('Ctrl Pts',(9.07668263151754,20.0800217251941,-5.55995978932681));
#10431=CARTESIAN_POINT('Ctrl Pts',(10.6930139230921,20.2388770847998,-2.33991560351307));
#10432=CARTESIAN_POINT('Ctrl Pts',(10.5082240576505,20.4771498522672,3.06359191036739));
#10433=CARTESIAN_POINT('Ctrl Pts',(7.7610444220363,20.7154020758523,7.71831352629605));
#10434=CARTESIAN_POINT('Ctrl Pts',(3.12105089944607,20.9536542994374,10.4913407524211));
#10435=CARTESIAN_POINT('Ctrl Pts',(-2.28002032107308,21.1919065230225,10.7055409903604));
#10436=CARTESIAN_POINT('Ctrl Pts',(-7.12508829170954,21.4301587466076,8.30910926435329));
#10437=CARTESIAN_POINT('Ctrl Pts',(-10.2325364964883,21.6684109701927,3.88625151956404));
#10438=CARTESIAN_POINT('Ctrl Pts',(-10.8445684035224,21.9066631937778,-1.48431630400501));
#10439=CARTESIAN_POINT('Ctrl Pts',(-8.81191628458542,22.1449154173629,-6.49291954617507));
#10440=CARTESIAN_POINT('Ctrl Pts',(-4.63029122950666,22.383167640948,-9.91807630779845));
#10441=CARTESIAN_POINT('Ctrl Pts',(0.680530483683632,22.6214198645331,-10.9245019479025));
#10442=CARTESIAN_POINT('Ctrl Pts',(5.82538981214024,22.8596720881182,-9.26675138990805));
#10443=CARTESIAN_POINT('Ctrl Pts',(9.54960316733972,23.0979243117033,-5.34910593878247));
#10444=CARTESIAN_POINT('Ctrl Pts',(10.9449409563647,23.3361765352884,-0.126965784354505));
#10445=CARTESIAN_POINT('Ctrl Pts',(9.67112030848427,23.5744287588735,5.12613742673736));
#10446=CARTESIAN_POINT('Ctrl Pts',(6.03878961601208,23.8126809824586,9.12912226706514));
#10447=CARTESIAN_POINT('Ctrl Pts',(0.933770628914186,24.0509332060437,10.9057748640797));
#10448=CARTESIAN_POINT('Ctrl Pts',(-4.3989683509955,24.2891854296288,10.0228204950036));
#10449=CARTESIAN_POINT('Ctrl Pts',(-8.65892458966233,24.5274376532139,6.69558646125051));
#10450=CARTESIAN_POINT('Ctrl Pts',(-10.8072164379082,24.765689876799,1.7354901366115));
#10451=CARTESIAN_POINT('Ctrl Pts',(-10.3199368707579,25.0039421003841,-3.64784266760709));
#10452=CARTESIAN_POINT('Ctrl Pts',(-7.31591945824722,25.2421943239692,-8.14157083244356));
#10453=CARTESIAN_POINT('Ctrl Pts',(-2.52775824622543,25.4804465475543,-10.6498024110112));
#10454=CARTESIAN_POINT('Ctrl Pts',(2.8768510043701,25.7186987711394,-10.5608513596116));
#10455=CARTESIAN_POINT('Ctrl Pts',(7.5798784633816,25.9569509947245,-7.89641029984006));
#10456=CARTESIAN_POINT('Ctrl Pts',(10.4343900608802,26.1952032183096,-3.30626030429192));
#10457=CARTESIAN_POINT('Ctrl Pts',(10.7442519485492,26.4334554418947,2.09019214633302));
#10458=CARTESIAN_POINT('Ctrl Pts',(8.43389766221118,26.6717076654798,6.9769064323582));
#10459=CARTESIAN_POINT('Ctrl Pts',(4.06675662420537,26.9099598890649,10.1621525132199));
#10460=CARTESIAN_POINT('Ctrl Pts',(-1.29215020014935,27.14821211265,10.8691398464998));
#10461=CARTESIAN_POINT('Ctrl Pts',(-6.33593849695176,27.3864643362351,8.92545441450063));
#10462=CARTESIAN_POINT('Ctrl Pts',(-9.83457236079029,27.6247165598202,4.80510557874393));
#10463=CARTESIAN_POINT('Ctrl Pts',(-10.934834919905,27.8629687834053,-0.487071264723974));
#10464=CARTESIAN_POINT('Ctrl Pts',(-9.36840356171729,28.1012210069904,-5.66046533840602));
#10465=CARTESIAN_POINT('Ctrl Pts',(-5.51728615423312,28.3394732305755,-9.45343358969647));
#10466=CARTESIAN_POINT('Ctrl Pts',(-0.320660237907371,28.5777254541606,
-10.9409793964854));
#10467=CARTESIAN_POINT('Ctrl Pts',(4.95416555177833,28.8159776777457,-9.76033282363192));
#10468=CARTESIAN_POINT('Ctrl Pts',(9.02081186376675,29.0542299013308,-6.1994198487454));
#10469=CARTESIAN_POINT('Ctrl Pts',(10.8875398137095,29.2924821249159,-1.12664543996017));
#10470=CARTESIAN_POINT('Ctrl Pts',(10.0991077719128,29.530734348501,4.22088561249689));
#10471=CARTESIAN_POINT('Ctrl Pts',(6.84779179425367,29.7689865720861,8.53906322057902));
#10472=CARTESIAN_POINT('Ctrl Pts',(1.92649498392104,30.0072387956712,10.7748072010324));
#10473=CARTESIAN_POINT('Ctrl Pts',(-3.46461892863268,30.2454910192563,10.3828834541207));
#10474=CARTESIAN_POINT('Ctrl Pts',(-8.0108112405926,30.4837432428414,7.45887098762869));
#10475=CARTESIAN_POINT('Ctrl Pts',(-10.6033954949622,30.7219954664265,2.71585292678186));
#10476=CARTESIAN_POINT('Ctrl Pts',(-10.6101144412331,30.9602476900116,-2.68948409298712));
#10477=CARTESIAN_POINT('Ctrl Pts',(-8.02932952031574,31.1984999135967,-7.43893275925249));
#10478=CARTESIAN_POINT('Ctrl Pts',(-3.49042046230085,31.4367521371818,-10.3742381955904));
#10479=CARTESIAN_POINT('Ctrl Pts',(1.89970245342874,31.6750043607669,-10.7795632439784));
#10480=CARTESIAN_POINT('Ctrl Pts',(6.8265421998787,31.913256584352,-8.55606070196843));
#10481=CARTESIAN_POINT('Ctrl Pts',(10.0885832827944,32.1515088079371,-4.24597933209919));
#10482=CARTESIAN_POINT('Ctrl Pts',(10.8903070521443,32.3897610315222,1.09957512363163));
#10483=CARTESIAN_POINT('Ctrl Pts',(9.03619597933803,32.6280132551074,6.1769746126635));
#10484=CARTESIAN_POINT('Ctrl Pts',(4.97841479809776,32.8662654786924,9.7479864197984));
#10485=CARTESIAN_POINT('Ctrl Pts',(-0.293459559412273,33.1045177022776,
10.9417427601586));
#10486=CARTESIAN_POINT('Ctrl Pts',(-5.49376751214475,33.3427699258626,9.46712055827954));
#10487=CARTESIAN_POINT('Ctrl Pts',(-9.35430248110292,33.5810221494478,5.68373805118744));
#10488=CARTESIAN_POINT('Ctrl Pts',(-10.9335902515748,33.8192743730328,0.514254171769246));
#10489=CARTESIAN_POINT('Ctrl Pts',(-9.84648764379592,34.0575265966179,-4.78064161206769));
#10490=CARTESIAN_POINT('Ctrl Pts',(-6.35810793409936,34.295778820203,-8.90967545092836));
#10491=CARTESIAN_POINT('Ctrl Pts',(-1.3191672989035,34.5340310437881,-10.8658939245695));
#10492=CARTESIAN_POINT('Ctrl Pts',(4.04148056253829,34.7722832673732,-10.1722312205807));
#10493=CARTESIAN_POINT('Ctrl Pts',(8.41652674720532,35.0105354909583,-6.9978518601521));
#10494=CARTESIAN_POINT('Ctrl Pts',(10.7390224500958,35.2487877145434,-2.11689630296171));
#10495=CARTESIAN_POINT('Ctrl Pts',(10.4425773045532,35.4870399381285,3.28030979990781));
#10496=CARTESIAN_POINT('Ctrl Pts',(7.59948581375965,35.7252921617136,7.87754203452586));
#10497=CARTESIAN_POINT('Ctrl Pts',(2.90309678978814,35.9635443852987,10.5536667643604));
#10498=CARTESIAN_POINT('Ctrl Pts',(-2.50127462534687,36.2017966088839,10.6560536034062));
#10499=CARTESIAN_POINT('Ctrl Pts',(-7.29565659631146,36.4400488324689,8.15973332519128));
#10500=CARTESIAN_POINT('Ctrl Pts',(-10.310836309689,36.678301056054,3.67348714751023));
#10501=CARTESIAN_POINT('Ctrl Pts',(-10.811497527272,36.9165532796391,-1.70861762580354));
#10502=CARTESIAN_POINT('Ctrl Pts',(-8.67554332886272,37.1548055032242,-6.67403935727874));
#10503=CARTESIAN_POINT('Ctrl Pts',(-4.42387183430699,37.3930577268093,-10.0118535213315));
#10504=CARTESIAN_POINT('Ctrl Pts',(0.906655509484174,37.6313099503944,-10.9080625518847));
#10505=CARTESIAN_POINT('Ctrl Pts',(6.01607574523276,37.8695621739795,-9.14410671556304));
#10506=CARTESIAN_POINT('Ctrl Pts',(9.65834638546719,38.1078143975646,-5.15016435505535));
#10507=CARTESIAN_POINT('Ctrl Pts',(10.9452233105833,38.3460666211498,0.0997558540279738));
#10508=CARTESIAN_POINT('Ctrl Pts',(9.56287066352806,38.5843188447348,5.32534873881454));
#10509=CARTESIAN_POINT('Ctrl Pts',(5.84841145753922,38.82257106832,9.25224060771052));
#10510=CARTESIAN_POINT('Ctrl Pts',(0.70768278248567,39.060823291905,10.9227763791256));
#10511=CARTESIAN_POINT('Ctrl Pts',(-4.60561153353682,39.2990755154902,9.92955670850569));
#10512=CARTESIAN_POINT('Ctrl Pts',(-8.79576482446728,39.5373277390752,6.51480629675831));
#10513=CARTESIAN_POINT('Ctrl Pts',(-10.8408098726847,39.7755799626604,1.51127160533644));
#10514=CARTESIAN_POINT('Ctrl Pts',(-10.2422364118163,40.0138321862454,-3.86080079579494));
#10515=CARTESIAN_POINT('Ctrl Pts',(-7.14558203450444,40.2520844098305,-8.29137091192963));
#10516=CARTESIAN_POINT('Ctrl Pts',(-2.30691296609827,40.4903366334156,-10.6998374196014));
#10517=CARTESIAN_POINT('Ctrl Pts',(3.09555850011698,40.7285888570008,-10.4990832245953));
#10518=CARTESIAN_POINT('Ctrl Pts',(6.19188889114855,40.8874236727241,-8.65783810040184));
#10519=CARTESIAN_POINT('Ctrl Pts',(7.42649694513297,40.9668410805858,-7.4225782431051));
#10520=CARTESIAN_POINT('Ctrl Pts',(8.35397305039485,19.6781514844946,-7.24556872889312));
#10521=CARTESIAN_POINT('Ctrl Pts',(9.5594544167933,19.7575894362386,-5.8556836592167));
#10522=CARTESIAN_POINT('Ctrl Pts',(11.2617553489193,19.9164447958442,-2.46437134127127));
#10523=CARTESIAN_POINT('Ctrl Pts',(11.0671368558985,20.1547175633116,3.22653863837005));
#10524=CARTESIAN_POINT('Ctrl Pts',(8.17383986981593,20.3929697868967,8.12883619759329));
#10525=CARTESIAN_POINT('Ctrl Pts',(3.28705376368968,20.6312220104819,11.0493555592179));
#10526=CARTESIAN_POINT('Ctrl Pts',(-2.40129034069979,20.869474234067,11.2749487074831));
#10527=CARTESIAN_POINT('Ctrl Pts',(-7.5040584214893,21.1077264576521,8.75105525678824));
#10528=CARTESIAN_POINT('Ctrl Pts',(-10.776785988605,21.3459786812371,4.0929539746676));
#10529=CARTESIAN_POINT('Ctrl Pts',(-11.4213707289154,21.5842309048223,-1.5632643140974));
#10530=CARTESIAN_POINT('Ctrl Pts',(-9.28060564270375,21.8224831284073,-6.83826580187362));
#10531=CARTESIAN_POINT('Ctrl Pts',(-4.87656776620671,22.0607353519925,-10.4456002501902));
#10532=CARTESIAN_POINT('Ctrl Pts',(0.716726628231168,22.2989875755775,-11.505555789129));
#10533=CARTESIAN_POINT('Ctrl Pts',(6.13523140886729,22.5372397991627,-9.75963257721301));
#10534=CARTESIAN_POINT('Ctrl Pts',(10.0575287120496,22.7754920227477,-5.63361488643787));
#10535=CARTESIAN_POINT('Ctrl Pts',(11.5270819102518,23.0137442463329,-0.133718857131222));
#10536=CARTESIAN_POINT('Ctrl Pts',(10.1855091228218,23.2519964699179,5.39878709595479));
#10537=CARTESIAN_POINT('Ctrl Pts',(6.35998154947282,23.4902486935031,9.61468321854846));
#10538=CARTESIAN_POINT('Ctrl Pts',(0.983436143492576,23.7285009170882,11.4858326467177));
#10539=CARTESIAN_POINT('Ctrl Pts',(-4.63294125611917,23.9667531406733,10.5559155849508));
#10540=CARTESIAN_POINT('Ctrl Pts',(-9.119476605462,24.2050053642584,7.05171219138697));
#10541=CARTESIAN_POINT('Ctrl Pts',(-11.3820320820593,24.4432575878435,1.82779761342809));
#10542=CARTESIAN_POINT('Ctrl Pts',(-10.868835025435,24.6815098114285,-3.84186460145004));
#10543=CARTESIAN_POINT('Ctrl Pts',(-7.70503954112062,24.9197620350137,-8.57460576880672));
#10544=CARTESIAN_POINT('Ctrl Pts',(-2.66220498308041,25.1580142585987,-11.216245497271));
#10545=CARTESIAN_POINT('Ctrl Pts',(3.02986533259278,25.3962664821839,-11.1225633056928));
#10546=CARTESIAN_POINT('Ctrl Pts',(7.98303803241107,25.6345187057689,-8.31640560566758));
#10547=CARTESIAN_POINT('Ctrl Pts',(10.9893757668322,25.8727709293541,-3.48211411063157));
#10548=CARTESIAN_POINT('Ctrl Pts',(11.3157186291889,26.1110231529392,2.20136556012525));
#10549=CARTESIAN_POINT('Ctrl Pts',(8.88248091630454,26.3492753765243,7.34799504598405));
#10550=CARTESIAN_POINT('Ctrl Pts',(4.28305980846921,26.5875276001094,10.702658412811));
#10551=CARTESIAN_POINT('Ctrl Pts',(-1.3608772543271,26.8257798236945,11.4472490810218));
#10552=CARTESIAN_POINT('Ctrl Pts',(-6.67293522403238,27.0640320472796,9.4001826535517));
#10553=CARTESIAN_POINT('Ctrl Pts',(-10.3576548843057,27.3022842708646,5.06068016396008));
#10554=CARTESIAN_POINT('Ctrl Pts',(-11.5164383526005,27.5405364944498,-0.512977674981265));
#10555=CARTESIAN_POINT('Ctrl Pts',(-9.86669143805761,27.7787887180349,-5.96153491061126));
#10556=CARTESIAN_POINT('Ctrl Pts',(-5.8107402932274,28.0170409416199,-9.95624405430786));
#10557=CARTESIAN_POINT('Ctrl Pts',(-0.337715556662699,28.2552931652051,
-11.5229096424065));
#10558=CARTESIAN_POINT('Ctrl Pts',(5.21766835837407,28.4935453887901,-10.2794666849161));
#10559=CARTESIAN_POINT('Ctrl Pts',(9.50061198732568,28.7317976123753,-6.52915540407486));
#10560=CARTESIAN_POINT('Ctrl Pts',(11.4666277080989,28.9700498359604,-1.1865696052641));
#10561=CARTESIAN_POINT('Ctrl Pts',(10.6362604395415,29.2083020595455,4.44538662958811));
#10562=CARTESIAN_POINT('Ctrl Pts',(7.21201304158794,29.4465542831306,8.99324003417244));
#10563=CARTESIAN_POINT('Ctrl Pts',(2.02896165158692,29.6848065067157,11.3478990584454));
#10564=CARTESIAN_POINT('Ctrl Pts',(-3.64889553423618,29.9230587303008,10.9351296199225));
#10565=CARTESIAN_POINT('Ctrl Pts',(-8.43689131864875,30.1613109538859,7.85559439518017));
#10566=CARTESIAN_POINT('Ctrl Pts',(-11.1673702840897,30.3995631774709,2.86030406815548));
#10567=CARTESIAN_POINT('Ctrl Pts',(-11.1744465985554,30.6378154010561,-2.83253272537331));
#10568=CARTESIAN_POINT('Ctrl Pts',(-8.45639455106058,30.8760676246412,-7.83459568970025));
#10569=CARTESIAN_POINT('Ctrl Pts',(-3.67606940325828,31.1143198482262,-10.9260245362485));
#10570=CARTESIAN_POINT('Ctrl Pts',(2.00074407647172,31.3525720718114,-11.3529080664269));
#10571=CARTESIAN_POINT('Ctrl Pts',(7.18963322100266,31.5908242953965,-9.01114157982946));
#10572=CARTESIAN_POINT('Ctrl Pts',(10.6251761725167,31.8290765189816,-4.47181503723706));
#10573=CARTESIAN_POINT('Ctrl Pts',(11.4695421307741,32.0673287425667,1.15805946940319));
#10574=CARTESIAN_POINT('Ctrl Pts',(9.51681435525202,32.3055809661518,6.50551634783486));
#10575=CARTESIAN_POINT('Ctrl Pts',(5.24320737678452,32.5438331897369,10.2664635989375));
#10576=CARTESIAN_POINT('Ctrl Pts',(-0.309068124915233,32.782085413322,11.5237136079667));
#10577=CARTESIAN_POINT('Ctrl Pts',(-5.78597073852161,33.020337636907,9.97065900716958));
#10578=CARTESIAN_POINT('Ctrl Pts',(-9.85184034731961,33.2585898604922,5.98604545548992));
#10579=CARTESIAN_POINT('Ctrl Pts',(-11.515127482688,33.4968420840773,0.541606390048691));
#10580=CARTESIAN_POINT('Ctrl Pts',(-10.3702039189452,33.7350943076624,-5.03491500461833));
#10581=CARTESIAN_POINT('Ctrl Pts',(-6.69628381210821,33.9733465312475,-9.38356443639719));
#10582=CARTESIAN_POINT('Ctrl Pts',(-1.3893313420703,34.2115987548326,-11.4438305145706));
#10583=CARTESIAN_POINT('Ctrl Pts',(4.25643936032185,34.4498509784177,-10.7132731877799));
#10584=CARTESIAN_POINT('Ctrl Pts',(8.8641860747949,34.6881032020028,-7.37005452193625));
#10585=CARTESIAN_POINT('Ctrl Pts',(11.3102109834865,34.9263554255879,-2.22949006093621));
#10586=CARTESIAN_POINT('Ctrl Pts',(10.9979984746946,35.164607649173,3.45478334741955));
#10587=CARTESIAN_POINT('Ctrl Pts',(8.00368826111052,35.4028598727581,8.29653377258524));
#10588=CARTESIAN_POINT('Ctrl Pts',(3.05750708228506,35.6411120963432,11.114996575248));
#10589=CARTESIAN_POINT('Ctrl Pts',(-2.63431274790397,35.8793643199283,11.2228291789063));
#10590=CARTESIAN_POINT('Ctrl Pts',(-7.68369893542883,36.1176165435133,8.59373429059882));
#10591=CARTESIAN_POINT('Ctrl Pts',(-10.8592504225313,36.3558687670984,3.86887306331091));
#10592=CARTESIAN_POINT('Ctrl Pts',(-11.3865408745652,36.5941209906836,-1.79949580399373));
#10593=CARTESIAN_POINT('Ctrl Pts',(-9.13697926434082,36.8323732142686,-7.02901903722545));
#10594=CARTESIAN_POINT('Ctrl Pts',(-4.65916930916454,37.0706254378537,-10.544365298446));
#10595=CARTESIAN_POINT('Ctrl Pts',(0.954878821536958,37.3088776614389,-11.4882420123614));
#10596=CARTESIAN_POINT('Ctrl Pts',(6.33605957035795,37.547129885024,-9.63046466185671));
#10597=CARTESIAN_POINT('Ctrl Pts',(10.1720557787132,37.7853821086091,-5.42409197168482));
#10598=CARTESIAN_POINT('Ctrl Pts',(11.5273792823635,38.0236343321941,0.105061681464705));
#10599=CARTESIAN_POINT('Ctrl Pts',(10.0715018815638,38.2618865557793,5.60859408540474));
#10600=CARTESIAN_POINT('Ctrl Pts',(6.15947753255868,38.5001387793643,9.74434999363035));
#10601=CARTESIAN_POINT('Ctrl Pts',(0.74532310706011,38.7383910029495,11.5037384405739));
#10602=CARTESIAN_POINT('Ctrl Pts',(-4.85057540333342,38.9766432265345,10.4576912719547));
#10603=CARTESIAN_POINT('Ctrl Pts',(-9.26359511660826,39.2148954501196,6.86131666781508));
#10604=CARTESIAN_POINT('Ctrl Pts',(-11.4174122888469,39.4531476737047,1.59165331752844));
#10605=CARTESIAN_POINT('Ctrl Pts',(-10.7870018243007,39.6913998972899,-4.06614957446744));
#10606=CARTESIAN_POINT('Ctrl Pts',(-7.52564218816163,39.929652120875,-8.73237343455133));
#10607=CARTESIAN_POINT('Ctrl Pts',(-2.42961335525277,40.1679043444601,-11.268941774455));
#10608=CARTESIAN_POINT('Ctrl Pts',(3.26020547128437,40.4061565680452,-11.0575098390168));
#10609=CARTESIAN_POINT('Ctrl Pts',(6.52122388891844,40.5649913837685,-9.11833232786835));
#10610=CARTESIAN_POINT('Ctrl Pts',(7.82149843786967,40.6444087916303,-7.81737130740481));
#10611=CARTESIAN_POINT('Ctrl Pts',(8.77586558817396,19.3557191955389,-7.61148460631401));
#10612=CARTESIAN_POINT('Ctrl Pts',(10.0422262020691,19.4351571472829,-6.15140752910658));
#10613=CARTESIAN_POINT('Ctrl Pts',(11.8304967747464,19.5940125068886,-2.58882707902948));
#10614=CARTESIAN_POINT('Ctrl Pts',(11.6260496541463,19.832285274356,3.38948536637273));
#10615=CARTESIAN_POINT('Ctrl Pts',(8.58663531759557,20.0705374979411,8.53935886889055));
#10616=CARTESIAN_POINT('Ctrl Pts',(3.45305662793327,20.3087897215262,11.6073703660148));
#10617=CARTESIAN_POINT('Ctrl Pts',(-2.52256036032647,20.5470419451113,11.8443564246056));
#10618=CARTESIAN_POINT('Ctrl Pts',(-7.8830285512691,20.7852941686964,9.1930012492232));
#10619=CARTESIAN_POINT('Ctrl Pts',(-11.3210354807218,21.0235463922815,4.29965642977116));
#10620=CARTESIAN_POINT('Ctrl Pts',(-11.9981730543084,21.2617986158666,-1.64221232418978));
#10621=CARTESIAN_POINT('Ctrl Pts',(-9.74929500082207,21.5000508394517,-7.18361205757219));
#10622=CARTESIAN_POINT('Ctrl Pts',(-5.12284430290676,21.7383030630368,-10.973124192582));
#10623=CARTESIAN_POINT('Ctrl Pts',(0.752922772778707,21.9765552866219,-12.0866096303556));
#10624=CARTESIAN_POINT('Ctrl Pts',(6.44507300559435,22.214807510207,-10.2525137645179));
#10625=CARTESIAN_POINT('Ctrl Pts',(10.5654542567593,22.4530597337921,-5.91812383409328));
#10626=CARTESIAN_POINT('Ctrl Pts',(12.1092228641389,22.6913119573772,-0.140471929907933));
#10627=CARTESIAN_POINT('Ctrl Pts',(10.6998979371592,22.9295641809623,5.67143676517222));
#10628=CARTESIAN_POINT('Ctrl Pts',(6.6811734829336,23.1678164045474,10.1002441700318));
#10629=CARTESIAN_POINT('Ctrl Pts',(1.03310165807095,23.4060686281325,12.0658904293558));
#10630=CARTESIAN_POINT('Ctrl Pts',(-4.86691416124282,23.6443208517176,11.089010674898));
#10631=CARTESIAN_POINT('Ctrl Pts',(-9.5800286212617,23.8825730753027,7.40783792152343));
#10632=CARTESIAN_POINT('Ctrl Pts',(-11.9568477262104,24.1208252988878,1.92010509024469));
#10633=CARTESIAN_POINT('Ctrl Pts',(-11.4177331801119,24.3590775224729,-4.03588653529299));
#10634=CARTESIAN_POINT('Ctrl Pts',(-8.09415962399401,24.597329746058,-9.00764070516989));
#10635=CARTESIAN_POINT('Ctrl Pts',(-2.79665171993538,24.8355819696431,-11.7826885835309));
#10636=CARTESIAN_POINT('Ctrl Pts',(3.18287966081545,25.0738341932282,-11.6842752517741));
#10637=CARTESIAN_POINT('Ctrl Pts',(8.38619760144056,25.3120864168133,-8.73640091149512));
#10638=CARTESIAN_POINT('Ctrl Pts',(11.5443614727842,25.5503386403984,-3.65796791697122));
#10639=CARTESIAN_POINT('Ctrl Pts',(11.8871853098286,25.7885908639836,2.3125389739175));
#10640=CARTESIAN_POINT('Ctrl Pts',(9.33106417039787,26.0268430875686,7.71908365960987));
#10641=CARTESIAN_POINT('Ctrl Pts',(4.49936299273306,26.2650953111537,11.2431643124021));
#10642=CARTESIAN_POINT('Ctrl Pts',(-1.42960430850484,26.5033475347388,12.0253583155439));
#10643=CARTESIAN_POINT('Ctrl Pts',(-7.00993195111298,26.7415997583239,9.87491089260278));
#10644=CARTESIAN_POINT('Ctrl Pts',(-10.880737407821,26.979851981909,5.31625474917623));
#10645=CARTESIAN_POINT('Ctrl Pts',(-12.098041785296,27.2181042054941,-0.538884085238557));
#10646=CARTESIAN_POINT('Ctrl Pts',(-10.3649793143979,27.4563564290792,-6.26260448281651));
#10647=CARTESIAN_POINT('Ctrl Pts',(-6.10419443222168,27.6946086526643,-10.4590545189192));
#10648=CARTESIAN_POINT('Ctrl Pts',(-0.354770875418026,27.9328608762494,
-12.1048398883276));
#10649=CARTESIAN_POINT('Ctrl Pts',(5.4811711649698,28.1711130998345,-10.7986005462002));
#10650=CARTESIAN_POINT('Ctrl Pts',(9.98041211088462,28.4093653234196,-6.85889095940433));
#10651=CARTESIAN_POINT('Ctrl Pts',(12.0457156024881,28.6476175470047,-1.24649377056803));
#10652=CARTESIAN_POINT('Ctrl Pts',(11.1734131071702,28.8858697705898,4.66988764667932));
#10653=CARTESIAN_POINT('Ctrl Pts',(7.57623428892219,29.1241219941749,9.44741684776587));
#10654=CARTESIAN_POINT('Ctrl Pts',(2.13142831925279,29.36237421776,11.9209909158584));
#10655=CARTESIAN_POINT('Ctrl Pts',(-3.83317213983967,29.6006264413451,11.4873757857244));
#10656=CARTESIAN_POINT('Ctrl Pts',(-8.86297139670491,29.8388786649302,8.25231780273166));
#10657=CARTESIAN_POINT('Ctrl Pts',(-11.7313450732173,30.0771308885153,3.00475520952911));
#10658=CARTESIAN_POINT('Ctrl Pts',(-11.7387787558777,30.3153831121004,-2.97558135775951));
#10659=CARTESIAN_POINT('Ctrl Pts',(-8.88345958180541,30.5536353356855,-8.23025862014802));
#10660=CARTESIAN_POINT('Ctrl Pts',(-3.86171834421572,30.7918875592706,-11.4778108769068));
#10661=CARTESIAN_POINT('Ctrl Pts',(2.10178569951469,31.0301397828557,-11.9262528888754));
#10662=CARTESIAN_POINT('Ctrl Pts',(7.55272424212662,31.2683920064408,-9.46622245769049));
#10663=CARTESIAN_POINT('Ctrl Pts',(11.1617690622389,31.5066442300259,-4.69765074237494));
#10664=CARTESIAN_POINT('Ctrl Pts',(12.0487772094039,31.744896453611,1.21654381517477));
#10665=CARTESIAN_POINT('Ctrl Pts',(9.99743273116598,31.9831486771961,6.83405808300622));
#10666=CARTESIAN_POINT('Ctrl Pts',(5.50799995547129,32.2214009007812,10.7849407780765));
#10667=CARTESIAN_POINT('Ctrl Pts',(-0.324676690418206,32.4596531243664,
12.1056844557749));
#10668=CARTESIAN_POINT('Ctrl Pts',(-6.07817396489844,32.6979053479514,10.4741974560597));
#10669=CARTESIAN_POINT('Ctrl Pts',(-10.3493782135363,32.9361575715365,6.28835285979241));
#10670=CARTESIAN_POINT('Ctrl Pts',(-12.0966647138013,33.1744097951216,0.568958608328141));
#10671=CARTESIAN_POINT('Ctrl Pts',(-10.8939201940946,33.4126620187067,-5.28918839716898));
#10672=CARTESIAN_POINT('Ctrl Pts',(-7.03445969011705,33.6509142422919,-9.85745342186599));
#10673=CARTESIAN_POINT('Ctrl Pts',(-1.45949538523709,33.8891664658769,-12.0217671045718));
#10674=CARTESIAN_POINT('Ctrl Pts',(4.4713981581054,34.127418689462,-11.2543151549789));
#10675=CARTESIAN_POINT('Ctrl Pts',(9.31184540238453,34.3656709130471,-7.7422571837204));
#10676=CARTESIAN_POINT('Ctrl Pts',(11.8813995168772,34.6039231366322,-2.34208381891072));
#10677=CARTESIAN_POINT('Ctrl Pts',(11.5534196448359,34.8421753602173,3.62925689493129));
#10678=CARTESIAN_POINT('Ctrl Pts',(8.4078907084614,35.0804275838025,8.71552551064461));
#10679=CARTESIAN_POINT('Ctrl Pts',(3.21191737478198,35.3186798073875,11.6763263861354));
#10680=CARTESIAN_POINT('Ctrl Pts',(-2.76735087046106,35.5569320309727,11.7896047544065));
#10681=CARTESIAN_POINT('Ctrl Pts',(-8.07174127454621,35.7951842545577,9.0277352560064));
#10682=CARTESIAN_POINT('Ctrl Pts',(-11.4076645353736,36.0334364781429,4.06425897911157));
#10683=CARTESIAN_POINT('Ctrl Pts',(-11.9615842218583,36.2716887017279,-1.89037398218391));
#10684=CARTESIAN_POINT('Ctrl Pts',(-9.59841519981894,36.5099409253131,-7.38399871717217));
#10685=CARTESIAN_POINT('Ctrl Pts',(-4.89446678402209,36.7481931488981,-11.0768770755603));
#10686=CARTESIAN_POINT('Ctrl Pts',(1.00310213358974,36.9864453724833,-12.0684214728383));
#10687=CARTESIAN_POINT('Ctrl Pts',(6.65604339548311,37.2246975960683,-10.1168226081503));
#10688=CARTESIAN_POINT('Ctrl Pts',(10.6857651719592,37.4629498196534,-5.69801958831428));
#10689=CARTESIAN_POINT('Ctrl Pts',(12.1095352541438,37.7012020432385,0.110367508901437));
#10690=CARTESIAN_POINT('Ctrl Pts',(10.5801330995995,37.9394542668236,5.89183943199493));
#10691=CARTESIAN_POINT('Ctrl Pts',(6.47054360757812,38.1777064904088,10.2364593795502));
#10692=CARTESIAN_POINT('Ctrl Pts',(0.782963431634552,38.4159587139938,12.0847005020222));
#10693=CARTESIAN_POINT('Ctrl Pts',(-5.09553927313002,38.654210937579,10.9858258354038));
#10694=CARTESIAN_POINT('Ctrl Pts',(-9.73142540874922,38.892463161164,7.20782703887185));
#10695=CARTESIAN_POINT('Ctrl Pts',(-11.9940147050091,39.1307153847492,1.67203502972045));
#10696=CARTESIAN_POINT('Ctrl Pts',(-11.3317672367851,39.3689676083343,-4.27149835313993));
#10697=CARTESIAN_POINT('Ctrl Pts',(-7.90570234181881,39.6072198319193,-9.17337595717302));
#10698=CARTESIAN_POINT('Ctrl Pts',(-2.55231374440726,39.8454720555045,-11.8380461293086));
#10699=CARTESIAN_POINT('Ctrl Pts',(3.42485244245177,40.0837242790895,-11.6159364534383));
#10700=CARTESIAN_POINT('Ctrl Pts',(6.85055888668833,40.2425590948129,-9.57882655533488));
#10701=CARTESIAN_POINT('Ctrl Pts',(8.21649993060639,40.3219765026746,-8.21216437170453));
#10702=CARTESIAN_POINT('Ctrl Pts',(9.19775812595308,19.0332869065834,-7.9774004837349));
#10703=CARTESIAN_POINT('Ctrl Pts',(10.5249979873448,19.1127248583274,-6.44713139899647));
#10704=CARTESIAN_POINT('Ctrl Pts',(12.3992382005735,19.2715802179331,-2.71328281678768));
#10705=CARTESIAN_POINT('Ctrl Pts',(12.1849624523942,19.5098529854005,3.5524320943754));
#10706=CARTESIAN_POINT('Ctrl Pts',(8.9994307653752,19.7481052089856,8.9498815401878));
#10707=CARTESIAN_POINT('Ctrl Pts',(3.61905949217688,19.9863574325707,12.1653851728116));
#10708=CARTESIAN_POINT('Ctrl Pts',(-2.64383037995317,20.2246096561558,12.4137641417282));
#10709=CARTESIAN_POINT('Ctrl Pts',(-8.26199868104885,20.4628618797409,9.63494724165815));
#10710=CARTESIAN_POINT('Ctrl Pts',(-11.8652849728387,20.701114103326,4.50635888487473));
#10711=CARTESIAN_POINT('Ctrl Pts',(-12.5749753797014,20.9393663269111,-1.72116033428216));
#10712=CARTESIAN_POINT('Ctrl Pts',(-10.2179843589404,21.1776185504962,-7.52895831327076));
#10713=CARTESIAN_POINT('Ctrl Pts',(-5.36912083960681,21.4158707740812,-11.5006481349737));
#10714=CARTESIAN_POINT('Ctrl Pts',(0.789118917326245,21.6541229976664,-12.6676634715821));
#10715=CARTESIAN_POINT('Ctrl Pts',(6.7549146023214,21.8923752212515,-10.7453949518229));
#10716=CARTESIAN_POINT('Ctrl Pts',(11.0733798014692,22.1306274448366,-6.20263278174869));
#10717=CARTESIAN_POINT('Ctrl Pts',(12.6913638180259,22.3688796684217,-0.147225002684643));
#10718=CARTESIAN_POINT('Ctrl Pts',(11.2142867514966,22.6071318920068,5.94408643438964));
#10719=CARTESIAN_POINT('Ctrl Pts',(7.00236541639435,22.8453841155919,10.585805121515));
#10720=CARTESIAN_POINT('Ctrl Pts',(1.08276717264934,23.083636339177,12.6459482119938));
#10721=CARTESIAN_POINT('Ctrl Pts',(-5.10088706636649,23.3218885627621,11.6221057648453));
#10722=CARTESIAN_POINT('Ctrl Pts',(-10.0405806370614,23.5601407863472,7.76396365165987));
#10723=CARTESIAN_POINT('Ctrl Pts',(-12.5316633703614,23.7983930099322,2.01241256706129));
#10724=CARTESIAN_POINT('Ctrl Pts',(-11.966631334789,24.0366452335174,-4.22990846913595));
#10725=CARTESIAN_POINT('Ctrl Pts',(-8.48327970686742,24.2748974571024,-9.44067564153303));
#10726=CARTESIAN_POINT('Ctrl Pts',(-2.93109845679036,24.5131496806876,-12.3491316697907));
#10727=CARTESIAN_POINT('Ctrl Pts',(3.33589398903813,24.7514019042726,-12.2459871978553));
#10728=CARTESIAN_POINT('Ctrl Pts',(8.78935717047004,24.9896541278578,-9.15639621732265));
#10729=CARTESIAN_POINT('Ctrl Pts',(12.0993471787362,25.2279063514429,-3.83382172331087));
#10730=CARTESIAN_POINT('Ctrl Pts',(12.4586519904683,25.466158575028,2.42371238770974));
#10731=CARTESIAN_POINT('Ctrl Pts',(9.77964742449122,25.7044107986131,8.09017227323569));
#10732=CARTESIAN_POINT('Ctrl Pts',(4.71566617699691,25.9426630221981,11.7836702119933));
#10733=CARTESIAN_POINT('Ctrl Pts',(-1.49833136268259,26.1809152457833,12.603467550066));
#10734=CARTESIAN_POINT('Ctrl Pts',(-7.34692867819359,26.4191674693684,10.3496391316539));
#10735=CARTESIAN_POINT('Ctrl Pts',(-11.4038199313364,26.6574196929535,5.57182933439236));
#10736=CARTESIAN_POINT('Ctrl Pts',(-12.6796452179915,26.8956719165386,-0.564790495495845));
#10737=CARTESIAN_POINT('Ctrl Pts',(-10.8632671907382,27.1339241401237,-6.56367405502175));
#10738=CARTESIAN_POINT('Ctrl Pts',(-6.39764857121597,27.3721763637088,-10.9618649835306));
#10739=CARTESIAN_POINT('Ctrl Pts',(-0.371826194173351,27.6104285872939,
-12.6867701342486));
#10740=CARTESIAN_POINT('Ctrl Pts',(5.74467397156553,27.848680810879,-11.3177344074843));
#10741=CARTESIAN_POINT('Ctrl Pts',(10.4602122344436,28.0869330344641,-7.1886265147338));
#10742=CARTESIAN_POINT('Ctrl Pts',(12.6248034968774,28.3251852580492,-1.30641793587195));
#10743=CARTESIAN_POINT('Ctrl Pts',(11.7105657747989,28.5634374816343,4.89438866377053));
#10744=CARTESIAN_POINT('Ctrl Pts',(7.94045553625644,28.8016897052194,9.90159366135931));
#10745=CARTESIAN_POINT('Ctrl Pts',(2.23389498691868,29.0399419288045,12.4940827732714));
#10746=CARTESIAN_POINT('Ctrl Pts',(-4.01744874544316,29.2781941523896,12.0396219515263));
#10747=CARTESIAN_POINT('Ctrl Pts',(-9.28905147476106,29.5164463759747,8.64904121028314));
#10748=CARTESIAN_POINT('Ctrl Pts',(-12.2953198623448,29.7546985995598,3.14920635090273));
#10749=CARTESIAN_POINT('Ctrl Pts',(-12.3031109132,29.9929508231448,-3.1186299901457));
#10750=CARTESIAN_POINT('Ctrl Pts',(-9.31052461255024,30.23120304673,-8.6259215505958));
#10751=CARTESIAN_POINT('Ctrl Pts',(-4.04736728517316,30.4694552703151,-12.0295972175649));
#10752=CARTESIAN_POINT('Ctrl Pts',(2.20282732255767,30.7077074939002,-12.4995977113237));
#10753=CARTESIAN_POINT('Ctrl Pts',(7.91581526325055,30.9459597174853,-9.92130333555153));
#10754=CARTESIAN_POINT('Ctrl Pts',(11.6983619519613,31.1842119410704,-4.92348644751282));
#10755=CARTESIAN_POINT('Ctrl Pts',(12.6280122880337,31.4224641646555,1.27502816094633));
#10756=CARTESIAN_POINT('Ctrl Pts',(10.47805110708,31.6607163882406,7.16259981817759));
#10757=CARTESIAN_POINT('Ctrl Pts',(5.77279253415804,31.8989686118257,11.3034179572156));
#10758=CARTESIAN_POINT('Ctrl Pts',(-0.340285255921168,32.1372208354108,
12.687655303583));
#10759=CARTESIAN_POINT('Ctrl Pts',(-6.37037719127529,32.3754730589959,10.9777359049497));
#10760=CARTESIAN_POINT('Ctrl Pts',(-10.846916079753,32.613725282581,6.59066026409488));
#10761=CARTESIAN_POINT('Ctrl Pts',(-12.6782019449145,32.8519775061661,0.596310826607595));
#10762=CARTESIAN_POINT('Ctrl Pts',(-11.4176364692439,33.0902297297512,-5.54346178971963));
#10763=CARTESIAN_POINT('Ctrl Pts',(-7.3726355681259,33.3284819533363,-10.3313424073348));
#10764=CARTESIAN_POINT('Ctrl Pts',(-1.52965942840387,33.5667341769214,-12.5997036945729));
#10765=CARTESIAN_POINT('Ctrl Pts',(4.68635695588896,33.8049864005065,-11.7953571221779));
#10766=CARTESIAN_POINT('Ctrl Pts',(9.75950472997414,34.0432386240916,-8.11445984550458));
#10767=CARTESIAN_POINT('Ctrl Pts',(12.4525880502679,34.2814908476767,-2.45467757688521));
#10768=CARTESIAN_POINT('Ctrl Pts',(12.1088408149773,34.5197430712618,3.80373044244303));
#10769=CARTESIAN_POINT('Ctrl Pts',(8.81209315581226,34.7579952948469,9.13451724870399));
#10770=CARTESIAN_POINT('Ctrl Pts',(3.3663276672789,34.996247518432,12.237656197023));
#10771=CARTESIAN_POINT('Ctrl Pts',(-2.90038899301814,35.2344997420171,12.3563803299066));
#10772=CARTESIAN_POINT('Ctrl Pts',(-8.45978361366359,35.4727519656022,9.46173622141396));
#10773=CARTESIAN_POINT('Ctrl Pts',(-11.9560786482159,35.7110041891873,4.25964489491223));
#10774=CARTESIAN_POINT('Ctrl Pts',(-12.5366275691515,35.9492564127724,-1.98125216037409));
#10775=CARTESIAN_POINT('Ctrl Pts',(-10.0598511352971,36.1875086363575,-7.7389783971189));
#10776=CARTESIAN_POINT('Ctrl Pts',(-5.12976425887965,36.4257608599426,-11.6093888526747));
#10777=CARTESIAN_POINT('Ctrl Pts',(1.05132544564253,36.6640130835277,-12.648600933315));
#10778=CARTESIAN_POINT('Ctrl Pts',(6.97602722060828,36.9022653071128,-10.6031805544441));
#10779=CARTESIAN_POINT('Ctrl Pts',(11.1994745652053,37.1405175306979,-5.97194720494374));
#10780=CARTESIAN_POINT('Ctrl Pts',(12.6916912259241,37.378769754283,0.115673336338169));
#10781=CARTESIAN_POINT('Ctrl Pts',(11.0887643176353,37.6170219778681,6.17508477858514));
#10782=CARTESIAN_POINT('Ctrl Pts',(6.78160968259758,37.8552742014532,10.7285687654699));
#10783=CARTESIAN_POINT('Ctrl Pts',(0.820603756208998,38.0935264250383,12.6656625634705));
#10784=CARTESIAN_POINT('Ctrl Pts',(-5.34050314292663,38.3317786486234,11.5139603988529));
#10785=CARTESIAN_POINT('Ctrl Pts',(-10.1992557008902,38.5700308722085,7.55433740992864));
#10786=CARTESIAN_POINT('Ctrl Pts',(-12.5706171211714,38.8082830957936,1.75241674191245));
#10787=CARTESIAN_POINT('Ctrl Pts',(-11.8765326492695,39.0465353193787,-4.47684713181242));
#10788=CARTESIAN_POINT('Ctrl Pts',(-8.28576249547599,39.2847875429638,-9.61437847979471));
#10789=CARTESIAN_POINT('Ctrl Pts',(-2.67501413356175,39.5230397665489,-12.4071504841623));
#10790=CARTESIAN_POINT('Ctrl Pts',(3.58949941361916,39.761291990134,-12.1743630678598));
#10791=CARTESIAN_POINT('Ctrl Pts',(7.17989388445823,39.9201268058574,-10.0393207828014));
#10792=CARTESIAN_POINT('Ctrl Pts',(8.61150142334309,39.9995442137191,-8.60695743600425));
#10793=CARTESIAN_POINT('',(-9.92496439632576,40.0002541663958,-3.43141021993915));
#10794=CARTESIAN_POINT('Ctrl Pts',(8.61094305413662,40.,-8.60639936142963));
#10795=CARTESIAN_POINT('Ctrl Pts',(8.39826176691632,40.,-8.79212327549388));
#10796=CARTESIAN_POINT('Ctrl Pts',(8.17937308111424,40.,-8.96994937667224));
#10797=CARTESIAN_POINT('Ctrl Pts',(7.95478109509821,40.,-9.13970638711401));
#10798=CARTESIAN_POINT('Ctrl Pts',(7.72804274042583,40.,-9.31108572225611));
#10799=CARTESIAN_POINT('Ctrl Pts',(7.49549100836207,40.,-9.4742413025714));
#10800=CARTESIAN_POINT('Ctrl Pts',(7.2576130834412,40.,-9.628954303971));
#10801=CARTESIAN_POINT('Ctrl Pts',(7.01927567556664,40.,-9.78396614767336));
#10802=CARTESIAN_POINT('Ctrl Pts',(6.77559089375214,40.,-9.93050302185609));
#10803=CARTESIAN_POINT('Ctrl Pts',(6.52702586473483,40.,-10.06829815855));
#10804=CARTESIAN_POINT('Ctrl Pts',(6.27982630250056,40.,-10.2053363316325));
#10805=CARTESIAN_POINT('Ctrl Pts',(6.02779937924827,40.,-10.3337287424236));
#10806=CARTESIAN_POINT('Ctrl Pts',(5.77139073271193,40.,-10.4531635932807));
#10807=CARTESIAN_POINT('Ctrl Pts',(5.51880872753046,40.,-10.5708159990226));
#10808=CARTESIAN_POINT('Ctrl Pts',(5.26197426321313,40.,-10.6797763194938));
#10809=CARTESIAN_POINT('Ctrl Pts',(5.00130823957099,40.,-10.7796963454939));
#10810=CARTESIAN_POINT('Ctrl Pts',(4.90713970256531,40.,-10.8157935803178));
#10811=CARTESIAN_POINT('Ctrl Pts',(4.81247110078974,40.,-10.8507104814013));
#10812=CARTESIAN_POINT('Ctrl Pts',(4.71732232047202,40.,-10.8844289444319));
#10813=CARTESIAN_POINT('Ctrl Pts',(4.68473084450778,40.,-10.8959785877772));
#10814=CARTESIAN_POINT('Ctrl Pts',(4.65208303079231,40.,-10.9073876128803));
#10815=CARTESIAN_POINT('Ctrl Pts',(4.61937968084376,40.,-10.9186552672316));
#10816=CARTESIAN_POINT('Ctrl Pts',(4.59185356383537,40.,-10.9281391510713));
#10817=CARTESIAN_POINT('Ctrl Pts',(4.56428866349076,40.,-10.9375226531726));
#10818=CARTESIAN_POINT('Ctrl Pts',(4.53669821841154,40.,-10.9468011456384));
#10819=CARTESIAN_POINT('Ctrl Pts',(4.27228656872567,40.,-11.0357211138538));
#10820=CARTESIAN_POINT('Ctrl Pts',(4.00522676966766,40.,-11.1151060432447));
#10821=CARTESIAN_POINT('Ctrl Pts',(3.73596790268647,40.,-11.1847326159485));
#10822=CARTESIAN_POINT('Ctrl Pts',(3.59988597511653,40.,-11.2199214969307));
#10823=CARTESIAN_POINT('Ctrl Pts',(3.46324208617,40.,-11.2526170856896));
#10824=CARTESIAN_POINT('Ctrl Pts',(3.3260929489447,40.,-11.2827856394737));
#10825=CARTESIAN_POINT('Ctrl Pts',(3.05396201990355,40.,-11.3426459983151));
#10826=CARTESIAN_POINT('Ctrl Pts',(2.77984200145982,40.,-11.3925606000749));
#10827=CARTESIAN_POINT('Ctrl Pts',(2.5042778621081,40.,-11.4325612835728));
#10828=CARTESIAN_POINT('Ctrl Pts',(2.22869992434682,40.,-11.4725639700375));
#10829=CARTESIAN_POINT('Ctrl Pts',(1.95167706598645,40.,-11.5026516740376));
#10830=CARTESIAN_POINT('Ctrl Pts',(1.67375680737823,40.,-11.5228042109087));
#10831=CARTESIAN_POINT('Ctrl Pts',(1.398642054319,40.,-11.5427533151323));
#10832=CARTESIAN_POINT('Ctrl Pts',(1.12264732111162,40.,-11.5529666784398));
#10833=CARTESIAN_POINT('Ctrl Pts',(0.846315503642963,40.,-11.5533754837982));
#10834=CARTESIAN_POINT('Ctrl Pts',(0.643529263690987,40.,-11.5536754858113));
#10835=CARTESIAN_POINT('Ctrl Pts',(0.440561695111733,40.,-11.5486943579065));
#10836=CARTESIAN_POINT('Ctrl Pts',(0.237634295057578,40.,-11.5383883933861));
#10837=CARTESIAN_POINT('Ctrl Pts',(0.200021572236072,40.,-11.5364781762995));
#10838=CARTESIAN_POINT('Ctrl Pts',(0.162410249405167,40.,-11.5343849868962));
#10839=CARTESIAN_POINT('Ctrl Pts',(0.124801765584846,40.,-11.5321084946763));
#10840=CARTESIAN_POINT('Ctrl Pts',(0.0953789719671696,40.,-11.5303274933182));
#10841=CARTESIAN_POINT('Ctrl Pts',(0.0659671184443719,40.,-11.5284348486951));
#10842=CARTESIAN_POINT('Ctrl Pts',(0.0365696537066474,40.,-11.5264308156415));
#10843=CARTESIAN_POINT('Ctrl Pts',(-0.236604483961971,40.,-11.5078084614291));
#10844=CARTESIAN_POINT('Ctrl Pts',(-0.508615486317793,40.,-11.4795673079924));
#10845=CARTESIAN_POINT('Ctrl Pts',(-0.778950107545348,40.,-11.4417467199426));
#10846=CARTESIAN_POINT('Ctrl Pts',(-1.05191932377349,40.,-11.4035575445037));
#10847=CARTESIAN_POINT('Ctrl Pts',(-1.32317999343784,40.,-11.355601299064));
#10848=CARTESIAN_POINT('Ctrl Pts',(-1.5921940890953,40.,-11.2978654190554));
#10849=CARTESIAN_POINT('Ctrl Pts',(-1.86120818475262,40.,-11.2401295390468));
#10850=CARTESIAN_POINT('Ctrl Pts',(-2.12797635797297,40.,-11.1726139378876));
#10851=CARTESIAN_POINT('Ctrl Pts',(-2.39194108188819,40.,-11.0952540671311));
#10852=CARTESIAN_POINT('Ctrl Pts',(-2.65358663251955,40.,-11.018573874109));
#10853=CARTESIAN_POINT('Ctrl Pts',(-2.91247824429409,40.,-10.9322209570423));
#10854=CARTESIAN_POINT('Ctrl Pts',(-3.16812267150498,40.,-10.8364284814825));
#10855=CARTESIAN_POINT('Ctrl Pts',(-3.42177931939053,40.,-10.7413808463422));
#10856=CARTESIAN_POINT('Ctrl Pts',(-3.67223957309176,40.,-10.6370394684347));
#10857=CARTESIAN_POINT('Ctrl Pts',(-3.91898715115294,40.,-10.5235942862973));
#10858=CARTESIAN_POINT('Ctrl Pts',(-3.96835687438594,40.,-10.5008959591719));
#10859=CARTESIAN_POINT('Ctrl Pts',(-4.01757784425976,40.,-10.4778330708281));
#10860=CARTESIAN_POINT('Ctrl Pts',(-4.06664573143816,40.,-10.4544069809796));
#10861=CARTESIAN_POINT('Ctrl Pts',(-4.10490890648528,40.,-10.43613929863));
#10862=CARTESIAN_POINT('Ctrl Pts',(-4.14308479220665,40.,-10.4176478398036));
#10863=CARTESIAN_POINT('Ctrl Pts',(-4.18113965154256,40.,-10.3989489818942));
#10864=CARTESIAN_POINT('Ctrl Pts',(-4.42108222934683,40.,-10.28104939569));
#10865=CARTESIAN_POINT('Ctrl Pts',(-4.65640472965588,40.,-10.154821243158));
#10866=CARTESIAN_POINT('Ctrl Pts',(-4.88668744403159,40.,-10.0205608401689));
#10867=CARTESIAN_POINT('Ctrl Pts',(-5.11739045524781,40.,-9.88605539393666));
#10868=CARTESIAN_POINT('Ctrl Pts',(-5.34303579544783,40.,-9.74348797347264));
#10869=CARTESIAN_POINT('Ctrl Pts',(-5.56317346295674,40.,-9.59311273009281));
#10870=CARTESIAN_POINT('Ctrl Pts',(-5.78203974193378,40.,-9.4436059676144));
#10871=CARTESIAN_POINT('Ctrl Pts',(-5.99546225346409,40.,-9.28638090254399));
#10872=CARTESIAN_POINT('Ctrl Pts',(-6.2029636998557,40.,-9.12164999441353));
#10873=CARTESIAN_POINT('Ctrl Pts',(-6.40709362068619,40.,-8.95959566746902));
#10874=CARTESIAN_POINT('Ctrl Pts',(-6.6054936866607,40.,-8.79027700894159));
#10875=CARTESIAN_POINT('Ctrl Pts',(-6.79766944482237,40.,-8.61386626430386));
#10876=CARTESIAN_POINT('Ctrl Pts',(-6.91421310725171,40.,-8.50688318553972));
#10877=CARTESIAN_POINT('Ctrl Pts',(-7.02846683556768,40.,-8.39729127275609));
#10878=CARTESIAN_POINT('Ctrl Pts',(-7.1403121407595,40.,-8.28512438529733));
#10879=CARTESIAN_POINT('Ctrl Pts',(-7.2322458360855,40.,-8.19292635839208));
#10880=CARTESIAN_POINT('Ctrl Pts',(-7.32255217347813,40.,-8.09898847748874));
#10881=CARTESIAN_POINT('Ctrl Pts',(-7.41118873118237,40.,-8.00335941612173));
#10882=CARTESIAN_POINT('Ctrl Pts',(-7.44595173802253,40.,-7.96585396915354));
#10883=CARTESIAN_POINT('Ctrl Pts',(-7.48045783348702,40.,-7.92808841917705));
#10884=CARTESIAN_POINT('Ctrl Pts',(-7.51470444838488,40.,-7.89006554590154));
#10885=CARTESIAN_POINT('Ctrl Pts',(-7.54132180621626,40.,-7.86051318206149));
#10886=CARTESIAN_POINT('Ctrl Pts',(-7.56778132931981,40.,-7.83080646494714));
#10887=CARTESIAN_POINT('Ctrl Pts',(-7.59406823367193,40.,-7.8009624951305));
#10888=CARTESIAN_POINT('Ctrl Pts',(-7.76810920210893,40.,-7.60337082213176));
#10889=CARTESIAN_POINT('Ctrl Pts',(-7.93474819741371,40.,-7.39958702375726));
#10890=CARTESIAN_POINT('Ctrl Pts',(-8.09372374437956,40.,-7.19007656351675));
#10891=CARTESIAN_POINT('Ctrl Pts',(-8.25269853624522,40.,-6.98056709840658));
#10892=CARTESIAN_POINT('Ctrl Pts',(-8.40401024026009,40.,-6.76533042182595));
#10893=CARTESIAN_POINT('Ctrl Pts',(-8.54735114309888,40.,-6.5448081825227));
#10894=CARTESIAN_POINT('Ctrl Pts',(-8.68948029878482,40.,-6.32615015078565));
#10895=CARTESIAN_POINT('Ctrl Pts',(-8.82377305934234,40.,-6.10229494668581));
#10896=CARTESIAN_POINT('Ctrl Pts',(-8.94988036808553,40.,-5.87365868822008));
#10897=CARTESIAN_POINT('Ctrl Pts',(-8.9666093409471,40.,-5.84332856856911));
#10898=CARTESIAN_POINT('Ctrl Pts',(-8.98319419398911,40.,-5.81291429953107));
#10899=CARTESIAN_POINT('Ctrl Pts',(-8.9996340436321,40.,-5.78241684186142));
#10900=CARTESIAN_POINT('Ctrl Pts',(-9.02204332078306,40.,-5.74084553822058));
#10901=CARTESIAN_POINT('Ctrl Pts',(-9.04417775820945,40.,-5.69912961527342));
#10902=CARTESIAN_POINT('Ctrl Pts',(-9.06603067483243,40.,-5.65728118478675));
#10903=CARTESIAN_POINT('Ctrl Pts',(-9.18590518867724,40.,-5.42772096880703));
#10904=CARTESIAN_POINT('Ctrl Pts',(-9.2973605568515,40.,-5.1940857613916));
#10905=CARTESIAN_POINT('Ctrl Pts',(-9.40010767792124,40.,-4.95680439652004));
#10906=CARTESIAN_POINT('Ctrl Pts',(-9.50150771815981,40.,-4.7226339429313));
#10907=CARTESIAN_POINT('Ctrl Pts',(-9.59442650170164,40.,-4.48491173585104));
#10908=CARTESIAN_POINT('Ctrl Pts',(-9.67853712541855,40.,-4.24403874401865));
#10909=CARTESIAN_POINT('Ctrl Pts',(-9.73985884517572,40.,-4.06842779917617));
#10910=CARTESIAN_POINT('Ctrl Pts',(-9.79649777669627,40.,-3.89114186081739));
#10911=CARTESIAN_POINT('Ctrl Pts',(-9.84830976294177,40.,-3.71233506504282));
#10912=CARTESIAN_POINT('Ctrl Pts',(-9.87531187063298,40.,-3.6191488989586));
#10913=CARTESIAN_POINT('Ctrl Pts',(-9.90100270302723,40.,-3.52554965431835));
#10914=CARTESIAN_POINT('Ctrl Pts',(-9.92537747903998,40.,-3.43156570488038));
#10915=CARTESIAN_POINT('Ctrl Pts',(-9.9245821948243,40.0002541663958,-3.43127807940082));
#10916=CARTESIAN_POINT('Ctrl Pts',(-9.92574247154754,40.0001694442638,-3.42792211073779));
#10917=CARTESIAN_POINT('Ctrl Pts',(-9.92690104605405,40.0000847221319,-3.42456555355841));
#10918=CARTESIAN_POINT('Ctrl Pts',(-9.92805791774767,39.9999999999999,-3.42120840958977));
#10919=CARTESIAN_POINT('Ctrl Pts',(7.93381306740072,20.,-6.87936125025729));
#10920=CARTESIAN_POINT('Ctrl Pts',(8.11334533077575,20.,-6.70251189458677));
#10921=CARTESIAN_POINT('Ctrl Pts',(8.28605380477994,20.,-6.51937440106475));
#10922=CARTESIAN_POINT('Ctrl Pts',(8.45179833248054,20.,-6.33047258793705));
#10923=CARTESIAN_POINT('Ctrl Pts',(8.62014953567792,20.,-6.13859990310451));
#10924=CARTESIAN_POINT('Ctrl Pts',(8.78131641961311,20.,-5.94077982210926));
#10925=CARTESIAN_POINT('Ctrl Pts',(8.9351278146894,20.,-5.73751337470593));
#10926=CARTESIAN_POINT('Ctrl Pts',(9.0913599031574,20.,-5.53104790719269));
#10927=CARTESIAN_POINT('Ctrl Pts',(9.24000360361905,20.,-5.31896290747305));
#10928=CARTESIAN_POINT('Ctrl Pts',(9.38084825717968,20.,-5.10173994365898));
#10929=CARTESIAN_POINT('Ctrl Pts',(9.52214874513409,20.,-4.88381395210817));
#10930=CARTESIAN_POINT('Ctrl Pts',(9.65560002896776,20.,-4.66071618702915));
#10931=CARTESIAN_POINT('Ctrl Pts',(9.78095181325634,20.,-4.43289630140568));
#10932=CARTESIAN_POINT('Ctrl Pts',(9.90574239039269,20.,-4.20609637852114));
#10933=CARTESIAN_POINT('Ctrl Pts',(10.0225061927535,20.,-3.97461598352399));
#10934=CARTESIAN_POINT('Ctrl Pts',(10.1309533974595,20.,-3.73887036917977));
#10935=CARTESIAN_POINT('Ctrl Pts',(10.1620449658876,20.,-3.67128263448554));
#10936=CARTESIAN_POINT('Ctrl Pts',(10.192452657003,20.,-3.6033441665067));
#10937=CARTESIAN_POINT('Ctrl Pts',(10.22216892119,20.,-3.53506441406799));
#10938=CARTESIAN_POINT('Ctrl Pts',(10.239684090736,20.,-3.49481940100045));
#10939=CARTESIAN_POINT('Ctrl Pts',(10.2569611674518,20.,-3.45445054561043));
#10940=CARTESIAN_POINT('Ctrl Pts',(10.2739835311413,20.,-3.41399615802963));
#10941=CARTESIAN_POINT('Ctrl Pts',(10.3769729884857,20.,-3.16923723382034));
#10942=CARTESIAN_POINT('Ctrl Pts',(10.4707505425509,20.,-2.92110624344397));
#10943=CARTESIAN_POINT('Ctrl Pts',(10.5551246852778,20.,-2.67011766558322));
#10944=CARTESIAN_POINT('Ctrl Pts',(10.5927935636692,20.,-2.55806368895609));
#10945=CARTESIAN_POINT('Ctrl Pts',(10.628587702233,20.,-2.44543962428696));
#10946=CARTESIAN_POINT('Ctrl Pts',(10.6624876486376,20.,-2.33228893760792));
#10947=CARTESIAN_POINT('Ctrl Pts',(10.7376977925035,20.,-2.08125374946669));
#10948=CARTESIAN_POINT('Ctrl Pts',(10.8035876329606,20.,-1.82762824132245));
#10949=CARTESIAN_POINT('Ctrl Pts',(10.8602429504416,20.,-1.57194508022933));
#10950=CARTESIAN_POINT('Ctrl Pts',(10.9173812906677,20.,-1.31408205698315));
#10951=CARTESIAN_POINT('Ctrl Pts',(10.9651271233675,20.,-1.05412557318626));
#10952=CARTESIAN_POINT('Ctrl Pts',(11.0035202228593,20.,-0.792598803439725));
#10953=CARTESIAN_POINT('Ctrl Pts',(11.04208073776,20.,-0.529931630555835));
#10954=CARTESIAN_POINT('Ctrl Pts',(11.0712069012117,20.,-0.265679827708335));
#10955=CARTESIAN_POINT('Ctrl Pts',(11.0908885652408,20.,-0.000359128635273066));
#10956=CARTESIAN_POINT('Ctrl Pts',(11.1054206053252,20.,0.195541534461971));
#10957=CARTESIAN_POINT('Ctrl Pts',(11.1148027799559,19.9999999999999,0.392025269686389));
#10958=CARTESIAN_POINT('Ctrl Pts',(11.1190128627105,20.,0.588886412300436));
#10959=CARTESIAN_POINT('Ctrl Pts',(11.1196345841872,20.,0.617957764914658));
#10960=CARTESIAN_POINT('Ctrl Pts',(11.1201435132142,20.,0.647039404376552));
#10961=CARTESIAN_POINT('Ctrl Pts',(11.1205394628636,20.,0.676124093961359));
#10962=CARTESIAN_POINT('Ctrl Pts',(11.1242136969702,20.,0.946016891253714));
#10963=CARTESIAN_POINT('Ctrl Pts',(11.1181568313559,20.,1.21559421576547));
#10964=CARTESIAN_POINT('Ctrl Pts',(11.1024699155507,20.,1.4843035710275));
#10965=CARTESIAN_POINT('Ctrl Pts',(11.0859047811347,20.,1.76805639051346));
#10966=CARTESIAN_POINT('Ctrl Pts',(11.0586017438614,20.,2.05084190407223));
#10967=CARTESIAN_POINT('Ctrl Pts',(11.0206211947832,20.,2.33203086493943));
#10968=CARTESIAN_POINT('Ctrl Pts',(10.9826406457049,20.,2.61321982580663));
#10969=CARTESIAN_POINT('Ctrl Pts',(10.9339826723985,20.,2.89281305830034));
#10970=CARTESIAN_POINT('Ctrl Pts',(10.87464624646,20.,3.17019109503699));
#10971=CARTESIAN_POINT('Ctrl Pts',(10.8153870220998,20.,3.4472082400973));
#10972=CARTESIAN_POINT('Ctrl Pts',(10.7454772306754,20.,3.72201679033749));
#10973=CARTESIAN_POINT('Ctrl Pts',(10.6652311260161,20.,3.99411127683229));
#10974=CARTESIAN_POINT('Ctrl Pts',(10.5849850213568,20.,4.26620576332708));
#10975=CARTESIAN_POINT('Ctrl Pts',(10.4944023351477,20.,4.53558691968042));
#10976=CARTESIAN_POINT('Ctrl Pts',(10.3937362784269,20.,4.80173496530221));
#10977=CARTESIAN_POINT('Ctrl Pts',(10.3777423329852,20.,4.84402089026791));
#10978=CARTESIAN_POINT('Ctrl Pts',(10.3614937302683,20.,4.88622515835007));
#10979=CARTESIAN_POINT('Ctrl Pts',(10.3449913509334,20.,4.92834563232135));
#10980=CARTESIAN_POINT('Ctrl Pts',(10.3343844651706,20.,4.95541851960774));
#10981=CARTESIAN_POINT('Ctrl Pts',(10.3236726703155,20.,4.98245685781199));
#10982=CARTESIAN_POINT('Ctrl Pts',(10.3128617315938,20.,5.00944653944195));
#10983=CARTESIAN_POINT('Ctrl Pts',(10.2113685957594,20.,5.26282577822009));
#10984=CARTESIAN_POINT('Ctrl Pts',(10.1010260091921,20.,5.51221436662185));
#10985=CARTESIAN_POINT('Ctrl Pts',(9.98219337299342,20.,5.75718786449119));
#10986=CARTESIAN_POINT('Ctrl Pts',(9.86134406368381,20.,6.00631873429003));
#10987=CARTESIAN_POINT('Ctrl Pts',(9.73171400193977,20.,6.25088396566522));
#10988=CARTESIAN_POINT('Ctrl Pts',(9.59362742884161,20.,6.49043373047328));
#10989=CARTESIAN_POINT('Ctrl Pts',(9.45505341266511,20.,6.73082910157132));
#10990=CARTESIAN_POINT('Ctrl Pts',(9.30796286005019,20.,6.9661741367737));
#10991=CARTESIAN_POINT('Ctrl Pts',(9.15263229120085,20.,7.19600189655872));
#10992=CARTESIAN_POINT('Ctrl Pts',(8.99804398992683,20.,7.42473139413262));
#10993=CARTESIAN_POINT('Ctrl Pts',(8.83529395846679,20.,7.64799680126327));
#10994=CARTESIAN_POINT('Ctrl Pts',(8.66460799086994,20.,7.86531682614724));
#10995=CARTESIAN_POINT('Ctrl Pts',(8.55444285882568,20.,8.00558078325092));
#10996=CARTESIAN_POINT('Ctrl Pts',(8.44097088268035,20.,8.14336759877014));
#10997=CARTESIAN_POINT('Ctrl Pts',(8.32424315342715,20.,8.27854145188553));
#10998=CARTESIAN_POINT('Ctrl Pts',(8.23663382474174,20.,8.37999541319385));
#10999=CARTESIAN_POINT('Ctrl Pts',(8.14719031008403,20.,8.47997733921384));
#11000=CARTESIAN_POINT('Ctrl Pts',(8.05595931410645,20.,8.57845490970599));
#11001=CARTESIAN_POINT('Ctrl Pts',(8.01761638595146,20.,8.61984345720345));
#11002=CARTESIAN_POINT('Ctrl Pts',(7.97895769437451,20.,8.66096625350117));
#11003=CARTESIAN_POINT('Ctrl Pts',(7.93998660061812,20.,8.70182079230146));
#11004=CARTESIAN_POINT('Ctrl Pts',(7.91066081913535,20.,8.73256386779547));
#11005=CARTESIAN_POINT('Ctrl Pts',(7.88115851935513,20.,8.76315450964986));
#11006=CARTESIAN_POINT('Ctrl Pts',(7.85149823336609,20.,8.79357447451951));
#11007=CARTESIAN_POINT('Ctrl Pts',(7.65681753608095,20.,8.99324146270702));
#11008=CARTESIAN_POINT('Ctrl Pts',(7.45515097010471,20.,9.18575086315305));
#11009=CARTESIAN_POINT('Ctrl Pts',(7.24701145539745,20.,9.37088205580245));
#11010=CARTESIAN_POINT('Ctrl Pts',(7.03612872419095,20.,9.5584532221537));
#11011=CARTESIAN_POINT('Ctrl Pts',(6.81860092022066,20.,9.73845086260295));
#11012=CARTESIAN_POINT('Ctrl Pts',(6.59491638245657,20.,9.910616184975));
#11013=CARTESIAN_POINT('Ctrl Pts',(6.37323524877219,20.,10.0812395290205));
#11014=CARTESIAN_POINT('Ctrl Pts',(6.14550664682392,20.,10.2441705629266));
#11015=CARTESIAN_POINT('Ctrl Pts',(5.91216887742395,20.,10.399123041683));
#11016=CARTESIAN_POINT('Ctrl Pts',(5.86175766100923,20.,10.4325995892675));
#11017=CARTESIAN_POINT('Ctrl Pts',(5.81108451494134,20.,10.4657035986193));
#11018=CARTESIAN_POINT('Ctrl Pts',(5.76015366565449,20.,10.4984319462714));
#11019=CARTESIAN_POINT('Ctrl Pts',(5.72101534194005,20.,10.5235823744104));
#11020=CARTESIAN_POINT('Ctrl Pts',(5.6817272115307,20.,10.548509349187));
#11021=CARTESIAN_POINT('Ctrl Pts',(5.64230701889093,20.,10.5732018577602));
#11022=CARTESIAN_POINT('Ctrl Pts',(5.39975652942212,20.,10.7251336378856));
#11023=CARTESIAN_POINT('Ctrl Pts',(5.1520474982564,20.,10.8682962685956));
#11024=CARTESIAN_POINT('Ctrl Pts',(4.89968271153781,20.,11.0024328305905));
#11025=CARTESIAN_POINT('Ctrl Pts',(4.64696653025092,20.,11.1367561653119));
#11026=CARTESIAN_POINT('Ctrl Pts',(4.38958112307547,20.,11.2620286878548));
#11027=CARTESIAN_POINT('Ctrl Pts',(4.12799552824453,20.,11.3779546569627));
#11028=CARTESIAN_POINT('Ctrl Pts',(3.90990991980607,20.,11.474602889917));
#11029=CARTESIAN_POINT('Ctrl Pts',(3.6889041237799,20.,11.5647540978177));
#11030=CARTESIAN_POINT('Ctrl Pts',(3.46523470555786,20.,11.6482137561969));
#11031=CARTESIAN_POINT('Ctrl Pts',(3.36017632166553,20.,11.6874150779477));
#11032=CARTESIAN_POINT('Ctrl Pts',(3.25453010754725,20.,11.7251397777184));
#11033=CARTESIAN_POINT('Ctrl Pts',(3.14832787575819,20.,11.7613864006883));
#11034=CARTESIAN_POINT('Ctrl Pts',(-3.14809266229074,20.0004548598273,11.7612561652465));
#11035=CARTESIAN_POINT('Ctrl Pts',(-5.10435921967941,20.079872267689,11.2376294107338));
#11036=CARTESIAN_POINT('Ctrl Pts',(-8.74855648214142,20.2387070834124,9.19577637638592));
#11037=CARTESIAN_POINT('Ctrl Pts',(-12.0824131583271,20.4769593069975,3.88694525557923));
#11038=CARTESIAN_POINT('Ctrl Pts',(-12.4691756011198,20.7152115305826,-2.36849165908917));
#11039=CARTESIAN_POINT('Ctrl Pts',(-9.81532842158459,20.9534637541677,-8.04695416362741));
#11040=CARTESIAN_POINT('Ctrl Pts',(-4.76767052948596,21.1917159777528,-11.7626807483446));
#11041=CARTESIAN_POINT('Ctrl Pts',(1.44262007163241,21.4299682013379,-12.6099815538241));
#11042=CARTESIAN_POINT('Ctrl Pts',(7.30112969128478,21.668220424923,-10.3819902917566));
#11043=CARTESIAN_POINT('Ctrl Pts',(11.3790859526647,21.9064726485081,-5.62216684002108));
#11044=CARTESIAN_POINT('Ctrl Pts',(12.6820163068472,22.1447248720932,0.508761805007711));
#11045=CARTESIAN_POINT('Ctrl Pts',(10.8921610480429,22.3829770956783,6.51560837433268));
#11046=CARTESIAN_POINT('Ctrl Pts',(6.44602083161166,22.6212293192634,10.9334889418598));
#11047=CARTESIAN_POINT('Ctrl Pts',(0.427879238319787,22.8594815428485,12.6850014557692));
#11048=CARTESIAN_POINT('Ctrl Pts',(-5.69460937880687,23.0977337664336,11.343005608659));
#11049=CARTESIAN_POINT('Ctrl Pts',(-10.4283456669994,23.3359859900187,7.23477408056129));
#11050=CARTESIAN_POINT('Ctrl Pts',(-12.6189061760199,23.5742382136038,1.36218808736743));
#11051=CARTESIAN_POINT('Ctrl Pts',(-11.7320759505821,23.8124904371889,-4.8425968202088));
#11052=CARTESIAN_POINT('Ctrl Pts',(-7.9841274603316,24.050742660774,-9.86641060411259));
#11053=CARTESIAN_POINT('Ctrl Pts',(-2.28907833971999,24.2889948843591,-12.4840886814594));
#11054=CARTESIAN_POINT('Ctrl Pts',(3.96421161517394,24.5272471079442,-12.0572540805866));
#11055=CARTESIAN_POINT('Ctrl Pts',(9.25074357873224,24.7654993315293,-8.68999959656226));
#11056=CARTESIAN_POINT('Ctrl Pts',(12.2812834041494,25.0037515551144,-3.20350240934556));
#11057=CARTESIAN_POINT('Ctrl Pts',(12.3167689831387,25.2420037786995,3.06423751515814));
#11058=CARTESIAN_POINT('Ctrl Pts',(9.34854639793627,25.4802560022846,8.58469743127442));
#11059=CARTESIAN_POINT('Ctrl Pts',(4.10048035829082,25.7185082258697,12.0115948386183));
#11060=CARTESIAN_POINT('Ctrl Pts',(-2.14757572311472,25.9567604494548,12.5092073390711));
#11061=CARTESIAN_POINT('Ctrl Pts',(-7.87189942455396,26.1950126730399,9.95618145611697));
#11062=CARTESIAN_POINT('Ctrl Pts',(-11.6764916927204,26.433264896625,4.97512728354432));
#11063=CARTESIAN_POINT('Ctrl Pts',(-12.6335211398357,26.6715171202101,-1.21921833443057));
#11064=CARTESIAN_POINT('Ctrl Pts',(-10.5095956183063,26.9097693437952,-7.11623142381309));
#11065=CARTESIAN_POINT('Ctrl Pts',(-5.82267989949552,27.1480215673803,-11.2777989220269));
#11066=CARTESIAN_POINT('Ctrl Pts',(0.284221140002502,27.3862737909654,-12.6890333785201));
#11067=CARTESIAN_POINT('Ctrl Pts',(6.32180876134884,27.6245260145505,-11.0057750168977));
#11068=CARTESIAN_POINT('Ctrl Pts',(10.8176877886728,27.8627782381356,-6.63852247449934));
#11069=CARTESIAN_POINT('Ctrl Pts',(12.6754417380569,28.1010304617207,-0.652323909386644));
#11070=CARTESIAN_POINT('Ctrl Pts',(11.4420174822295,28.3392826853058,5.49295782561536));
#11071=CARTESIAN_POINT('Ctrl Pts',(7.41821196824626,28.5775349088909,10.2986640362622));
#11072=CARTESIAN_POINT('Ctrl Pts',(1.58531643343681,28.815787132476,12.592820237878));
#11073=CARTESIAN_POINT('Ctrl Pts',(-4.63419249983834,29.0540393560611,11.8159472583486));
#11074=CARTESIAN_POINT('Ctrl Pts',(-9.72355424374603,29.2922915796462,8.15750222841293));
#11075=CARTESIAN_POINT('Ctrl Pts',(-12.4416188307888,29.5305438032313,2.50967539873089));
#11076=CARTESIAN_POINT('Ctrl Pts',(-12.125527941276,29.7687960268164,-3.75018957960365));
#11077=CARTESIAN_POINT('Ctrl Pts',(-8.85236711500348,30.0070482504015,-9.0954904320129));
#11078=CARTESIAN_POINT('Ctrl Pts',(-3.42036678980662,30.2453004739866,-12.2226609525431));
#11079=CARTESIAN_POINT('Ctrl Pts',(2.8457633032496,30.4835526975717,-12.3690735691688));
#11080=CARTESIAN_POINT('Ctrl Pts',(8.41789300705035,30.7218049211568,-9.49902242651769));
#11081=CARTESIAN_POINT('Ctrl Pts',(11.9371390374505,30.9600571447419,-4.31243102416829));
#11082=CARTESIAN_POINT('Ctrl Pts',(12.5452578039889,31.198309368327,1.92583913375176));
#11083=CARTESIAN_POINT('Ctrl Pts',(10.0939465085343,31.4365615919121,7.69445213257467));
#11084=CARTESIAN_POINT('Ctrl Pts',(5.18100996193967,31.6748138154972,11.5866080244356));
#11085=CARTESIAN_POINT('Ctrl Pts',(-0.995426934883139,31.9130660390823,
12.6531211546773));
#11086=CARTESIAN_POINT('Ctrl Pts',(-6.92910763357261,32.1513182626674,10.6338994324754));
#11087=CARTESIAN_POINT('Ctrl Pts',(-11.1729768889136,32.3895704862526,6.02137336306566));
#11088=CARTESIAN_POINT('Ctrl Pts',(-12.692076202498,32.6278227098376,-0.0595936877313756));
#11089=CARTESIAN_POINT('Ctrl Pts',(-11.1159406401054,32.8660749334227,-6.12602754019977));
#11090=CARTESIAN_POINT('Ctrl Pts',(-6.82894464797713,33.1043271570078,-10.6984982465997));
#11091=CARTESIAN_POINT('Ctrl Pts',(-0.876564103841478,33.3425793805929,
-12.6619108000923));
#11092=CARTESIAN_POINT('Ctrl Pts',(5.28958538888388,33.580831604178,-11.5374449576727));
#11093=CARTESIAN_POINT('Ctrl Pts',(10.1657560858716,33.8190838277631,-7.5993258214283));
#11094=CARTESIAN_POINT('Ctrl Pts',(12.5627892268212,34.0573360513483,-1.80794816851931));
#11095=CARTESIAN_POINT('Ctrl Pts',(11.8961168924868,34.2955882749333,4.42433640425057));
#11096=CARTESIAN_POINT('Ctrl Pts',(8.32832142376291,34.5338404985185,9.57765169549019));
#11097=CARTESIAN_POINT('Ctrl Pts',(2.72948623249549,34.7720927221035,12.395251294106));
#11098=CARTESIAN_POINT('Ctrl Pts',(-3.53499269162053,35.0103449456886,12.1900031340674));
#11099=CARTESIAN_POINT('Ctrl Pts',(-8.9373878642459,35.2485971692737,9.01196137918274));
#11100=CARTESIAN_POINT('Ctrl Pts',(-12.1602094057867,35.4868493928589,3.63615964285339));
#11101=CARTESIAN_POINT('Ctrl Pts',(-12.4175031914886,35.7251016164439,-2.62639757513609));
#11102=CARTESIAN_POINT('Ctrl Pts',(-9.6465226171822,35.9633538400291,-8.24845143865874));
#11103=CARTESIAN_POINT('Ctrl Pts',(-4.52303069773245,36.2016060636141,-11.858943589337));
#11104=CARTESIAN_POINT('Ctrl Pts',(1.70349921887366,36.4398582871992,-12.5773781093279));
#11105=CARTESIAN_POINT('Ctrl Pts',(7.51459433853916,36.6781105107843,-10.2285493487157));
#11106=CARTESIAN_POINT('Ctrl Pts',(11.4930945153334,36.9163627343694,-5.38526953581525));
#11107=CARTESIAN_POINT('Ctrl Pts',(12.6687572341596,37.1546149579545,0.771323677356681));
#11108=CARTESIAN_POINT('Ctrl Pts',(10.7548718477098,37.3928671815396,6.73981312826219));
#11109=CARTESIAN_POINT('Ctrl Pts',(6.2181805169326,37.6311194051247,11.0646545543017));
#11110=CARTESIAN_POINT('Ctrl Pts',(0.165052320677689,37.8693716287098,12.6911429724317));
#11111=CARTESIAN_POINT('Ctrl Pts',(-5.92832693959693,38.107623852295,11.2226236804367));
#11112=CARTESIAN_POINT('Ctrl Pts',(-10.5759575529497,38.34587607588,7.01722786017004));
#11113=CARTESIAN_POINT('Ctrl Pts',(-12.644412242237,38.5841282994652,1.10052888764604));
#11114=CARTESIAN_POINT('Ctrl Pts',(-11.6292598420606,38.8223805230502,-5.08455422895767));
#11115=CARTESIAN_POINT('Ctrl Pts',(-7.77805527350331,39.0606327466353,-10.0296666573467));
#11116=CARTESIAN_POINT('Ctrl Pts',(-2.03002093474416,39.2988849702204,-12.528816073021));
#11117=CARTESIAN_POINT('Ctrl Pts',(4.21310916249937,39.5371371938055,-11.972572766274));
#11118=CARTESIAN_POINT('Ctrl Pts',(9.42871875276412,39.7753894173906,-8.49650536082229));
#11119=CARTESIAN_POINT('Ctrl Pts',(12.3450606821512,40.0136416409757,-2.94849454622041));
#11120=CARTESIAN_POINT('Ctrl Pts',(12.2505387102373,40.2518938645608,3.31879409118882));
#11121=CARTESIAN_POINT('Ctrl Pts',(9.16897630005181,40.4901460881459,8.77627054946899));
#11122=CARTESIAN_POINT('Ctrl Pts',(3.84984706557643,40.7284188590102,12.0946935166284));
#11123=CARTESIAN_POINT('Ctrl Pts',(-0.32088071557368,40.8872742220127,12.3384797159896));
#11124=CARTESIAN_POINT('Ctrl Pts',(-2.30975236282056,40.9667121771535,11.9541908119849));
#11125=CARTESIAN_POINT('Ctrl Pts',(-3.00369270810988,19.6780228441179,11.2217787630359));
#11126=CARTESIAN_POINT('Ctrl Pts',(-4.87022721769824,19.7574402519795,10.7221702594042));
#11127=CARTESIAN_POINT('Ctrl Pts',(-8.34726868959891,19.916275067703,8.77397504146546));
#11128=CARTESIAN_POINT('Ctrl Pts',(-11.5282045966303,20.154527291288,3.70865485023876));
#11129=CARTESIAN_POINT('Ctrl Pts',(-11.8972266216495,20.3927795148732,-2.25985124607116));
#11130=CARTESIAN_POINT('Ctrl Pts',(-9.36510883582578,20.6310317384582,-7.67784818830401));
#11131=CARTESIAN_POINT('Ctrl Pts',(-4.54898211085908,20.8692839620433,-11.2231380018903));
#11132=CARTESIAN_POINT('Ctrl Pts',(1.3764484894743,21.1075361856285,-12.031573942001));
#11133=CARTESIAN_POINT('Ctrl Pts',(6.96623396044474,21.3457884092135,-9.90577847614093));
#11134=CARTESIAN_POINT('Ctrl Pts',(10.8571383270859,21.5840406327987,-5.364283505194));
#11135=CARTESIAN_POINT('Ctrl Pts',(12.1003045308358,21.8222928563837,0.485425394929287));
#11136=CARTESIAN_POINT('Ctrl Pts',(10.3925481951215,22.0605450799689,6.21674374369965));
#11137=CARTESIAN_POINT('Ctrl Pts',(6.15034811400611,22.2987973035539,10.431980418571));
#11138=CARTESIAN_POINT('Ctrl Pts',(0.408252833052742,22.5370495271391,12.1031527538748));
#11139=CARTESIAN_POINT('Ctrl Pts',(-5.43340317505451,22.7753017507242,10.8227129534321));
#11140=CARTESIAN_POINT('Ctrl Pts',(-9.95000757532424,23.0135539743092,6.90292201716564));
#11141=CARTESIAN_POINT('Ctrl Pts',(-12.0400892004408,23.2518061978944,1.2997058422424));
#11142=CARTESIAN_POINT('Ctrl Pts',(-11.1939370164893,23.4900584214795,-4.62047160536659));
#11143=CARTESIAN_POINT('Ctrl Pts',(-7.61790328489481,23.7283106450646,-9.41384792823294));
#11144=CARTESIAN_POINT('Ctrl Pts',(-2.18408053856523,23.9665628686497,-11.911455653472));
#11145=CARTESIAN_POINT('Ctrl Pts',(3.78237707693078,24.2048150922347,-11.5041995413608));
#11146=CARTESIAN_POINT('Ctrl Pts',(8.82642095160353,24.4430673158199,-8.29139775151294));
#11147=CARTESIAN_POINT('Ctrl Pts',(11.7179528573444,24.6813195394049,-3.05656086386032));
#11148=CARTESIAN_POINT('Ctrl Pts',(11.7518107472756,24.9195717629901,2.92368391516781));
#11149=CARTESIAN_POINT('Ctrl Pts',(8.91973765043983,25.1578239865751,8.19092569431719));
#11150=CARTESIAN_POINT('Ctrl Pts',(3.9123953050936,25.3960762101603,11.4606346444945));
#11151=CARTESIAN_POINT('Ctrl Pts',(-2.04906850960975,25.6343284337454,11.9354221426448));
#11152=CARTESIAN_POINT('Ctrl Pts',(-7.51082304016482,25.8725806573305,9.49950107840742));
#11153=CARTESIAN_POINT('Ctrl Pts',(-11.1409023545732,26.1108328809156,4.74692302501242));
#11154=CARTESIAN_POINT('Ctrl Pts',(-12.0540337900549,26.3490851045007,-1.16329397307453));
#11155=CARTESIAN_POINT('Ctrl Pts',(-10.0275306702439,26.5873373280858,-6.78981679699862));
#11156=CARTESIAN_POINT('Ctrl Pts',(-5.55559922529289,26.8255895516709,-10.7604972342117));
#11157=CARTESIAN_POINT('Ctrl Pts',(0.271184192238789,27.063841775256,-12.1069997362434));
#11158=CARTESIAN_POINT('Ctrl Pts',(6.03183353081841,27.3020939988411,-10.500950801524));
#11159=CARTESIAN_POINT('Ctrl Pts',(10.3214909518584,27.5403462224262,-6.3340198934194));
#11160=CARTESIAN_POINT('Ctrl Pts',(12.0940315311332,27.7785984460113,-0.622402444953652));
#11161=CARTESIAN_POINT('Ctrl Pts',(10.9171832484849,28.0168506695964,5.24100118284009));
#11162=CARTESIAN_POINT('Ctrl Pts',(7.07794578702808,28.2551028931814,9.82627431509112));
#11163=CARTESIAN_POINT('Ctrl Pts',(1.51259950769554,28.4933551167666,12.0151997989567));
#11164=CARTESIAN_POINT('Ctrl Pts',(-4.42162658884796,28.7316073403516,11.2739612287927));
#11165=CARTESIAN_POINT('Ctrl Pts',(-9.27754425042827,28.9698595639368,7.78332552068034));
#11166=CARTESIAN_POINT('Ctrl Pts',(-11.870933853621,29.2081117875218,2.39455902463984));
#11167=CARTESIAN_POINT('Ctrl Pts',(-11.5693417463421,29.446364011107,-3.57817202435472));
#11168=CARTESIAN_POINT('Ctrl Pts',(-8.44631762951329,29.6846162346921,-8.678289116001));
#11169=CARTESIAN_POINT('Ctrl Pts',(-3.26347788572639,29.9228684582772,-11.6620193606813));
#11170=CARTESIAN_POINT('Ctrl Pts',(2.71523090325989,30.1611206818622,-11.801716172723));
#11171=CARTESIAN_POINT('Ctrl Pts',(8.03177242709483,30.3993729054474,-9.06331148967571));
#11172=CARTESIAN_POINT('Ctrl Pts',(11.3895940586429,30.6376251290325,-4.11462399969371));
#11173=CARTESIAN_POINT('Ctrl Pts',(11.9698190077354,30.8758773526176,1.83750276233406));
#11174=CARTESIAN_POINT('Ctrl Pts',(9.63094698161567,31.1141295762027,7.34151508319885));
#11175=CARTESIAN_POINT('Ctrl Pts',(4.94336206482527,31.3523817997878,11.0551415628917));
#11176=CARTESIAN_POINT('Ctrl Pts',(-0.949767667762671,31.5906340233729,
12.0727347712439));
#11177=CARTESIAN_POINT('Ctrl Pts',(-6.61127619335253,31.828886246958,10.1461327891339));
#11178=CARTESIAN_POINT('Ctrl Pts',(-10.6604832859937,32.0671384705431,5.7451788125851));
#11179=CARTESIAN_POINT('Ctrl Pts',(-12.1099029888395,32.3053906941281,-0.0568601831300151));
#11180=CARTESIAN_POINT('Ctrl Pts',(-10.6060632345463,32.5436429177133,-5.84503260421468));
#11181=CARTESIAN_POINT('Ctrl Pts',(-6.51570758666586,32.7818951412983,-10.2077685183684));
#11182=CARTESIAN_POINT('Ctrl Pts',(-0.836356959386205,33.0201473648835,
-12.0811212441569));
#11183=CARTESIAN_POINT('Ctrl Pts',(5.04695724234298,33.2583995884685,-11.0082335582726));
#11184=CARTESIAN_POINT('Ctrl Pts',(9.69946272335483,33.4966518120537,-7.25075212359403));
#11185=CARTESIAN_POINT('Ctrl Pts',(11.9865462812223,33.7349040356388,-1.72501934122564));
#11186=CARTESIAN_POINT('Ctrl Pts',(11.3504535596434,33.9731562592238,4.22139638863183));
#11187=CARTESIAN_POINT('Ctrl Pts',(7.94630940537469,34.211408482809,9.13833411041546));
#11188=CARTESIAN_POINT('Ctrl Pts',(2.6042873488569,34.4496607063941,11.8266931508312));
#11189=CARTESIAN_POINT('Ctrl Pts',(-3.37284600870548,34.6879129299792,11.630859524634));
#11190=CARTESIAN_POINT('Ctrl Pts',(-8.52743855952799,34.9261651535643,8.5985914597323));
#11191=CARTESIAN_POINT('Ctrl Pts',(-11.6024324057451,35.1644173771494,3.46937253010039));
#11192=CARTESIAN_POINT('Ctrl Pts',(-11.8479243752835,35.4026696007345,-2.5059272681298));
#11193=CARTESIAN_POINT('Ctrl Pts',(-9.20404598979087,35.6409218243196,-7.8701029789477));
#11194=CARTESIAN_POINT('Ctrl Pts',(-4.31556367068634,35.8791740479047,-11.3149853598205));
#11195=CARTESIAN_POINT('Ctrl Pts',(1.62536136349889,36.1174262714898,-12.0004659858516));
#11196=CARTESIAN_POINT('Ctrl Pts',(7.16990719156578,36.3556784950749,-9.75937572019344));
#11197=CARTESIAN_POINT('Ctrl Pts',(10.965917427667,36.59393071866,-5.1382524503469));
#11198=CARTESIAN_POINT('Ctrl Pts',(12.0876536389402,36.8321829422451,0.735943809094519));
#11199=CARTESIAN_POINT('Ctrl Pts',(10.2615563171244,37.0704351658302,6.43066444322939));
#11200=CARTESIAN_POINT('Ctrl Pts',(5.93295861336892,37.3086873894153,10.5571295917087));
#11201=CARTESIAN_POINT('Ctrl Pts',(0.157481530964674,37.5469396130003,12.1090125651303));
#11202=CARTESIAN_POINT('Ctrl Pts',(-5.65640033822935,37.7851918365855,10.7078528273879));
#11203=CARTESIAN_POINT('Ctrl Pts',(-10.0908486473709,38.0234440601705,6.69535443070501));
#11204=CARTESIAN_POINT('Ctrl Pts',(-12.0644253281625,38.2616962837557,1.05004869598765));
#11205=CARTESIAN_POINT('Ctrl Pts',(-11.0958369830495,38.4999485073408,-4.85133066267378));
#11206=CARTESIAN_POINT('Ctrl Pts',(-7.42128342921687,38.7382007309259,-9.56961558479783));
#11207=CARTESIAN_POINT('Ctrl Pts',(-1.93690584525694,38.976452954511,-11.954131443005));
#11208=CARTESIAN_POINT('Ctrl Pts',(4.01985793539565,39.2147051780961,-11.4234024767251));
#11209=CARTESIAN_POINT('Ctrl Pts',(8.99623257718483,39.4529574016812,-8.10677890851787));
#11210=CARTESIAN_POINT('Ctrl Pts',(11.7788047335206,39.6912096252663,-2.8132499638494));
#11211=CARTESIAN_POINT('Ctrl Pts',(11.6886183926944,39.9294618488514,3.16656422818516));
#11212=CARTESIAN_POINT('Ctrl Pts',(8.74840425861466,40.1677140724365,8.3737115395636));
#11213=CARTESIAN_POINT('Ctrl Pts',(3.67325831819566,40.4059868433008,11.5399216668183));
#11214=CARTESIAN_POINT('Ctrl Pts',(-0.306162228668456,40.5648422063033,
11.7725256298878));
#11215=CARTESIAN_POINT('Ctrl Pts',(-2.20380626429698,40.6442801614442,11.4058636848336));
#11216=CARTESIAN_POINT('Ctrl Pts',(-2.85929275392902,19.3555908284084,10.6823013608252));
#11217=CARTESIAN_POINT('Ctrl Pts',(-4.63609521571708,19.4350082362701,10.2067111080746));
#11218=CARTESIAN_POINT('Ctrl Pts',(-7.94598089705643,19.5938430519935,8.35217370654499));
#11219=CARTESIAN_POINT('Ctrl Pts',(-10.9739960349335,19.8320952755786,3.53036444489831));
#11220=CARTESIAN_POINT('Ctrl Pts',(-11.3252776421793,20.0703474991637,-2.15121083305315));
#11221=CARTESIAN_POINT('Ctrl Pts',(-8.91488925006696,20.3085997227488,-7.3087422129806));
#11222=CARTESIAN_POINT('Ctrl Pts',(-4.33029369223223,20.5468519463339,-10.683595255436));
#11223=CARTESIAN_POINT('Ctrl Pts',(1.31027690731619,20.785104169919,-11.4531663301778));
#11224=CARTESIAN_POINT('Ctrl Pts',(6.6313382296047,21.0233563935041,-9.42956666052528));
#11225=CARTESIAN_POINT('Ctrl Pts',(10.3351907015071,21.2616086170892,-5.10640017036693));
#11226=CARTESIAN_POINT('Ctrl Pts',(11.5185927548245,21.4998608406743,0.46208898485087));
#11227=CARTESIAN_POINT('Ctrl Pts',(9.89293534220016,21.7381130642594,5.91787911306662));
#11228=CARTESIAN_POINT('Ctrl Pts',(5.85467539640056,21.9763652878445,9.93047189528233));
#11229=CARTESIAN_POINT('Ctrl Pts',(0.388626427785698,22.2146175114296,11.5213040519803));
#11230=CARTESIAN_POINT('Ctrl Pts',(-5.17219697130216,22.4528697350147,10.3024202982052));
#11231=CARTESIAN_POINT('Ctrl Pts',(-9.47166948364905,22.6911219585998,6.57106995376998));
#11232=CARTESIAN_POINT('Ctrl Pts',(-11.4612722248617,22.9293741821849,1.23722359711736));
#11233=CARTESIAN_POINT('Ctrl Pts',(-10.6557980823965,23.16762640577,-4.39834639052438));
#11234=CARTESIAN_POINT('Ctrl Pts',(-7.25167910945802,23.4058786293551,-8.96128525235328));
#11235=CARTESIAN_POINT('Ctrl Pts',(-2.07908273741047,23.6441308529403,-11.3388226254846));
#11236=CARTESIAN_POINT('Ctrl Pts',(3.6005425386876,23.8823830765253,-10.9511450021349));
#11237=CARTESIAN_POINT('Ctrl Pts',(8.40209832447484,24.1206353001105,-7.89279590646365));
#11238=CARTESIAN_POINT('Ctrl Pts',(11.1546223105393,24.3588875236955,-2.90961931837506));
#11239=CARTESIAN_POINT('Ctrl Pts',(11.1868525114124,24.5971397472806,2.78313031517747));
#11240=CARTESIAN_POINT('Ctrl Pts',(8.49092890294339,24.8353919708657,7.79715395735995));
#11241=CARTESIAN_POINT('Ctrl Pts',(3.72431025189639,25.0736441944508,10.9096744503706));
#11242=CARTESIAN_POINT('Ctrl Pts',(-1.95056129610478,25.3118964180359,11.3616369462185));
#11243=CARTESIAN_POINT('Ctrl Pts',(-7.14974665577569,25.550148641621,9.04282070069786));
#11244=CARTESIAN_POINT('Ctrl Pts',(-10.6053130164261,25.7884008652061,4.51871876648054));
#11245=CARTESIAN_POINT('Ctrl Pts',(-11.4745464402741,26.0266530887912,-1.1073696117185));
#11246=CARTESIAN_POINT('Ctrl Pts',(-9.54546572218151,26.2649053123763,-6.46340217018414));
#11247=CARTESIAN_POINT('Ctrl Pts',(-5.28851855109027,26.5031575359614,-10.2431955463965));
#11248=CARTESIAN_POINT('Ctrl Pts',(0.258147244475094,26.7414097595465,-11.5249660939666));
#11249=CARTESIAN_POINT('Ctrl Pts',(5.74185830028796,26.9796619831316,-9.9961265861502));
#11250=CARTESIAN_POINT('Ctrl Pts',(9.82529411504405,27.2179142067167,-6.02951731233947));
#11251=CARTESIAN_POINT('Ctrl Pts',(11.5126213242094,27.4561664303018,-0.592480980520653));
#11252=CARTESIAN_POINT('Ctrl Pts',(10.3923490147401,27.6944186538869,4.98904454006481));
#11253=CARTESIAN_POINT('Ctrl Pts',(6.73767960580988,27.932670877472,9.35388459392002));
#11254=CARTESIAN_POINT('Ctrl Pts',(1.43988258195426,28.1709231010571,11.4375793600353));
#11255=CARTESIAN_POINT('Ctrl Pts',(-4.2090606778576,28.4091753246422,10.7319751992368));
#11256=CARTESIAN_POINT('Ctrl Pts',(-8.83153425711049,28.6474275482273,7.40914881294773));
#11257=CARTESIAN_POINT('Ctrl Pts',(-11.3002488764531,28.8856797718124,2.27944265054878));
#11258=CARTESIAN_POINT('Ctrl Pts',(-11.0131555514081,29.1239319953975,-3.40615446910582));
#11259=CARTESIAN_POINT('Ctrl Pts',(-8.04026814402308,29.3621842189826,-8.2610877999891));
#11260=CARTESIAN_POINT('Ctrl Pts',(-3.10658898164615,29.6004364425677,-11.1013777688193));
#11261=CARTESIAN_POINT('Ctrl Pts',(2.58469850327018,29.8386886661528,-11.2343587762771));
#11262=CARTESIAN_POINT('Ctrl Pts',(7.64565184713929,30.0769408897379,-8.62760055283371));
#11263=CARTESIAN_POINT('Ctrl Pts',(10.8420490798353,30.315193113323,-3.91681697521912));
#11264=CARTESIAN_POINT('Ctrl Pts',(11.3943802114819,30.5534453369081,1.74916639091636));
#11265=CARTESIAN_POINT('Ctrl Pts',(9.16794745469711,30.7916975604932,6.98857803382302));
#11266=CARTESIAN_POINT('Ctrl Pts',(4.70571416771088,31.0299497840783,10.5236751013477));
#11267=CARTESIAN_POINT('Ctrl Pts',(-0.904108400642208,31.2682020076634,
11.4923483878104));
#11268=CARTESIAN_POINT('Ctrl Pts',(-6.29344475313245,31.5064542312485,9.65836614579251));
#11269=CARTESIAN_POINT('Ctrl Pts',(-10.1479896830738,31.7447064548336,5.46898426210454));
#11270=CARTESIAN_POINT('Ctrl Pts',(-11.527729775181,31.9829586784187,-0.0541266785286571));
#11271=CARTESIAN_POINT('Ctrl Pts',(-10.0961858289872,32.2212109020038,-5.56403766822957));
#11272=CARTESIAN_POINT('Ctrl Pts',(-6.20247052535459,32.4594631255889,-9.71703879013706));
#11273=CARTESIAN_POINT('Ctrl Pts',(-0.79614981493094,32.6977153491741,-11.5003316882214));
#11274=CARTESIAN_POINT('Ctrl Pts',(4.80432909580209,32.9359675727591,-10.4790221588725));
#11275=CARTESIAN_POINT('Ctrl Pts',(9.23316936083815,33.1742197963443,-6.90217842575973));
#11276=CARTESIAN_POINT('Ctrl Pts',(11.4103033356234,33.4124720199293,-1.64209051393198));
#11277=CARTESIAN_POINT('Ctrl Pts',(10.8047902268001,33.6507242435144,4.01845637301311));
#11278=CARTESIAN_POINT('Ctrl Pts',(7.56429738698645,33.8889764670995,8.69901652534074));
#11279=CARTESIAN_POINT('Ctrl Pts',(2.47908846521831,34.1272286906846,11.2581350075564));
#11280=CARTESIAN_POINT('Ctrl Pts',(-3.21069932579042,34.3654809142697,11.0717159152007));
#11281=CARTESIAN_POINT('Ctrl Pts',(-8.11748925481006,34.6037331378548,8.18522154028186));
#11282=CARTESIAN_POINT('Ctrl Pts',(-11.0446554057036,34.8419853614399,3.30258541734742));
#11283=CARTESIAN_POINT('Ctrl Pts',(-11.2783455590783,35.080237585025,-2.38545696112353));
#11284=CARTESIAN_POINT('Ctrl Pts',(-8.76156936239957,35.3184898086102,-7.49175451923664));
#11285=CARTESIAN_POINT('Ctrl Pts',(-4.10809664364021,35.5567420321952,-10.771027130304));
#11286=CARTESIAN_POINT('Ctrl Pts',(1.5472235081241,35.7949942557803,-11.4235538623753));
#11287=CARTESIAN_POINT('Ctrl Pts',(6.82522004459241,36.0332464793655,-9.2902020916712));
#11288=CARTESIAN_POINT('Ctrl Pts',(10.4387403400005,36.2714987029505,-4.89123536487858));
#11289=CARTESIAN_POINT('Ctrl Pts',(11.5065500437207,36.5097509265356,0.70056394083236));
#11290=CARTESIAN_POINT('Ctrl Pts',(9.76824078653887,36.7480031501207,6.12151575819658));
#11291=CARTESIAN_POINT('Ctrl Pts',(5.64773670980524,36.9862553737058,10.0496046291158));
#11292=CARTESIAN_POINT('Ctrl Pts',(0.149910741251658,37.2245075972909,11.5268821578289));
#11293=CARTESIAN_POINT('Ctrl Pts',(-5.38447373686177,37.4627598208761,10.1930819743391));
#11294=CARTESIAN_POINT('Ctrl Pts',(-9.60573974179206,37.7010120444611,6.37348100123998));
#11295=CARTESIAN_POINT('Ctrl Pts',(-11.4844384140878,37.9392642680463,0.999568504329265));
#11296=CARTESIAN_POINT('Ctrl Pts',(-10.5624141240384,38.1775164916313,-4.61810709638991));
#11297=CARTESIAN_POINT('Ctrl Pts',(-7.06451158493042,38.4157687152165,-9.10956451224892));
#11298=CARTESIAN_POINT('Ctrl Pts',(-1.84379075576973,38.6540209388016,-11.379446812989));
#11299=CARTESIAN_POINT('Ctrl Pts',(3.82660670829195,38.8922731623866,-10.8742321871762));
#11300=CARTESIAN_POINT('Ctrl Pts',(8.56374640160554,39.1305253859717,-7.71705245621345));
#11301=CARTESIAN_POINT('Ctrl Pts',(11.2125487848899,39.3687776095568,-2.67800538147839));
#11302=CARTESIAN_POINT('Ctrl Pts',(11.1266980751514,39.607029833142,3.01433436518149));
#11303=CARTESIAN_POINT('Ctrl Pts',(8.32783221717754,39.845282056727,7.97115252965823));
#11304=CARTESIAN_POINT('Ctrl Pts',(3.49666957081488,40.0835548275914,10.9851498170082));
#11305=CARTESIAN_POINT('Ctrl Pts',(-0.291443741763231,40.2424101905938,
11.2065715437861));
#11306=CARTESIAN_POINT('Ctrl Pts',(-2.09786016577339,40.3218481457347,10.8575365576823));
#11307=CARTESIAN_POINT('Ctrl Pts',(-2.71489279974816,19.033158812699,10.1428239586147));
#11308=CARTESIAN_POINT('Ctrl Pts',(-4.40196321373591,19.1125762205607,9.69125195674494));
#11309=CARTESIAN_POINT('Ctrl Pts',(-7.54469310451393,19.2714110362841,7.93037237162453));
#11310=CARTESIAN_POINT('Ctrl Pts',(-10.4197874732365,19.5096632598692,3.35207403955784));
#11311=CARTESIAN_POINT('Ctrl Pts',(-10.7533286627092,19.7479154834543,-2.04257042003514));
#11312=CARTESIAN_POINT('Ctrl Pts',(-8.46466966430815,19.9861677070394,-6.9396362376572));
#11313=CARTESIAN_POINT('Ctrl Pts',(-4.11160527360535,20.2244199306245,-10.1440525089817));
#11314=CARTESIAN_POINT('Ctrl Pts',(1.24410532515808,20.4626721542096,-10.8747587183546));
#11315=CARTESIAN_POINT('Ctrl Pts',(6.29644249876465,20.7009243777947,-8.95335484490964));
#11316=CARTESIAN_POINT('Ctrl Pts',(9.81324307592822,20.9391766013798,-4.84851683553984));
#11317=CARTESIAN_POINT('Ctrl Pts',(10.936880978813,21.177428824965,0.438752574772446));
#11318=CARTESIAN_POINT('Ctrl Pts',(9.39332248927878,21.41568104855,5.6190144824336));
#11319=CARTESIAN_POINT('Ctrl Pts',(5.55900267879502,21.6539332721351,9.42896337199362));
#11320=CARTESIAN_POINT('Ctrl Pts',(0.369000022518657,21.8921854957201,10.9394553500859));
#11321=CARTESIAN_POINT('Ctrl Pts',(-4.9109907675498,22.1304377193053,9.78212764297827));
#11322=CARTESIAN_POINT('Ctrl Pts',(-8.99333139197382,22.3686899428904,6.23921789037432));
#11323=CARTESIAN_POINT('Ctrl Pts',(-10.8824552492826,22.6069421664755,1.17474135199233));
#11324=CARTESIAN_POINT('Ctrl Pts',(-10.1176591483038,22.8451943900607,-4.17622117568216));
#11325=CARTESIAN_POINT('Ctrl Pts',(-6.88545493402124,23.0834466136456,-8.50872257647364));
#11326=CARTESIAN_POINT('Ctrl Pts',(-1.9740849362557,23.3216988372308,-10.7661895974971));
#11327=CARTESIAN_POINT('Ctrl Pts',(3.41870800044444,23.5599510608158,-10.398090462909));
#11328=CARTESIAN_POINT('Ctrl Pts',(7.97777569734612,23.798203284401,-7.49419406141432));
#11329=CARTESIAN_POINT('Ctrl Pts',(10.5912917637341,24.0364555079861,-2.76267777288981));
#11330=CARTESIAN_POINT('Ctrl Pts',(10.6218942755493,24.2747077315713,2.64257671518715));
#11331=CARTESIAN_POINT('Ctrl Pts',(8.06212015544694,24.5129599551563,7.4033822204027));
#11332=CARTESIAN_POINT('Ctrl Pts',(3.53622519869919,24.7512121787414,10.3587142562468));
#11333=CARTESIAN_POINT('Ctrl Pts',(-1.85205408259982,24.9894644023265,10.7878517497922));
#11334=CARTESIAN_POINT('Ctrl Pts',(-6.78867027138654,25.2277166259116,8.5861403229883));
#11335=CARTESIAN_POINT('Ctrl Pts',(-10.0697236782791,25.4659688494967,4.29051450794865));
#11336=CARTESIAN_POINT('Ctrl Pts',(-10.8950590904933,25.7042210730819,-1.05144525036245));
#11337=CARTESIAN_POINT('Ctrl Pts',(-9.06340077411911,25.942473296667,-6.13698754336968));
#11338=CARTESIAN_POINT('Ctrl Pts',(-5.02143787688763,26.180725520252,-9.72589385858134));
#11339=CARTESIAN_POINT('Ctrl Pts',(0.245110296711381,26.4189777438371,-10.9429324516899));
#11340=CARTESIAN_POINT('Ctrl Pts',(5.45188306975753,26.6572299674222,-9.49130237077641));
#11341=CARTESIAN_POINT('Ctrl Pts',(9.32909727822967,26.8954821910073,-5.72501473125955));
#11342=CARTESIAN_POINT('Ctrl Pts',(10.9312111172857,27.1337344145924,-0.562559516087658));
#11343=CARTESIAN_POINT('Ctrl Pts',(9.86751478099552,27.3719866381776,4.73708789728954));
#11344=CARTESIAN_POINT('Ctrl Pts',(6.3974134245917,27.6102388617626,8.8814948727489));
#11345=CARTESIAN_POINT('Ctrl Pts',(1.367165656213,27.8484910853477,10.8599589211139));
#11346=CARTESIAN_POINT('Ctrl Pts',(-3.99649476686722,28.0867433089328,10.1899891696809));
#11347=CARTESIAN_POINT('Ctrl Pts',(-8.38552426379272,28.3249955325179,7.03497210521514));
#11348=CARTESIAN_POINT('Ctrl Pts',(-10.7295638992853,28.563247756103,2.16432627645773));
#11349=CARTESIAN_POINT('Ctrl Pts',(-10.4569693564742,28.8014999796882,-3.23413691385691));
#11350=CARTESIAN_POINT('Ctrl Pts',(-7.63421865853288,29.0397522032733,-7.84388648397718));
#11351=CARTESIAN_POINT('Ctrl Pts',(-2.94970007756592,29.2780044268583,-10.5407361769574));
#11352=CARTESIAN_POINT('Ctrl Pts',(2.45416610328047,29.5162566504434,-10.6670013798312));
#11353=CARTESIAN_POINT('Ctrl Pts',(7.25953126718375,29.7545088740285,-8.19188961599171));
#11354=CARTESIAN_POINT('Ctrl Pts',(10.2945041010277,29.9927610976136,-3.71900995074453));
#11355=CARTESIAN_POINT('Ctrl Pts',(10.8189414152284,30.2310133211988,1.66083001949865));
#11356=CARTESIAN_POINT('Ctrl Pts',(8.70494792777857,30.4692655447839,6.63564098444718));
#11357=CARTESIAN_POINT('Ctrl Pts',(4.46806627059647,30.7075177683689,9.9922086398038));
#11358=CARTESIAN_POINT('Ctrl Pts',(-0.858449133521731,30.945769991954,10.911962004377));
#11359=CARTESIAN_POINT('Ctrl Pts',(-5.97561331291237,31.1840222155391,9.17059950245109));
#11360=CARTESIAN_POINT('Ctrl Pts',(-9.63549608015401,31.4222744391242,5.19278971162398));
#11361=CARTESIAN_POINT('Ctrl Pts',(-10.9455565615224,31.6605266627094,-0.0513931739272948));
#11362=CARTESIAN_POINT('Ctrl Pts',(-9.58630842342816,31.8987788862945,-5.28304273224449));
#11363=CARTESIAN_POINT('Ctrl Pts',(-5.88923346404332,32.1370311098796,-9.2263090619057));
#11364=CARTESIAN_POINT('Ctrl Pts',(-0.755942670475671,32.3752833334646,
-10.919542132286));
#11365=CARTESIAN_POINT('Ctrl Pts',(4.56170094926121,32.6135355570497,-9.94981075947233));
#11366=CARTESIAN_POINT('Ctrl Pts',(8.76687599832148,32.8517877806348,-6.55360472792545));
#11367=CARTESIAN_POINT('Ctrl Pts',(10.8340603900244,33.0900400042199,-1.55916168663833));
#11368=CARTESIAN_POINT('Ctrl Pts',(10.2591268939567,33.3282922278051,3.81551635739438));
#11369=CARTESIAN_POINT('Ctrl Pts',(7.18228536859824,33.5665444513902,8.25969894026603));
#11370=CARTESIAN_POINT('Ctrl Pts',(2.35388958157973,33.8047966749752,10.6895768642816));
#11371=CARTESIAN_POINT('Ctrl Pts',(-3.04855264287536,34.0430488985603,10.5125723057673));
#11372=CARTESIAN_POINT('Ctrl Pts',(-7.70753995009214,34.2813011221453,7.77185162083141));
#11373=CARTESIAN_POINT('Ctrl Pts',(-10.4868784056621,34.5195533457305,3.13579830459444));
#11374=CARTESIAN_POINT('Ctrl Pts',(-10.7087667428733,34.7578055693157,-2.26498665411725));
#11375=CARTESIAN_POINT('Ctrl Pts',(-8.31909273500825,34.9960577929008,-7.11340605952559));
#11376=CARTESIAN_POINT('Ctrl Pts',(-3.90062961659408,35.2343100164858,-10.2270689007874));
#11377=CARTESIAN_POINT('Ctrl Pts',(1.46908565274932,35.4725622400709,-10.846641738899));
#11378=CARTESIAN_POINT('Ctrl Pts',(6.48053289761904,35.710814463656,-8.82102846314895));
#11379=CARTESIAN_POINT('Ctrl Pts',(9.91156325233417,35.9490666872411,-4.64421827941024));
#11380=CARTESIAN_POINT('Ctrl Pts',(10.9254464485013,36.1873189108261,0.665184072570199));
#11381=CARTESIAN_POINT('Ctrl Pts',(9.27492525595335,36.4255711344113,5.81236707316377));
#11382=CARTESIAN_POINT('Ctrl Pts',(5.36251480624159,36.6638233579963,9.54207966652283));
#11383=CARTESIAN_POINT('Ctrl Pts',(0.142339951538634,36.9020755815815,10.9447517505275));
#11384=CARTESIAN_POINT('Ctrl Pts',(-5.11254713549418,37.1403278051666,9.67831112129031));
#11385=CARTESIAN_POINT('Ctrl Pts',(-9.12063083621321,37.3785800287517,6.05160757177495));
#11386=CARTESIAN_POINT('Ctrl Pts',(-10.9044515000132,37.6168322523368,0.949088312670873));
#11387=CARTESIAN_POINT('Ctrl Pts',(-10.0289912650274,37.855084475922,-4.38488353010602));
#11388=CARTESIAN_POINT('Ctrl Pts',(-6.707739740644,38.093336699507,-8.64951343970004));
#11389=CARTESIAN_POINT('Ctrl Pts',(-1.75067566628252,38.3315889230921,-10.8047621829729));
#11390=CARTESIAN_POINT('Ctrl Pts',(3.63335548118823,38.5698411466772,-10.3250618976272));
#11391=CARTESIAN_POINT('Ctrl Pts',(8.13126022602624,38.8080933702623,-7.32732600390901));
#11392=CARTESIAN_POINT('Ctrl Pts',(10.6462928362593,39.0463455938474,-2.54276079910738));
#11393=CARTESIAN_POINT('Ctrl Pts',(10.5647777576085,39.2845978174326,2.86210450217782));
#11394=CARTESIAN_POINT('Ctrl Pts',(7.90726017574041,39.5228500410177,7.56859351975284));
#11395=CARTESIAN_POINT('Ctrl Pts',(3.32008082343409,39.7611228118819,10.430377967198));
#11396=CARTESIAN_POINT('Ctrl Pts',(-0.276725254858005,39.9199781748845,
10.6406174576843));
#11397=CARTESIAN_POINT('Ctrl Pts',(-1.99191406724981,39.9994161300253,10.309209430531));
#11398=CARTESIAN_POINT('Ctrl Pts',(-1.99079507083261,40.,10.3105642903746));
#11399=CARTESIAN_POINT('Ctrl Pts',(-1.74787308387841,40.,10.3776190639041));
#11400=CARTESIAN_POINT('Ctrl Pts',(-1.50291730396296,40.,10.4356201925428));
#11401=CARTESIAN_POINT('Ctrl Pts',(-1.25645144932171,40.,10.4847082098123));
#11402=CARTESIAN_POINT('Ctrl Pts',(-1.00610937738997,40.,10.5345682440478));
#11403=CARTESIAN_POINT('Ctrl Pts',(-0.754208867844965,40.,10.5752327777935));
#11404=CARTESIAN_POINT('Ctrl Pts',(-0.501269410076261,40.,10.6068040927733));
#11405=CARTESIAN_POINT('Ctrl Pts',(-0.244349094599502,40.,10.638872289156));
#11406=CARTESIAN_POINT('Ctrl Pts',(0.0136436862107205,40.,10.6615589815521));
#11407=CARTESIAN_POINT('Ctrl Pts',(0.272186552083508,40.,10.6749225223864));
#11408=CARTESIAN_POINT('Ctrl Pts',(0.531566233231362,40.,10.6883293164547));
#11409=CARTESIAN_POINT('Ctrl Pts',(0.79150020091699,40.,10.6923526126103));
#11410=CARTESIAN_POINT('Ctrl Pts',(1.05147389557568,40.,10.6870004795277));
#11411=CARTESIAN_POINT('Ctrl Pts',(1.31028375616657,40.,10.6816723065417));
#11412=CARTESIAN_POINT('Ctrl Pts',(1.56913363753882,40.,10.667052504031));
#11413=CARTESIAN_POINT('Ctrl Pts',(1.82751900740169,40.,10.6430977087009));
#11414=CARTESIAN_POINT('Ctrl Pts',(1.90159763837717,40.,10.6362299110222));
#11415=CARTESIAN_POINT('Ctrl Pts',(1.97563807441582,40.,10.62859448903));
#11416=CARTESIAN_POINT('Ctrl Pts',(2.04962835769163,40.,10.6201896290691));
#11417=CARTESIAN_POINT('Ctrl Pts',(2.08954125923063,40.,10.6156557587659));
#11418=CARTESIAN_POINT('Ctrl Pts',(2.12944528573599,40.,10.6108972103674));
#11419=CARTESIAN_POINT('Ctrl Pts',(2.1693057513364,40.,10.6059179310049));
#11420=CARTESIAN_POINT('Ctrl Pts',(2.43279869411477,40.,10.5730029875293));
#11421=CARTESIAN_POINT('Ctrl Pts',(2.69461388759011,40.,10.5304238386819));
#11422=CARTESIAN_POINT('Ctrl Pts',(2.95420990430317,40.,10.4782725649796));
#11423=CARTESIAN_POINT('Ctrl Pts',(3.07376860221186,40.,10.4542539438271));
#11424=CARTESIAN_POINT('Ctrl Pts',(3.19285681334819,40.,10.4282042572862));
#11425=CARTESIAN_POINT('Ctrl Pts',(3.31142253876288,40.,10.4001289044428));
#11426=CARTESIAN_POINT('Ctrl Pts',(3.56622266861186,40.,10.3397944062138));
#11427=CARTESIAN_POINT('Ctrl Pts',(3.81860986323782,40.,10.2701083948083));
#11428=CARTESIAN_POINT('Ctrl Pts',(4.06816673278697,40.,10.1914106777718));
#11429=CARTESIAN_POINT('Ctrl Pts',(4.32019405300233,40.,10.1119339045312));
#11430=CARTESIAN_POINT('Ctrl Pts',(4.56933530459187,40.,10.0232659756233));
#11431=CARTESIAN_POINT('Ctrl Pts',(4.81515658717821,40.,9.92570343342688));
#11432=CARTESIAN_POINT('Ctrl Pts',(5.0619503348636,40.,9.82775493535928));
#11433=CARTESIAN_POINT('Ctrl Pts',(5.30539839347577,40.,9.72084110650416));
#11434=CARTESIAN_POINT('Ctrl Pts',(5.54504886067588,40.,9.60521113795994));
#11435=CARTESIAN_POINT('Ctrl Pts',(5.66474353075312,40.,9.54745914983473));
#11436=CARTESIAN_POINT('Ctrl Pts',(5.7834906148258,40.,9.48753209970937));
#11437=CARTESIAN_POINT('Ctrl Pts',(5.90123189477887,40.,9.42545655578914));
#11438=CARTESIAN_POINT('Ctrl Pts',(5.95755288857904,40.,9.39576300798952));
#11439=CARTESIAN_POINT('Ctrl Pts',(6.0136437182583,40.,9.36557781144656));
#11440=CARTESIAN_POINT('Ctrl Pts',(6.06949788210085,40.,9.33490364295837));
#11441=CARTESIAN_POINT('Ctrl Pts',(6.11005050514561,40.,9.31263282362574));
#11442=CARTESIAN_POINT('Ctrl Pts',(6.15048573176791,40.,9.29010000366931));
#11443=CARTESIAN_POINT('Ctrl Pts',(6.19076456917044,40.,9.26732701566816));
#11444=CARTESIAN_POINT('Ctrl Pts',(6.42582634078894,40.,9.13442698056777));
#11445=CARTESIAN_POINT('Ctrl Pts',(6.65571575867433,40.,8.99327172535973));
#11446=CARTESIAN_POINT('Ctrl Pts',(6.8800037608189,40.,8.8442223141287));
#11447=CARTESIAN_POINT('Ctrl Pts',(7.10949099987972,40.,8.69171777737241));
#11448=CARTESIAN_POINT('Ctrl Pts',(7.33311477943246,40.,8.53094877669126));
#11449=CARTESIAN_POINT('Ctrl Pts',(7.55040528259981,40.,8.36224719022096));
#11450=CARTESIAN_POINT('Ctrl Pts',(7.76769578576717,40.,8.19354560375065));
#11451=CARTESIAN_POINT('Ctrl Pts',(7.97865366192367,40.,8.01691114350707));
#11452=CARTESIAN_POINT('Ctrl Pts',(8.18278913651048,40.,7.83262450231714));
#11453=CARTESIAN_POINT('Ctrl Pts',(8.3828805419461,40.,7.65198871075106));
#11454=CARTESIAN_POINT('Ctrl Pts',(8.57641773083029,40.,7.46400053667558));
#11455=CARTESIAN_POINT('Ctrl Pts',(8.76315973735538,40.,7.26911327772968));
#11456=CARTESIAN_POINT('Ctrl Pts',(8.95087399741526,40.,7.07321135780887));
#11457=CARTESIAN_POINT('Ctrl Pts',(9.13172256221306,40.,6.87033788468238));
#11458=CARTESIAN_POINT('Ctrl Pts',(9.305425145709,40.,6.66091475544659));
#11459=CARTESIAN_POINT('Ctrl Pts',(9.35096602906598,40.,6.60600875399955));
#11460=CARTESIAN_POINT('Ctrl Pts',(9.39601551120144,40.,6.5506523646528));
#11461=CARTESIAN_POINT('Ctrl Pts',(9.44056808201162,40.,6.49485281517297));
#11462=CARTESIAN_POINT('Ctrl Pts',(9.45871046836229,40.,6.47213051281313));
#11463=CARTESIAN_POINT('Ctrl Pts',(9.4767704796353,40.,6.44933463079931));
#11464=CARTESIAN_POINT('Ctrl Pts',(9.49473878095482,40.,6.42647721576431));
#11465=CARTESIAN_POINT('Ctrl Pts',(9.66342503031443,40.,6.21189201131206));
#11466=CARTESIAN_POINT('Ctrl Pts',(9.82423055529979,40.,5.99163828046606));
#11467=CARTESIAN_POINT('Ctrl Pts',(9.97696748002078,40.,5.76623949569044));
#11468=CARTESIAN_POINT('Ctrl Pts',(10.132296481448,40.,5.53701550007802));
#11469=CARTESIAN_POINT('Ctrl Pts',(10.2792811505019,40.,5.30246996680171));
#11470=CARTESIAN_POINT('Ctrl Pts',(10.417694044559,40.,5.06310861315508));
#11471=CARTESIAN_POINT('Ctrl Pts',(10.5565955437288,40.,4.82290230079295));
#11472=CARTESIAN_POINT('Ctrl Pts',(10.6868650563927,40.,4.57784561876773));
#11473=CARTESIAN_POINT('Ctrl Pts',(10.8082364605648,40.,4.32841151267132));
#11474=CARTESIAN_POINT('Ctrl Pts',(10.9290278820725,40.,4.08016934678893));
#11475=CARTESIAN_POINT('Ctrl Pts',(11.0410063966906,40.,3.82759096156524));
#11476=CARTESIAN_POINT('Ctrl Pts',(11.1438680898851,40.,3.5711125486244));
#11477=CARTESIAN_POINT('Ctrl Pts',(11.210257734195,40.,3.40557462989577));
#11478=CARTESIAN_POINT('Ctrl Pts',(11.2728486825664,40.,3.23841146991623));
#11479=CARTESIAN_POINT('Ctrl Pts',(11.3315488558307,40.,3.06973522608137));
#11480=CARTESIAN_POINT('Ctrl Pts',(11.3969138737467,40.,2.88190740399589));
#11481=CARTESIAN_POINT('Ctrl Pts',(11.4574546537082,40.,2.69220336876743));
#11482=CARTESIAN_POINT('Ctrl Pts',(11.5131538719282,40.,2.50080739873));
#11483=CARTESIAN_POINT('Ctrl Pts',(11.5219564527078,40.,2.47055960457811));
#11484=CARTESIAN_POINT('Ctrl Pts',(11.5306367798565,40.,2.44027394775997));
#11485=CARTESIAN_POINT('Ctrl Pts',(11.5391927173603,40.,2.40995901899243));
#11486=CARTESIAN_POINT('Ctrl Pts',(11.6149930718682,40.,2.14138735791638));
#11487=CARTESIAN_POINT('Ctrl Pts',(11.6810877877354,40.,1.87033611873908));
#11488=CARTESIAN_POINT('Ctrl Pts',(11.7375427831218,40.,1.59736118879834));
#11489=CARTESIAN_POINT('Ctrl Pts',(11.7945063360496,40.,1.32192724777677));
#11490=CARTESIAN_POINT('Ctrl Pts',(11.84165587897,40.,1.04453424120747));
#11491=CARTESIAN_POINT('Ctrl Pts',(11.8790117311798,40.,0.765728997851488));
#11492=CARTESIAN_POINT('Ctrl Pts',(11.9165716381981,40.,0.485400792305021));
#11493=CARTESIAN_POINT('Ctrl Pts',(11.9442307186072,40.,0.203644272153142));
#11494=CARTESIAN_POINT('Ctrl Pts',(11.9619595697314,40.,-0.079000249593141));
#11495=CARTESIAN_POINT('Ctrl Pts',(11.9657577577725,40.,-0.139553357906196));
#11496=CARTESIAN_POINT('Ctrl Pts',(11.9690999836776,40.,-0.200147260578903));
#11497=CARTESIAN_POINT('Ctrl Pts',(11.9719856511623,40.,-0.260776694674976));
#11498=CARTESIAN_POINT('Ctrl Pts',(11.9737712450156,40.,-0.298292986980646));
#11499=CARTESIAN_POINT('Ctrl Pts',(11.9753819638708,40.,-0.335822485014976));
#11500=CARTESIAN_POINT('Ctrl Pts',(11.9768172604587,40.,-0.37335023804946));
#11501=CARTESIAN_POINT('Ctrl Pts',(11.9877545329118,40.,-0.659319885686097));
#11502=CARTESIAN_POINT('Ctrl Pts',(11.9885197420998,40.,-0.945390292321608));
#11503=CARTESIAN_POINT('Ctrl Pts',(11.9791433269757,40.,-1.23099730766982));
#11504=CARTESIAN_POINT('Ctrl Pts',(11.9697517430833,40.,-1.51706636598248));
#11505=CARTESIAN_POINT('Ctrl Pts',(11.9501858036841,40.,-1.80267116625394));
#11506=CARTESIAN_POINT('Ctrl Pts',(11.920425517138,40.,-2.08725729224288));
#11507=CARTESIAN_POINT('Ctrl Pts',(11.894682539692,40.,-2.33342744290519));
#11508=CARTESIAN_POINT('Ctrl Pts',(11.8613109472795,40.,-2.57883581888343));
#11509=CARTESIAN_POINT('Ctrl Pts',(11.8202663870092,40.,-2.82312554759088));
#11510=CARTESIAN_POINT('Ctrl Pts',(11.8016841988292,40.,-2.93372333885433));
#11511=CARTESIAN_POINT('Ctrl Pts',(11.7815289081037,40.,-3.04409183784577));
#11512=CARTESIAN_POINT('Ctrl Pts',(11.7598151666302,40.,-3.1542027559576));
#11513=CARTESIAN_POINT('Ctrl Pts',(-3.14788895504392,20.,11.7604951161383));
#11514=CARTESIAN_POINT('Ctrl Pts',(-3.41583726409301,20.,11.6689078365353));
#11515=CARTESIAN_POINT('Ctrl Pts',(-3.6800281171579,20.,11.5679423474188));
#11516=CARTESIAN_POINT('Ctrl Pts',(-3.9400576560663,20.,11.4579525320777));
#11517=CARTESIAN_POINT('Ctrl Pts',(-4.20217416504438,20.,11.3470799499035));
#11518=CARTESIAN_POINT('Ctrl Pts',(-4.46006282882018,20.,11.2270372658007));
#11519=CARTESIAN_POINT('Ctrl Pts',(-4.71328870839101,20.,11.0981380892181));
#11520=CARTESIAN_POINT('Ctrl Pts',(-4.96683786887351,20.,10.9690743534546));
#11521=CARTESIAN_POINT('Ctrl Pts',(-5.21571284554744,20.,10.83113111242));
#11522=CARTESIAN_POINT('Ctrl Pts',(-5.45944793424098,20.,10.6845799111558));
#11523=CARTESIAN_POINT('Ctrl Pts',(-5.70414316212735,20.,10.5374514046179));
#11524=CARTESIAN_POINT('Ctrl Pts',(-5.94365846472394,20.,10.3816466219635));
#11525=CARTESIAN_POINT('Ctrl Pts',(-6.17748537895062,20.,10.217402357069));
#11526=CARTESIAN_POINT('Ctrl Pts',(-6.35285556462064,20.,10.0942191583982));
#11527=CARTESIAN_POINT('Ctrl Pts',(-6.52502531488677,20.,9.96628793618934));
#11528=CARTESIAN_POINT('Ctrl Pts',(-6.69376370917604,20.,9.83369652447978));
#11529=CARTESIAN_POINT('Ctrl Pts',(-6.820317504893,20.,9.73425296569761));
#11530=CARTESIAN_POINT('Ctrl Pts',(-6.94494088210404,20.,9.63218783287827));
#11531=CARTESIAN_POINT('Ctrl Pts',(-7.06753052972854,20.,9.52753487809413));
#11532=CARTESIAN_POINT('Ctrl Pts',(-7.10083026097056,20.,9.49910739391806));
#11533=CARTESIAN_POINT('Ctrl Pts',(-7.13398139822032,20.,9.47048763974647));
#11534=CARTESIAN_POINT('Ctrl Pts',(-7.16697685356759,20.,9.44168058839424));
#11535=CARTESIAN_POINT('Ctrl Pts',(-7.19428556748663,20.,9.41783841025336));
#11536=CARTESIAN_POINT('Ctrl Pts',(-7.22148095759086,20.,9.39387375887951));
#11537=CARTESIAN_POINT('Ctrl Pts',(-7.24855699528293,20.,9.36979178935576));
#11538=CARTESIAN_POINT('Ctrl Pts',(-7.45693217325836,20.,9.18445873794766));
#11539=CARTESIAN_POINT('Ctrl Pts',(-7.65835188432274,20.,8.99208370611105));
#11540=CARTESIAN_POINT('Ctrl Pts',(-7.85239628045986,20.,8.79294161458531));
#11541=CARTESIAN_POINT('Ctrl Pts',(-7.93912888420864,20.,8.70393047869144));
#11542=CARTESIAN_POINT('Ctrl Pts',(-8.02438754640145,20.,8.61356687435558));
#11543=CARTESIAN_POINT('Ctrl Pts',(-8.1081323460688,20.,8.52187300942612));
#11544=CARTESIAN_POINT('Ctrl Pts',(-8.29599191369493,20.,8.31618179172615));
#11545=CARTESIAN_POINT('Ctrl Pts',(-8.47623651864031,20.,8.10379842051365));
#11546=CARTESIAN_POINT('Ctrl Pts',(-8.64862143631702,20.,7.88521040928684));
#11547=CARTESIAN_POINT('Ctrl Pts',(-8.82101815485311,20.,7.66660743430092));
#11548=CARTESIAN_POINT('Ctrl Pts',(-8.98555437557762,20.,7.44179836758922));
#11549=CARTESIAN_POINT('Ctrl Pts',(-9.14193907463545,20.,7.21124696764572));
#11550=CARTESIAN_POINT('Ctrl Pts',(-9.29725248533917,20.,6.9822749231716));
#11551=CARTESIAN_POINT('Ctrl Pts',(-9.44452587936642,20.,6.74763835396367));
#11552=CARTESIAN_POINT('Ctrl Pts',(-9.58342512130665,20.,6.50777699622786));
#11553=CARTESIAN_POINT('Ctrl Pts',(-9.65196330298591,20.,6.38942025730912));
#11554=CARTESIAN_POINT('Ctrl Pts',(-9.71846176138575,20.,6.26979121209968));
#11555=CARTESIAN_POINT('Ctrl Pts',(-9.7828756676878,20.,6.14894204377767));
#11556=CARTESIAN_POINT('Ctrl Pts',(-9.8132088705112,20.,6.0920328677286));
#11557=CARTESIAN_POINT('Ctrl Pts',(-9.84307976363647,20.,6.03485311738496));
#11558=CARTESIAN_POINT('Ctrl Pts',(-9.87248341765159,20.,5.97740823126373));
#11559=CARTESIAN_POINT('Ctrl Pts',(-9.88901621089197,20.,5.94510869378205));
#11560=CARTESIAN_POINT('Ctrl Pts',(-9.90540128472552,20.,5.91272533420826));
#11561=CARTESIAN_POINT('Ctrl Pts',(-9.92163774038952,20.,5.88025911929686));
#11562=CARTESIAN_POINT('Ctrl Pts',(-9.93566445772471,20.,5.85221146967865));
#11563=CARTESIAN_POINT('Ctrl Pts',(-9.94957694938171,20.,5.82410855112396));
#11564=CARTESIAN_POINT('Ctrl Pts',(-9.96337153280697,20.,5.79595784393599));
#11565=CARTESIAN_POINT('Ctrl Pts',(-10.0085819479117,20.,5.70369661949572));
#11566=CARTESIAN_POINT('Ctrl Pts',(-10.0525370783396,20.,5.61089988168351));
#11567=CARTESIAN_POINT('Ctrl Pts',(-10.0952260574459,20.,5.51759230643859));
#11568=CARTESIAN_POINT('Ctrl Pts',(-10.2089718891463,20.,5.26897198399479));
#11569=CARTESIAN_POINT('Ctrl Pts',(-10.3137316524454,20.,5.01672675586682));
#11570=CARTESIAN_POINT('Ctrl Pts',(-10.409265014146,20.,4.76131291339675));
#11571=CARTESIAN_POINT('Ctrl Pts',(-10.5040506875237,20.,4.50789805792076));
#11572=CARTESIAN_POINT('Ctrl Pts',(-10.5897539804176,20.,4.25136340325132));
#11573=CARTESIAN_POINT('Ctrl Pts',(-10.6660911547673,20.,3.99214066991294));
#11574=CARTESIAN_POINT('Ctrl Pts',(-10.7164100476478,20.,3.82126977952232));
#11575=CARTESIAN_POINT('Ctrl Pts',(-10.7626583544202,20.,3.64923065117632));
#11576=CARTESIAN_POINT('Ctrl Pts',(-10.8047424783443,20.,3.47614542570932));
#11577=CARTESIAN_POINT('Ctrl Pts',(-10.8705314538897,20.,3.20556596239269));
#11578=CARTESIAN_POINT('Ctrl Pts',(-10.9261465394823,20.,2.93242944986049));
#11579=CARTESIAN_POINT('Ctrl Pts',(-10.971539533839,20.,2.65731524077356));
#11580=CARTESIAN_POINT('Ctrl Pts',(-11.0169325281957,20.,2.38220103168662));
#11581=CARTESIAN_POINT('Ctrl Pts',(-11.0521033806315,20.,2.10510839212968));
#11582=CARTESIAN_POINT('Ctrl Pts',(-11.0769480123086,20.,1.82662914162098));
#11583=CARTESIAN_POINT('Ctrl Pts',(-11.0805510773543,20.,1.78624299838922));
#11584=CARTESIAN_POINT('Ctrl Pts',(-11.0839368669433,20.,1.74582772459025));
#11585=CARTESIAN_POINT('Ctrl Pts',(-11.0871049669885,20.,1.70538516141017));
#11586=CARTESIAN_POINT('Ctrl Pts',(-11.0904162776532,20.,1.6631144348383));
#11587=CARTESIAN_POINT('Ctrl Pts',(-11.093490147485,20.,1.62080741465348));
#11588=CARTESIAN_POINT('Ctrl Pts',(-11.0963238911948,20.,1.57850150671815));
#11589=CARTESIAN_POINT('Ctrl Pts',(-11.1141911417013,20.,1.31175534601927));
#11590=CARTESIAN_POINT('Ctrl Pts',(-11.1225356031101,20.,1.04484600136694));
#11591=CARTESIAN_POINT('Ctrl Pts',(-11.1214040387022,20.,0.778285111146802));
#11592=CARTESIAN_POINT('Ctrl Pts',(-11.1202704089922,20.,0.511237700885669));
#11593=CARTESIAN_POINT('Ctrl Pts',(-11.1096260686206,20.,0.244539372120431));
#11594=CARTESIAN_POINT('Ctrl Pts',(-11.0894661186789,20.,-0.0212930842774587));
#11595=CARTESIAN_POINT('Ctrl Pts',(-11.0694226014249,20.,-0.285590239869608));
#11596=CARTESIAN_POINT('Ctrl Pts',(-11.0399729544881,20.,-0.549032106527681));
#11597=CARTESIAN_POINT('Ctrl Pts',(-11.0010625248055,20.,-0.811099100292543));
#11598=CARTESIAN_POINT('Ctrl Pts',(-10.9627843225331,20.,-1.06890795714815));
#11599=CARTESIAN_POINT('Ctrl Pts',(-10.9153500990796,20.,-1.32538677858601));
#11600=CARTESIAN_POINT('Ctrl Pts',(-10.8586617973662,20.,-1.58002123097109));
#11601=CARTESIAN_POINT('Ctrl Pts',(-10.824283554091,20.,-1.73444259985593));
#11602=CARTESIAN_POINT('Ctrl Pts',(-10.786501025353,20.,-1.88818524282884));
#11603=CARTESIAN_POINT('Ctrl Pts',(-10.7452842897659,20.,-2.04112961510651));
#11604=CARTESIAN_POINT('Ctrl Pts',(-10.6983394263361,20.,-2.21532955031828));
#11605=CARTESIAN_POINT('Ctrl Pts',(-10.6469394936606,20.,-2.38849410088829));
#11606=CARTESIAN_POINT('Ctrl Pts',(-10.5911391151801,20.,-2.5604596881072));
#11607=CARTESIAN_POINT('Ctrl Pts',(-10.5808112700642,20.,-2.59228803763508));
#11608=CARTESIAN_POINT('Ctrl Pts',(-10.5703323195386,20.,-2.6240761705273));
#11609=CARTESIAN_POINT('Ctrl Pts',(-10.5597080024052,20.,-2.65580723494851));
#11610=CARTESIAN_POINT('Ctrl Pts',(-10.4761217376019,20.,-2.90544974089902));
#11611=CARTESIAN_POINT('Ctrl Pts',(-10.3834680471007,20.,-3.15179168198811));
#11612=CARTESIAN_POINT('Ctrl Pts',(-10.282020382983,20.,-3.39437485165473));
#11613=CARTESIAN_POINT('Ctrl Pts',(-10.1805768302556,20.,-3.63694819010331));
#11614=CARTESIAN_POINT('Ctrl Pts',(-10.0703396373221,20.,-3.87576361222901));
#11615=CARTESIAN_POINT('Ctrl Pts',(-9.95153837324811,20.,-4.1103350806491));
#11616=CARTESIAN_POINT('Ctrl Pts',(-9.83294619673873,20.,-4.34449370853715));
#11617=CARTESIAN_POINT('Ctrl Pts',(-9.70581969057772,20.,-4.5744238410096));
#11618=CARTESIAN_POINT('Ctrl Pts',(-9.57034919813197,20.,-4.79960611610117));
#11619=CARTESIAN_POINT('Ctrl Pts',(-9.54674783630744,20.,-4.83883686115094));
#11620=CARTESIAN_POINT('Ctrl Pts',(-9.52289211440892,20.,-4.8779250440819));
#11621=CARTESIAN_POINT('Ctrl Pts',(-9.49878620932176,20.,-4.91686250731363));
#11622=CARTESIAN_POINT('Ctrl Pts',(-9.4714725605423,20.,-4.96098133177716));
#11623=CARTESIAN_POINT('Ctrl Pts',(-9.44384412923328,20.,-5.00489629459305));
#11624=CARTESIAN_POINT('Ctrl Pts',(-9.41590688328757,20.,-5.0485974151017));
#11625=CARTESIAN_POINT('Ctrl Pts',(-9.27645734340157,20.,-5.26673277315658));
#11626=CARTESIAN_POINT('Ctrl Pts',(-9.12928197466736,20.,-5.47959889217826));
#11627=CARTESIAN_POINT('Ctrl Pts',(-8.97460595807497,20.,-5.68672989826698));
#11628=CARTESIAN_POINT('Ctrl Pts',(-8.82197249701016,20.,-5.89112566077535));
#11629=CARTESIAN_POINT('Ctrl Pts',(-8.66203475265525,20.,-6.08993719137158));
#11630=CARTESIAN_POINT('Ctrl Pts',(-8.49497511955485,20.,-6.28267973360122));
#11631=CARTESIAN_POINT('Ctrl Pts',(-8.37973300106364,20.,-6.41563859671912));
#11632=CARTESIAN_POINT('Ctrl Pts',(-8.2611011573261,20.,-6.54570870489164));
#11633=CARTESIAN_POINT('Ctrl Pts',(-8.13913138220323,20.,-6.6727188759329));
#11634=CARTESIAN_POINT('Ctrl Pts',(-8.07193084909504,20.,-6.74269646829574));
#11635=CARTESIAN_POINT('Ctrl Pts',(-8.0037169417772,20.,-6.81174500263592));
#11636=CARTESIAN_POINT('Ctrl Pts',(-7.93451184210526,20.,-6.87984615149801));
#11637=CARTESIAN_POINT('Origin',(0.,40.,-2.22044604925031E-15));
#11638=CARTESIAN_POINT('',(9.46171656752341,40.,16.3881738217667));
#11639=CARTESIAN_POINT('',(-9.46171656752339,40.,16.3881738217667));
#11640=CARTESIAN_POINT('',(9.46171656752341,40.,16.3881738217667));
#11641=CARTESIAN_POINT('',(18.9234331350468,40.,-1.22124532708767E-14));
#11642=CARTESIAN_POINT('',(18.9234331350468,40.,-1.22124532708767E-14));
#11643=CARTESIAN_POINT('',(9.46171656752339,40.,-16.3881738217667));
#11644=CARTESIAN_POINT('',(9.46171656752339,40.,-16.3881738217667));
#11645=CARTESIAN_POINT('',(-9.4617165675234,40.,-16.3881738217667));
#11646=CARTESIAN_POINT('',(-9.4617165675234,40.,-16.3881738217667));
#11647=CARTESIAN_POINT('',(-18.9234331350468,40.,4.44089209850063E-15));
#11648=CARTESIAN_POINT('',(-18.9234331350468,40.,4.44089209850063E-15));
#11649=CARTESIAN_POINT('',(-9.46171656752339,40.,16.3881738217667));
#11650=CARTESIAN_POINT('Origin',(18.9234331350468,20.,-1.22124532708767E-14));
#11651=CARTESIAN_POINT('',(18.9234331350468,20.,-1.22124532708767E-14));
#11652=CARTESIAN_POINT('',(9.46171656752341,20.,16.3881738217667));
#11653=CARTESIAN_POINT('',(18.9234331350468,20.,-1.22124532708767E-14));
#11654=CARTESIAN_POINT('',(18.9234331350468,20.,-1.22124532708767E-14));
#11655=CARTESIAN_POINT('',(9.46171656752341,20.,16.3881738217667));
#11656=CARTESIAN_POINT('Origin',(9.46171656752339,20.,-16.3881738217667));
#11657=CARTESIAN_POINT('',(9.46171656752339,20.,-16.3881738217667));
#11658=CARTESIAN_POINT('',(9.46171656752339,20.,-16.3881738217667));
#11659=CARTESIAN_POINT('',(9.46171656752339,20.,-16.3881738217667));
#11660=CARTESIAN_POINT('Origin',(-9.4617165675234,20.,-16.3881738217667));
#11661=CARTESIAN_POINT('',(-9.4617165675234,20.,-16.3881738217667));
#11662=CARTESIAN_POINT('',(-9.4617165675234,20.,-16.3881738217667));
#11663=CARTESIAN_POINT('',(-9.4617165675234,20.,-16.3881738217667));
#11664=CARTESIAN_POINT('Origin',(-18.9234331350468,20.,4.44089209850063E-15));
#11665=CARTESIAN_POINT('',(-18.9234331350468,20.,4.44089209850063E-15));
#11666=CARTESIAN_POINT('',(-18.9234331350468,20.,4.44089209850063E-15));
#11667=CARTESIAN_POINT('',(-18.9234331350468,20.,4.44089209850063E-15));
#11668=CARTESIAN_POINT('Origin',(-9.46171656752339,20.,16.3881738217667));
#11669=CARTESIAN_POINT('',(-9.46171656752339,20.,16.3881738217667));
#11670=CARTESIAN_POINT('',(-9.46171656752339,20.,16.3881738217667));
#11671=CARTESIAN_POINT('',(-9.46171656752339,20.,16.3881738217667));
#11672=CARTESIAN_POINT('Origin',(9.46171656752341,20.,16.3881738217667));
#11673=CARTESIAN_POINT('',(9.46171656752341,20.,16.3881738217667));
#11674=CARTESIAN_POINT('Origin',(0.,20.,-2.22044604925031E-15));
#42650=UNCERTAINTY_MEASURE_WITH_UNIT(LENGTH_MEASURE(0.01),#42668,
'DISTANCE_ACCURACY_VALUE',
'Maximum model space distance between geometric entities at asserted c
onnectivities');
#42656=UNCERTAINTY_MEASURE_WITH_UNIT(LENGTH_MEASURE(0.01),#42668,
'DISTANCE_ACCURACY_VALUE',
'Maximum model space distance between geometric entities at asserted c
onnectivities');
#42661=(
GEOMETRIC_REPRESENTATION_CONTEXT(3)
GLOBAL_UNCERTAINTY_ASSIGNED_CONTEXT((#42650))
GLOBAL_UNIT_ASSIGNED_CONTEXT((#42668,#42670,#42671))
REPRESENTATION_CONTEXT('','3D')
);
#42667=(
GEOMETRIC_REPRESENTATION_CONTEXT(3)
GLOBAL_UNCERTAINTY_ASSIGNED_CONTEXT((#42656))
GLOBAL_UNIT_ASSIGNED_CONTEXT((#42668,#42670,#42671))
REPRESENTATION_CONTEXT('','3D')
);
#42668=(
LENGTH_UNIT()
NAMED_UNIT(*)
SI_UNIT(.MILLI.,.METRE.)
);
#42670=(
NAMED_UNIT(*)
PLANE_ANGLE_UNIT()
SI_UNIT($,.RADIAN.)
);
#42671=(
NAMED_UNIT(*)
SI_UNIT($,.STERADIAN.)
SOLID_ANGLE_UNIT()
);
#42676=SHAPE_DEFINITION_REPRESENTATION(#42686,#42705);
#42686=PRODUCT_DEFINITION_SHAPE('',$,#42716);
#42705=SHAPE_REPRESENTATION('',(#4235),#42661);
#42711=PRODUCT_DEFINITION_CONTEXT('part definition',#42743,'design');
#42716=PRODUCT_DEFINITION('Adapter','Adapter',#42726,#42711);
#42726=PRODUCT_DEFINITION_FORMATION('',$,#42749);
#42743=APPLICATION_CONTEXT(
'Core Data for Automotive Mechanical Design Process');
#42744=PRODUCT_CONTEXT('part definition',#42743,'mechanical');
#42749=PRODUCT('Adapter','Adapter',$,(#42744));
#42756=PRESENTATION_STYLE_ASSIGNMENT((#42758));
#42758=SURFACE_STYLE_USAGE(.BOTH.,#42760);
#42760=SURFACE_SIDE_STYLE('',(#42762));
#42762=SURFACE_STYLE_FILL_AREA(#42764);
#42764=FILL_AREA_STYLE('Opaque(160,160,160)',(#42766));
#42766=FILL_AREA_STYLE_COLOUR('Opaque(160,160,160)',#42768);
#42768=COLOUR_RGB('Opaque(160,160,160)', 0.09019608, 0.27058824, 0.51372549);
ENDSEC;
END-ISO-10303-21;
